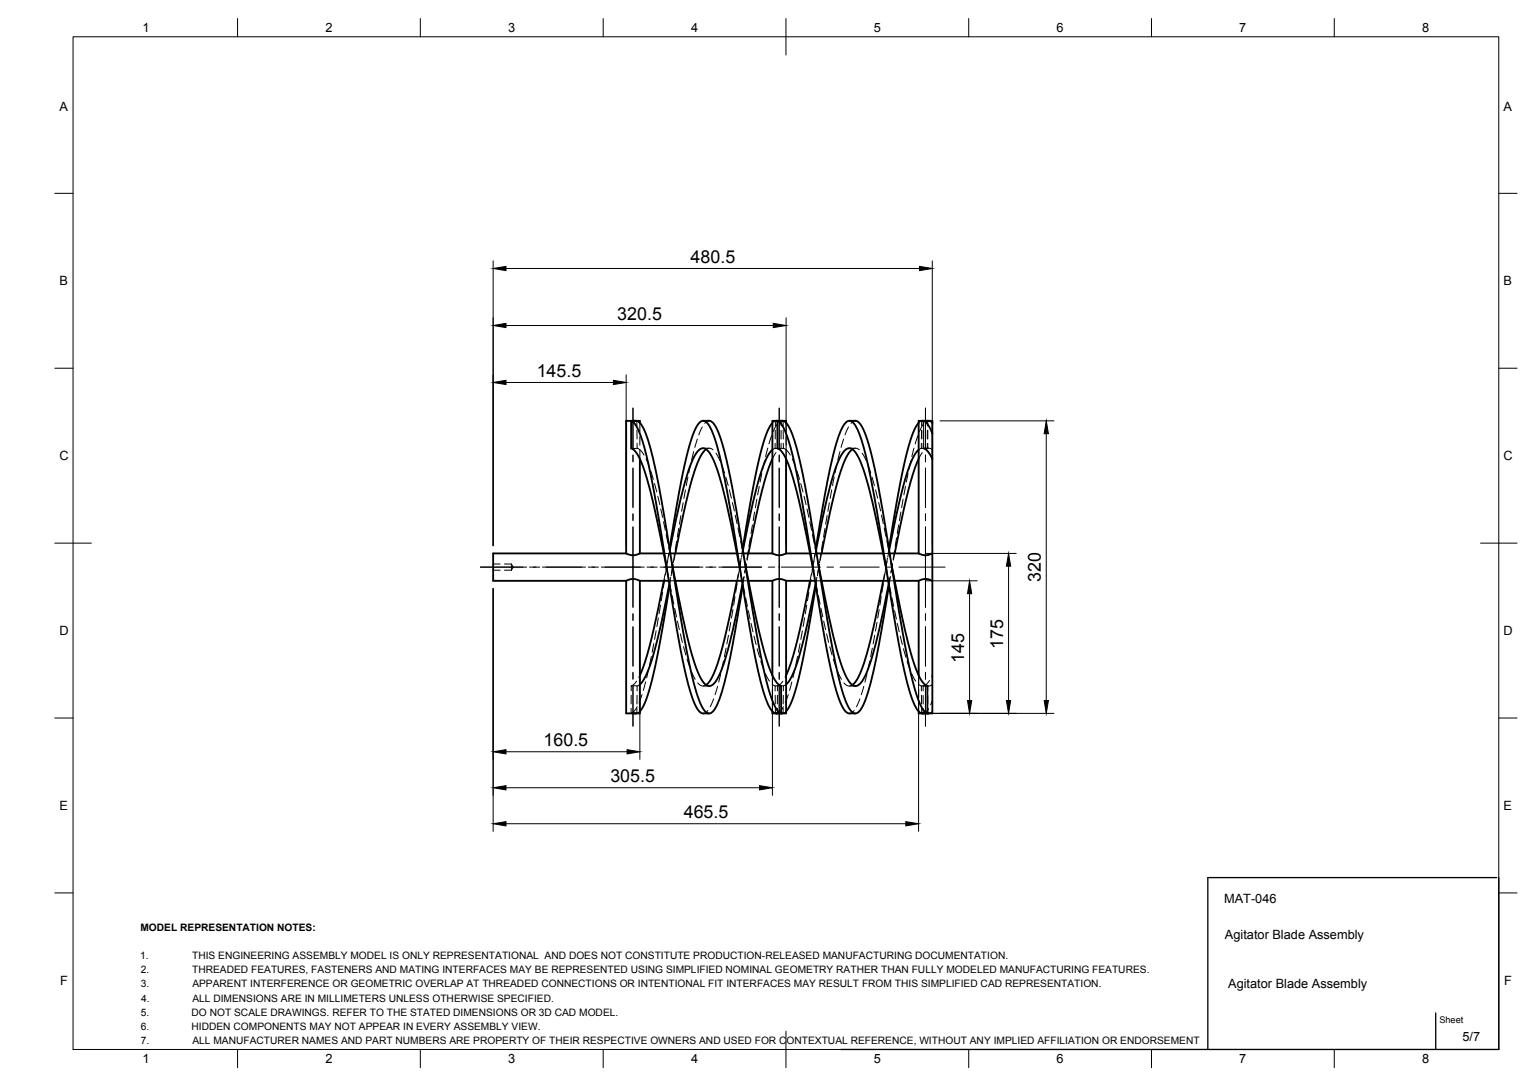
ISO-10303-21;
HEADER;
/* Generated by software containing ST-Developer
 * from STEP Tools, Inc. (www.steptools.com) 
 */

FILE_DESCRIPTION(
/* description */ ('STEP AP214'),
/* implementation_level */ '2;1');

FILE_NAME(
/* name */ 'Agitator Blade Assembly.step',
/* time_stamp */ '2026-11-14T22:16:48-08:00',
/* author */ (''),
/* organization */ (''),
/* preprocessor_version */ 'ST-DEVELOPER v20.2',
/* originating_system */ 'Autodesk Translation Framework v15.17.0.0',
/* authorisation */ '');

FILE_SCHEMA (('AUTOMOTIVE_DESIGN { 1 0 10303 214 3 1 1 }'));
ENDSEC;

DATA;
#10=MECHANICAL_DESIGN_GEOMETRIC_PRESENTATION_REPRESENTATION('',(#5496,#5497,#5498),#276462);
#335=CONICAL_SURFACE('',#110842,3.4,1.02974425867665);
#4017=(
BOUNDED_SURFACE()
B_SPLINE_SURFACE(1,2,((#265160,#265161,#265162,#265163,#265164,#265165,
#265166,#265167,#265168,#265169,#265170,#265171,#265172,#265173,#265174,
#265175,#265176,#265177,#265178,#265179,#265180,#265181,#265182,#265183,
#265184,#265185,#265186,#265187,#265188,#265189,#265190,#265191,#265192,
#265193,#265194,#265195,#265196,#265197,#265198,#265199,#265200,#265201,
#265202,#265203,#265204,#265205,#265206,#265207,#265208,#265209,#265210,
#265211,#265212,#265213,#265214,#265215,#265216,#265217,#265218,#265219,
#265220,#265221,#265222,#265223,#265224,#265225,#265226,#265227,#265228,
#265229,#265230,#265231,#265232,#265233,#265234,#265235,#265236,#265237,
#265238,#265239,#265240),(#265241,#265242,#265243,#265244,#265245,#265246,
#265247,#265248,#265249,#265250,#265251,#265252,#265253,#265254,#265255,
#265256,#265257,#265258,#265259,#265260,#265261,#265262,#265263,#265264,
#265265,#265266,#265267,#265268,#265269,#265270,#265271,#265272,#265273,
#265274,#265275,#265276,#265277,#265278,#265279,#265280,#265281,#265282,
#265283,#265284,#265285,#265286,#265287,#265288,#265289,#265290,#265291,
#265292,#265293,#265294,#265295,#265296,#265297,#265298,#265299,#265300,
#265301,#265302,#265303,#265304,#265305,#265306,#265307,#265308,#265309,
#265310,#265311,#265312,#265313,#265314,#265315,#265316,#265317,#265318,
#265319,#265320,#265321)),.UNSPECIFIED.,.F.,.F.,.F.)
B_SPLINE_SURFACE_WITH_KNOTS((2,2),(3,2,2,2,2,2,2,2,2,2,2,2,2,2,2,2,2,2,
2,2,2,2,2,2,2,2,2,2,2,2,2,2,2,2,2,2,2,2,2,2,3),(0.,1.),(0.,0.025,0.05,0.075,
0.1,0.125,0.15,0.175,0.2,0.225,0.25,0.275,0.3,0.325,0.35,0.375,0.4,0.425,
0.45,0.475,0.5,0.525,0.55,0.575,0.6,0.625,0.65,0.675,0.7,0.725,0.75,0.775,
0.8,0.825,0.85,0.875,0.9,0.925,0.95,0.975,1.),.UNSPECIFIED.)
GEOMETRIC_REPRESENTATION_ITEM()
RATIONAL_B_SPLINE_SURFACE(((1.,0.996917333733128,1.,0.996917333733128,1.,
0.996917333733128,1.,0.996917333733128,1.,0.996917333733128,1.,0.996917333733128,
1.,0.996917333733128,1.,0.996917333733128,1.,0.996917333733128,1.,0.996917333733128,
1.,0.996917333733128,1.,0.996917333733128,1.,0.996917333733128,1.,0.996917333733128,
1.,0.996917333733128,1.,0.996917333733128,1.,0.996917333733128,1.,0.996917333733128,
1.,0.996917333733128,1.,0.996917333733128,1.,0.996917333733128,1.,0.996917333733128,
1.,0.996917333733128,1.,0.996917333733128,1.,0.996917333733128,1.,0.996917333733128,
1.,0.996917333733128,1.,0.996917333733128,1.,0.996917333733128,1.,0.996917333733128,
1.,0.996917333733128,1.,0.996917333733128,1.,0.996917333733128,1.,0.996917333733128,
1.,0.996917333733128,1.,0.996917333733128,1.,0.996917333733128,1.,0.996917333733128,
1.,0.996917333733128,1.,0.996917333733128,1.),(1.,0.996917333733128,1.,
0.996917333733128,1.,0.996917333733128,1.,0.996917333733128,1.,0.996917333733128,
1.,0.996917333733128,1.,0.996917333733128,1.,0.996917333733128,1.,0.996917333733128,
1.,0.996917333733128,1.,0.996917333733128,1.,0.996917333733128,1.,0.996917333733128,
1.,0.996917333733128,1.,0.996917333733128,1.,0.996917333733128,1.,0.996917333733128,
1.,0.996917333733128,1.,0.996917333733128,1.,0.996917333733128,1.,0.996917333733128,
1.,0.996917333733128,1.,0.996917333733128,1.,0.996917333733128,1.,0.996917333733128,
1.,0.996917333733128,1.,0.996917333733128,1.,0.996917333733128,1.,0.996917333733128,
1.,0.996917333733128,1.,0.996917333733128,1.,0.996917333733128,1.,0.996917333733128,
1.,0.996917333733128,1.,0.996917333733128,1.,0.996917333733128,1.,0.996917333733128,
1.,0.996917333733128,1.,0.996917333733128,1.,0.996917333733128,1.)))
REPRESENTATION_ITEM('')
SURFACE()
);
#4018=(
BOUNDED_SURFACE()
B_SPLINE_SURFACE(1,2,((#265347,#265348,#265349,#265350,#265351,#265352,
#265353,#265354,#265355,#265356,#265357,#265358,#265359,#265360,#265361,
#265362,#265363,#265364,#265365,#265366,#265367,#265368,#265369,#265370,
#265371,#265372,#265373,#265374,#265375,#265376,#265377,#265378,#265379,
#265380,#265381,#265382,#265383,#265384,#265385,#265386,#265387,#265388,
#265389,#265390,#265391,#265392,#265393,#265394,#265395,#265396,#265397,
#265398,#265399,#265400,#265401,#265402,#265403,#265404,#265405,#265406,
#265407,#265408,#265409,#265410,#265411,#265412,#265413,#265414,#265415,
#265416,#265417,#265418,#265419,#265420,#265421,#265422,#265423,#265424,
#265425,#265426,#265427),(#265428,#265429,#265430,#265431,#265432,#265433,
#265434,#265435,#265436,#265437,#265438,#265439,#265440,#265441,#265442,
#265443,#265444,#265445,#265446,#265447,#265448,#265449,#265450,#265451,
#265452,#265453,#265454,#265455,#265456,#265457,#265458,#265459,#265460,
#265461,#265462,#265463,#265464,#265465,#265466,#265467,#265468,#265469,
#265470,#265471,#265472,#265473,#265474,#265475,#265476,#265477,#265478,
#265479,#265480,#265481,#265482,#265483,#265484,#265485,#265486,#265487,
#265488,#265489,#265490,#265491,#265492,#265493,#265494,#265495,#265496,
#265497,#265498,#265499,#265500,#265501,#265502,#265503,#265504,#265505,
#265506,#265507,#265508)),.UNSPECIFIED.,.F.,.F.,.F.)
B_SPLINE_SURFACE_WITH_KNOTS((2,2),(3,2,2,2,2,2,2,2,2,2,2,2,2,2,2,2,2,2,
2,2,2,2,2,2,2,2,2,2,2,2,2,2,2,2,2,2,2,2,2,2,3),(0.,1.),(0.,0.025,0.05,0.075,
0.1,0.125,0.15,0.175,0.2,0.225,0.25,0.275,0.3,0.325,0.35,0.375,0.4,0.425,
0.45,0.475,0.5,0.525,0.55,0.575,0.6,0.625,0.65,0.675,0.7,0.725,0.75,0.775,
0.8,0.825,0.85,0.875,0.9,0.925,0.95,0.975,1.),.UNSPECIFIED.)
GEOMETRIC_REPRESENTATION_ITEM()
RATIONAL_B_SPLINE_SURFACE(((1.,0.996917333733128,1.,0.996917333733128,1.,
0.996917333733128,1.,0.996917333733128,1.,0.996917333733128,1.,0.996917333733128,
1.,0.996917333733128,1.,0.996917333733128,1.,0.996917333733128,1.,0.996917333733128,
1.,0.996917333733128,1.,0.996917333733128,1.,0.996917333733128,1.,0.996917333733128,
1.,0.996917333733128,1.,0.996917333733128,1.,0.996917333733128,1.,0.996917333733128,
1.,0.996917333733128,1.,0.996917333733128,1.,0.996917333733128,1.,0.996917333733128,
1.,0.996917333733128,1.,0.996917333733128,1.,0.996917333733128,1.,0.996917333733128,
1.,0.996917333733128,1.,0.996917333733128,1.,0.996917333733128,1.,0.996917333733128,
1.,0.996917333733128,1.,0.996917333733128,1.,0.996917333733128,1.,0.996917333733128,
1.,0.996917333733128,1.,0.996917333733128,1.,0.996917333733128,1.,0.996917333733128,
1.,0.996917333733128,1.,0.996917333733128,1.),(1.,0.996917333733128,1.,
0.996917333733128,1.,0.996917333733128,1.,0.996917333733128,1.,0.996917333733128,
1.,0.996917333733128,1.,0.996917333733128,1.,0.996917333733128,1.,0.996917333733128,
1.,0.996917333733128,1.,0.996917333733128,1.,0.996917333733128,1.,0.996917333733128,
1.,0.996917333733128,1.,0.996917333733128,1.,0.996917333733128,1.,0.996917333733128,
1.,0.996917333733128,1.,0.996917333733128,1.,0.996917333733128,1.,0.996917333733128,
1.,0.996917333733128,1.,0.996917333733128,1.,0.996917333733128,1.,0.996917333733128,
1.,0.996917333733128,1.,0.996917333733128,1.,0.996917333733128,1.,0.996917333733128,
1.,0.996917333733128,1.,0.996917333733128,1.,0.996917333733128,1.,0.996917333733128,
1.,0.996917333733128,1.,0.996917333733128,1.,0.996917333733128,1.,0.996917333733128,
1.,0.996917333733128,1.,0.996917333733128,1.,0.996917333733128,1.)))
REPRESENTATION_ITEM('')
SURFACE()
);
#4019=(
BOUNDED_SURFACE()
B_SPLINE_SURFACE(1,2,((#265518,#265519,#265520,#265521,#265522,#265523,
#265524,#265525,#265526,#265527,#265528,#265529,#265530,#265531,#265532,
#265533,#265534,#265535,#265536,#265537,#265538,#265539,#265540,#265541,
#265542,#265543,#265544,#265545,#265546,#265547,#265548,#265549,#265550,
#265551,#265552,#265553,#265554,#265555,#265556,#265557,#265558,#265559,
#265560,#265561,#265562,#265563,#265564,#265565,#265566,#265567,#265568,
#265569,#265570,#265571,#265572,#265573,#265574,#265575,#265576,#265577,
#265578,#265579,#265580,#265581,#265582,#265583,#265584,#265585,#265586,
#265587,#265588,#265589,#265590,#265591,#265592,#265593,#265594,#265595,
#265596,#265597,#265598),(#265599,#265600,#265601,#265602,#265603,#265604,
#265605,#265606,#265607,#265608,#265609,#265610,#265611,#265612,#265613,
#265614,#265615,#265616,#265617,#265618,#265619,#265620,#265621,#265622,
#265623,#265624,#265625,#265626,#265627,#265628,#265629,#265630,#265631,
#265632,#265633,#265634,#265635,#265636,#265637,#265638,#265639,#265640,
#265641,#265642,#265643,#265644,#265645,#265646,#265647,#265648,#265649,
#265650,#265651,#265652,#265653,#265654,#265655,#265656,#265657,#265658,
#265659,#265660,#265661,#265662,#265663,#265664,#265665,#265666,#265667,
#265668,#265669,#265670,#265671,#265672,#265673,#265674,#265675,#265676,
#265677,#265678,#265679)),.UNSPECIFIED.,.F.,.F.,.F.)
B_SPLINE_SURFACE_WITH_KNOTS((2,2),(3,2,2,2,2,2,2,2,2,2,2,2,2,2,2,2,2,2,
2,2,2,2,2,2,2,2,2,2,2,2,2,2,2,2,2,2,2,2,2,2,3),(0.,1.),(0.,0.025,0.05,0.075,
0.1,0.125,0.15,0.175,0.2,0.225,0.25,0.275,0.3,0.325,0.35,0.375,0.4,0.425,
0.45,0.475,0.5,0.525,0.55,0.575,0.6,0.625,0.65,0.675,0.7,0.725,0.75,0.775,
0.8,0.825,0.85,0.875,0.9,0.925,0.95,0.975,1.),.UNSPECIFIED.)
GEOMETRIC_REPRESENTATION_ITEM()
RATIONAL_B_SPLINE_SURFACE(((1.,0.996917333733128,1.,0.996917333733128,1.,
0.996917333733128,1.,0.996917333733128,1.,0.996917333733128,1.,0.996917333733128,
1.,0.996917333733128,1.,0.996917333733128,1.,0.996917333733128,1.,0.996917333733128,
1.,0.996917333733128,1.,0.996917333733128,1.,0.996917333733128,1.,0.996917333733128,
1.,0.996917333733128,1.,0.996917333733128,1.,0.996917333733128,1.,0.996917333733128,
1.,0.996917333733128,1.,0.996917333733128,1.,0.996917333733128,1.,0.996917333733128,
1.,0.996917333733128,1.,0.996917333733128,1.,0.996917333733128,1.,0.996917333733128,
1.,0.996917333733128,1.,0.996917333733128,1.,0.996917333733128,1.,0.996917333733128,
1.,0.996917333733128,1.,0.996917333733128,1.,0.996917333733128,1.,0.996917333733128,
1.,0.996917333733128,1.,0.996917333733128,1.,0.996917333733128,1.,0.996917333733128,
1.,0.996917333733128,1.,0.996917333733128,1.),(1.,0.996917333733128,1.,
0.996917333733128,1.,0.996917333733128,1.,0.996917333733128,1.,0.996917333733128,
1.,0.996917333733128,1.,0.996917333733128,1.,0.996917333733128,1.,0.996917333733128,
1.,0.996917333733128,1.,0.996917333733128,1.,0.996917333733128,1.,0.996917333733128,
1.,0.996917333733128,1.,0.996917333733128,1.,0.996917333733128,1.,0.996917333733128,
1.,0.996917333733128,1.,0.996917333733128,1.,0.996917333733128,1.,0.996917333733128,
1.,0.996917333733128,1.,0.996917333733128,1.,0.996917333733128,1.,0.996917333733128,
1.,0.996917333733128,1.,0.996917333733128,1.,0.996917333733128,1.,0.996917333733128,
1.,0.996917333733128,1.,0.996917333733128,1.,0.996917333733128,1.,0.996917333733128,
1.,0.996917333733128,1.,0.996917333733128,1.,0.996917333733128,1.,0.996917333733128,
1.,0.996917333733128,1.,0.996917333733128,1.,0.996917333733128,1.)))
REPRESENTATION_ITEM('')
SURFACE()
);
#4020=(
BOUNDED_SURFACE()
B_SPLINE_SURFACE(1,2,((#265698,#265699,#265700,#265701,#265702,#265703,
#265704,#265705,#265706,#265707,#265708,#265709,#265710,#265711,#265712,
#265713,#265714,#265715,#265716,#265717,#265718,#265719,#265720,#265721,
#265722,#265723,#265724,#265725,#265726,#265727,#265728,#265729,#265730,
#265731,#265732,#265733,#265734,#265735,#265736,#265737,#265738,#265739,
#265740,#265741,#265742,#265743,#265744,#265745,#265746,#265747,#265748,
#265749,#265750,#265751,#265752,#265753,#265754,#265755,#265756,#265757,
#265758,#265759,#265760,#265761,#265762,#265763,#265764,#265765,#265766,
#265767,#265768,#265769,#265770,#265771,#265772,#265773,#265774,#265775,
#265776,#265777,#265778),(#265779,#265780,#265781,#265782,#265783,#265784,
#265785,#265786,#265787,#265788,#265789,#265790,#265791,#265792,#265793,
#265794,#265795,#265796,#265797,#265798,#265799,#265800,#265801,#265802,
#265803,#265804,#265805,#265806,#265807,#265808,#265809,#265810,#265811,
#265812,#265813,#265814,#265815,#265816,#265817,#265818,#265819,#265820,
#265821,#265822,#265823,#265824,#265825,#265826,#265827,#265828,#265829,
#265830,#265831,#265832,#265833,#265834,#265835,#265836,#265837,#265838,
#265839,#265840,#265841,#265842,#265843,#265844,#265845,#265846,#265847,
#265848,#265849,#265850,#265851,#265852,#265853,#265854,#265855,#265856,
#265857,#265858,#265859)),.UNSPECIFIED.,.F.,.F.,.F.)
B_SPLINE_SURFACE_WITH_KNOTS((2,2),(3,2,2,2,2,2,2,2,2,2,2,2,2,2,2,2,2,2,
2,2,2,2,2,2,2,2,2,2,2,2,2,2,2,2,2,2,2,2,2,2,3),(0.,1.),(0.,0.025,0.05,0.075,
0.1,0.125,0.15,0.175,0.2,0.225,0.25,0.275,0.3,0.325,0.35,0.375,0.4,0.425,
0.45,0.475,0.5,0.525,0.55,0.575,0.6,0.625,0.65,0.675,0.7,0.725,0.75,0.775,
0.8,0.825,0.85,0.875,0.9,0.925,0.95,0.975,1.),.UNSPECIFIED.)
GEOMETRIC_REPRESENTATION_ITEM()
RATIONAL_B_SPLINE_SURFACE(((1.,0.996917333733128,1.,0.996917333733128,1.,
0.996917333733128,1.,0.996917333733128,1.,0.996917333733128,1.,0.996917333733128,
1.,0.996917333733128,1.,0.996917333733128,1.,0.996917333733128,1.,0.996917333733128,
1.,0.996917333733128,1.,0.996917333733128,1.,0.996917333733128,1.,0.996917333733128,
1.,0.996917333733128,1.,0.996917333733128,1.,0.996917333733128,1.,0.996917333733128,
1.,0.996917333733128,1.,0.996917333733128,1.,0.996917333733128,1.,0.996917333733128,
1.,0.996917333733128,1.,0.996917333733128,1.,0.996917333733128,1.,0.996917333733128,
1.,0.996917333733128,1.,0.996917333733128,1.,0.996917333733128,1.,0.996917333733128,
1.,0.996917333733128,1.,0.996917333733128,1.,0.996917333733128,1.,0.996917333733128,
1.,0.996917333733128,1.,0.996917333733128,1.,0.996917333733128,1.,0.996917333733128,
1.,0.996917333733128,1.,0.996917333733128,1.),(1.,0.996917333733128,1.,
0.996917333733128,1.,0.996917333733128,1.,0.996917333733128,1.,0.996917333733128,
1.,0.996917333733128,1.,0.996917333733128,1.,0.996917333733128,1.,0.996917333733128,
1.,0.996917333733128,1.,0.996917333733128,1.,0.996917333733128,1.,0.996917333733128,
1.,0.996917333733128,1.,0.996917333733128,1.,0.996917333733128,1.,0.996917333733128,
1.,0.996917333733128,1.,0.996917333733128,1.,0.996917333733128,1.,0.996917333733128,
1.,0.996917333733128,1.,0.996917333733128,1.,0.996917333733128,1.,0.996917333733128,
1.,0.996917333733128,1.,0.996917333733128,1.,0.996917333733128,1.,0.996917333733128,
1.,0.996917333733128,1.,0.996917333733128,1.,0.996917333733128,1.,0.996917333733128,
1.,0.996917333733128,1.,0.996917333733128,1.,0.996917333733128,1.,0.996917333733128,
1.,0.996917333733128,1.,0.996917333733128,1.,0.996917333733128,1.)))
REPRESENTATION_ITEM('')
SURFACE()
);
#4021=(
BOUNDED_SURFACE()
B_SPLINE_SURFACE(1,2,((#265864,#265865,#265866,#265867,#265868,#265869,
#265870,#265871,#265872,#265873,#265874,#265875,#265876,#265877,#265878,
#265879,#265880,#265881,#265882,#265883,#265884,#265885,#265886,#265887,
#265888,#265889,#265890,#265891,#265892,#265893,#265894,#265895,#265896,
#265897,#265898,#265899,#265900,#265901,#265902,#265903,#265904,#265905,
#265906,#265907,#265908,#265909,#265910,#265911,#265912,#265913,#265914,
#265915,#265916,#265917,#265918,#265919,#265920,#265921,#265922,#265923,
#265924,#265925,#265926,#265927,#265928,#265929,#265930,#265931,#265932,
#265933,#265934,#265935,#265936,#265937,#265938,#265939,#265940,#265941,
#265942,#265943,#265944),(#265945,#265946,#265947,#265948,#265949,#265950,
#265951,#265952,#265953,#265954,#265955,#265956,#265957,#265958,#265959,
#265960,#265961,#265962,#265963,#265964,#265965,#265966,#265967,#265968,
#265969,#265970,#265971,#265972,#265973,#265974,#265975,#265976,#265977,
#265978,#265979,#265980,#265981,#265982,#265983,#265984,#265985,#265986,
#265987,#265988,#265989,#265990,#265991,#265992,#265993,#265994,#265995,
#265996,#265997,#265998,#265999,#266000,#266001,#266002,#266003,#266004,
#266005,#266006,#266007,#266008,#266009,#266010,#266011,#266012,#266013,
#266014,#266015,#266016,#266017,#266018,#266019,#266020,#266021,#266022,
#266023,#266024,#266025)),.UNSPECIFIED.,.F.,.F.,.F.)
B_SPLINE_SURFACE_WITH_KNOTS((2,2),(3,2,2,2,2,2,2,2,2,2,2,2,2,2,2,2,2,2,
2,2,2,2,2,2,2,2,2,2,2,2,2,2,2,2,2,2,2,2,2,2,3),(0.,1.),(0.,0.025,0.05,0.075,
0.1,0.125,0.15,0.175,0.2,0.225,0.25,0.275,0.3,0.325,0.35,0.375,0.4,0.425,
0.45,0.475,0.5,0.525,0.55,0.575,0.6,0.625,0.65,0.675,0.7,0.725,0.75,0.775,
0.8,0.825,0.85,0.875,0.9,0.925,0.95,0.975,1.),.UNSPECIFIED.)
GEOMETRIC_REPRESENTATION_ITEM()
RATIONAL_B_SPLINE_SURFACE(((1.,0.996917333733128,1.,0.996917333733128,1.,
0.996917333733128,1.,0.996917333733128,1.,0.996917333733128,1.,0.996917333733128,
1.,0.996917333733128,1.,0.996917333733128,1.,0.996917333733128,1.,0.996917333733128,
1.,0.996917333733128,1.,0.996917333733128,1.,0.996917333733128,1.,0.996917333733128,
1.,0.996917333733128,1.,0.996917333733128,1.,0.996917333733128,1.,0.996917333733128,
1.,0.996917333733128,1.,0.996917333733128,1.,0.996917333733128,1.,0.996917333733128,
1.,0.996917333733128,1.,0.996917333733128,1.,0.996917333733128,1.,0.996917333733128,
1.,0.996917333733128,1.,0.996917333733128,1.,0.996917333733128,1.,0.996917333733128,
1.,0.996917333733128,1.,0.996917333733128,1.,0.996917333733128,1.,0.996917333733128,
1.,0.996917333733128,1.,0.996917333733128,1.,0.996917333733128,1.,0.996917333733128,
1.,0.996917333733128,1.,0.996917333733128,1.),(1.,0.996917333733128,1.,
0.996917333733128,1.,0.996917333733128,1.,0.996917333733128,1.,0.996917333733128,
1.,0.996917333733128,1.,0.996917333733128,1.,0.996917333733128,1.,0.996917333733128,
1.,0.996917333733128,1.,0.996917333733128,1.,0.996917333733128,1.,0.996917333733128,
1.,0.996917333733128,1.,0.996917333733128,1.,0.996917333733128,1.,0.996917333733128,
1.,0.996917333733128,1.,0.996917333733128,1.,0.996917333733128,1.,0.996917333733128,
1.,0.996917333733128,1.,0.996917333733128,1.,0.996917333733128,1.,0.996917333733128,
1.,0.996917333733128,1.,0.996917333733128,1.,0.996917333733128,1.,0.996917333733128,
1.,0.996917333733128,1.,0.996917333733128,1.,0.996917333733128,1.,0.996917333733128,
1.,0.996917333733128,1.,0.996917333733128,1.,0.996917333733128,1.,0.996917333733128,
1.,0.996917333733128,1.,0.996917333733128,1.,0.996917333733128,1.)))
REPRESENTATION_ITEM('')
SURFACE()
);
#4022=(
BOUNDED_SURFACE()
B_SPLINE_SURFACE(1,2,((#266051,#266052,#266053,#266054,#266055,#266056,
#266057,#266058,#266059,#266060,#266061,#266062,#266063,#266064,#266065,
#266066,#266067,#266068,#266069,#266070,#266071,#266072,#266073,#266074,
#266075,#266076,#266077,#266078,#266079,#266080,#266081,#266082,#266083,
#266084,#266085,#266086,#266087,#266088,#266089,#266090,#266091,#266092,
#266093,#266094,#266095,#266096,#266097,#266098,#266099,#266100,#266101,
#266102,#266103,#266104,#266105,#266106,#266107,#266108,#266109,#266110,
#266111,#266112,#266113,#266114,#266115,#266116,#266117,#266118,#266119,
#266120,#266121,#266122,#266123,#266124,#266125,#266126,#266127,#266128,
#266129,#266130,#266131),(#266132,#266133,#266134,#266135,#266136,#266137,
#266138,#266139,#266140,#266141,#266142,#266143,#266144,#266145,#266146,
#266147,#266148,#266149,#266150,#266151,#266152,#266153,#266154,#266155,
#266156,#266157,#266158,#266159,#266160,#266161,#266162,#266163,#266164,
#266165,#266166,#266167,#266168,#266169,#266170,#266171,#266172,#266173,
#266174,#266175,#266176,#266177,#266178,#266179,#266180,#266181,#266182,
#266183,#266184,#266185,#266186,#266187,#266188,#266189,#266190,#266191,
#266192,#266193,#266194,#266195,#266196,#266197,#266198,#266199,#266200,
#266201,#266202,#266203,#266204,#266205,#266206,#266207,#266208,#266209,
#266210,#266211,#266212)),.UNSPECIFIED.,.F.,.F.,.F.)
B_SPLINE_SURFACE_WITH_KNOTS((2,2),(3,2,2,2,2,2,2,2,2,2,2,2,2,2,2,2,2,2,
2,2,2,2,2,2,2,2,2,2,2,2,2,2,2,2,2,2,2,2,2,2,3),(0.,1.),(0.,0.025,0.05,0.075,
0.1,0.125,0.15,0.175,0.2,0.225,0.25,0.275,0.3,0.325,0.35,0.375,0.4,0.425,
0.45,0.475,0.5,0.525,0.55,0.575,0.6,0.625,0.65,0.675,0.7,0.725,0.75,0.775,
0.8,0.825,0.85,0.875,0.9,0.925,0.95,0.975,1.),.UNSPECIFIED.)
GEOMETRIC_REPRESENTATION_ITEM()
RATIONAL_B_SPLINE_SURFACE(((1.,0.996917333733128,1.,0.996917333733128,1.,
0.996917333733128,1.,0.996917333733128,1.,0.996917333733128,1.,0.996917333733128,
1.,0.996917333733128,1.,0.996917333733128,1.,0.996917333733128,1.,0.996917333733128,
1.,0.996917333733128,1.,0.996917333733128,1.,0.996917333733128,1.,0.996917333733128,
1.,0.996917333733128,1.,0.996917333733128,1.,0.996917333733128,1.,0.996917333733128,
1.,0.996917333733128,1.,0.996917333733128,1.,0.996917333733128,1.,0.996917333733128,
1.,0.996917333733128,1.,0.996917333733128,1.,0.996917333733128,1.,0.996917333733128,
1.,0.996917333733128,1.,0.996917333733128,1.,0.996917333733128,1.,0.996917333733128,
1.,0.996917333733128,1.,0.996917333733128,1.,0.996917333733128,1.,0.996917333733128,
1.,0.996917333733128,1.,0.996917333733128,1.,0.996917333733128,1.,0.996917333733128,
1.,0.996917333733128,1.,0.996917333733128,1.),(1.,0.996917333733128,1.,
0.996917333733128,1.,0.996917333733128,1.,0.996917333733128,1.,0.996917333733128,
1.,0.996917333733128,1.,0.996917333733128,1.,0.996917333733128,1.,0.996917333733128,
1.,0.996917333733128,1.,0.996917333733128,1.,0.996917333733128,1.,0.996917333733128,
1.,0.996917333733128,1.,0.996917333733128,1.,0.996917333733128,1.,0.996917333733128,
1.,0.996917333733128,1.,0.996917333733128,1.,0.996917333733128,1.,0.996917333733128,
1.,0.996917333733128,1.,0.996917333733128,1.,0.996917333733128,1.,0.996917333733128,
1.,0.996917333733128,1.,0.996917333733128,1.,0.996917333733128,1.,0.996917333733128,
1.,0.996917333733128,1.,0.996917333733128,1.,0.996917333733128,1.,0.996917333733128,
1.,0.996917333733128,1.,0.996917333733128,1.,0.996917333733128,1.,0.996917333733128,
1.,0.996917333733128,1.,0.996917333733128,1.,0.996917333733128,1.)))
REPRESENTATION_ITEM('')
SURFACE()
);
#4023=(
BOUNDED_SURFACE()
B_SPLINE_SURFACE(1,2,((#266224,#266225,#266226,#266227,#266228,#266229,
#266230,#266231,#266232,#266233,#266234,#266235,#266236,#266237,#266238,
#266239,#266240,#266241,#266242,#266243,#266244,#266245,#266246,#266247,
#266248,#266249,#266250,#266251,#266252,#266253,#266254,#266255,#266256,
#266257,#266258,#266259,#266260,#266261,#266262,#266263,#266264,#266265,
#266266,#266267,#266268,#266269,#266270,#266271,#266272,#266273,#266274,
#266275,#266276,#266277,#266278,#266279,#266280,#266281,#266282,#266283,
#266284,#266285,#266286,#266287,#266288,#266289,#266290,#266291,#266292,
#266293,#266294,#266295,#266296,#266297,#266298,#266299,#266300,#266301,
#266302,#266303,#266304),(#266305,#266306,#266307,#266308,#266309,#266310,
#266311,#266312,#266313,#266314,#266315,#266316,#266317,#266318,#266319,
#266320,#266321,#266322,#266323,#266324,#266325,#266326,#266327,#266328,
#266329,#266330,#266331,#266332,#266333,#266334,#266335,#266336,#266337,
#266338,#266339,#266340,#266341,#266342,#266343,#266344,#266345,#266346,
#266347,#266348,#266349,#266350,#266351,#266352,#266353,#266354,#266355,
#266356,#266357,#266358,#266359,#266360,#266361,#266362,#266363,#266364,
#266365,#266366,#266367,#266368,#266369,#266370,#266371,#266372,#266373,
#266374,#266375,#266376,#266377,#266378,#266379,#266380,#266381,#266382,
#266383,#266384,#266385)),.UNSPECIFIED.,.F.,.F.,.F.)
B_SPLINE_SURFACE_WITH_KNOTS((2,2),(3,2,2,2,2,2,2,2,2,2,2,2,2,2,2,2,2,2,
2,2,2,2,2,2,2,2,2,2,2,2,2,2,2,2,2,2,2,2,2,2,3),(0.,1.),(0.,0.025,0.05,0.075,
0.1,0.125,0.15,0.175,0.2,0.225,0.25,0.275,0.3,0.325,0.35,0.375,0.4,0.425,
0.45,0.475,0.5,0.525,0.55,0.575,0.6,0.625,0.65,0.675,0.7,0.725,0.75,0.775,
0.8,0.825,0.85,0.875,0.9,0.925,0.95,0.975,1.),.UNSPECIFIED.)
GEOMETRIC_REPRESENTATION_ITEM()
RATIONAL_B_SPLINE_SURFACE(((1.,0.996917333733128,1.,0.996917333733128,1.,
0.996917333733128,1.,0.996917333733128,1.,0.996917333733128,1.,0.996917333733128,
1.,0.996917333733128,1.,0.996917333733128,1.,0.996917333733128,1.,0.996917333733128,
1.,0.996917333733128,1.,0.996917333733128,1.,0.996917333733128,1.,0.996917333733128,
1.,0.996917333733128,1.,0.996917333733128,1.,0.996917333733128,1.,0.996917333733128,
1.,0.996917333733128,1.,0.996917333733128,1.,0.996917333733128,1.,0.996917333733128,
1.,0.996917333733128,1.,0.996917333733128,1.,0.996917333733128,1.,0.996917333733128,
1.,0.996917333733128,1.,0.996917333733128,1.,0.996917333733128,1.,0.996917333733128,
1.,0.996917333733128,1.,0.996917333733128,1.,0.996917333733128,1.,0.996917333733128,
1.,0.996917333733128,1.,0.996917333733128,1.,0.996917333733128,1.,0.996917333733128,
1.,0.996917333733128,1.,0.996917333733128,1.),(1.,0.996917333733128,1.,
0.996917333733128,1.,0.996917333733128,1.,0.996917333733128,1.,0.996917333733128,
1.,0.996917333733128,1.,0.996917333733128,1.,0.996917333733128,1.,0.996917333733128,
1.,0.996917333733128,1.,0.996917333733128,1.,0.996917333733128,1.,0.996917333733128,
1.,0.996917333733128,1.,0.996917333733128,1.,0.996917333733128,1.,0.996917333733128,
1.,0.996917333733128,1.,0.996917333733128,1.,0.996917333733128,1.,0.996917333733128,
1.,0.996917333733128,1.,0.996917333733128,1.,0.996917333733128,1.,0.996917333733128,
1.,0.996917333733128,1.,0.996917333733128,1.,0.996917333733128,1.,0.996917333733128,
1.,0.996917333733128,1.,0.996917333733128,1.,0.996917333733128,1.,0.996917333733128,
1.,0.996917333733128,1.,0.996917333733128,1.,0.996917333733128,1.,0.996917333733128,
1.,0.996917333733128,1.,0.996917333733128,1.,0.996917333733128,1.)))
REPRESENTATION_ITEM('')
SURFACE()
);
#4024=(
BOUNDED_SURFACE()
B_SPLINE_SURFACE(1,2,((#266402,#266403,#266404,#266405,#266406,#266407,
#266408,#266409,#266410,#266411,#266412,#266413,#266414,#266415,#266416,
#266417,#266418,#266419,#266420,#266421,#266422,#266423,#266424,#266425,
#266426,#266427,#266428,#266429,#266430,#266431,#266432,#266433,#266434,
#266435,#266436,#266437,#266438,#266439,#266440,#266441,#266442,#266443,
#266444,#266445,#266446,#266447,#266448,#266449,#266450,#266451,#266452,
#266453,#266454,#266455,#266456,#266457,#266458,#266459,#266460,#266461,
#266462,#266463,#266464,#266465,#266466,#266467,#266468,#266469,#266470,
#266471,#266472,#266473,#266474,#266475,#266476,#266477,#266478,#266479,
#266480,#266481,#266482),(#266483,#266484,#266485,#266486,#266487,#266488,
#266489,#266490,#266491,#266492,#266493,#266494,#266495,#266496,#266497,
#266498,#266499,#266500,#266501,#266502,#266503,#266504,#266505,#266506,
#266507,#266508,#266509,#266510,#266511,#266512,#266513,#266514,#266515,
#266516,#266517,#266518,#266519,#266520,#266521,#266522,#266523,#266524,
#266525,#266526,#266527,#266528,#266529,#266530,#266531,#266532,#266533,
#266534,#266535,#266536,#266537,#266538,#266539,#266540,#266541,#266542,
#266543,#266544,#266545,#266546,#266547,#266548,#266549,#266550,#266551,
#266552,#266553,#266554,#266555,#266556,#266557,#266558,#266559,#266560,
#266561,#266562,#266563)),.UNSPECIFIED.,.F.,.F.,.F.)
B_SPLINE_SURFACE_WITH_KNOTS((2,2),(3,2,2,2,2,2,2,2,2,2,2,2,2,2,2,2,2,2,
2,2,2,2,2,2,2,2,2,2,2,2,2,2,2,2,2,2,2,2,2,2,3),(0.,1.),(0.,0.025,0.05,0.075,
0.1,0.125,0.15,0.175,0.2,0.225,0.25,0.275,0.3,0.325,0.35,0.375,0.4,0.425,
0.45,0.475,0.5,0.525,0.55,0.575,0.6,0.625,0.65,0.675,0.7,0.725,0.75,0.775,
0.8,0.825,0.85,0.875,0.9,0.925,0.95,0.975,1.),.UNSPECIFIED.)
GEOMETRIC_REPRESENTATION_ITEM()
RATIONAL_B_SPLINE_SURFACE(((1.,0.996917333733128,1.,0.996917333733128,1.,
0.996917333733128,1.,0.996917333733128,1.,0.996917333733128,1.,0.996917333733128,
1.,0.996917333733128,1.,0.996917333733128,1.,0.996917333733128,1.,0.996917333733128,
1.,0.996917333733128,1.,0.996917333733128,1.,0.996917333733128,1.,0.996917333733128,
1.,0.996917333733128,1.,0.996917333733128,1.,0.996917333733128,1.,0.996917333733128,
1.,0.996917333733128,1.,0.996917333733128,1.,0.996917333733128,1.,0.996917333733128,
1.,0.996917333733128,1.,0.996917333733128,1.,0.996917333733128,1.,0.996917333733128,
1.,0.996917333733128,1.,0.996917333733128,1.,0.996917333733128,1.,0.996917333733128,
1.,0.996917333733128,1.,0.996917333733128,1.,0.996917333733128,1.,0.996917333733128,
1.,0.996917333733128,1.,0.996917333733128,1.,0.996917333733128,1.,0.996917333733128,
1.,0.996917333733128,1.,0.996917333733128,1.),(1.,0.996917333733128,1.,
0.996917333733128,1.,0.996917333733128,1.,0.996917333733128,1.,0.996917333733128,
1.,0.996917333733128,1.,0.996917333733128,1.,0.996917333733128,1.,0.996917333733128,
1.,0.996917333733128,1.,0.996917333733128,1.,0.996917333733128,1.,0.996917333733128,
1.,0.996917333733128,1.,0.996917333733128,1.,0.996917333733128,1.,0.996917333733128,
1.,0.996917333733128,1.,0.996917333733128,1.,0.996917333733128,1.,0.996917333733128,
1.,0.996917333733128,1.,0.996917333733128,1.,0.996917333733128,1.,0.996917333733128,
1.,0.996917333733128,1.,0.996917333733128,1.,0.996917333733128,1.,0.996917333733128,
1.,0.996917333733128,1.,0.996917333733128,1.,0.996917333733128,1.,0.996917333733128,
1.,0.996917333733128,1.,0.996917333733128,1.,0.996917333733128,1.,0.996917333733128,
1.,0.996917333733128,1.,0.996917333733128,1.,0.996917333733128,1.)))
REPRESENTATION_ITEM('')
SURFACE()
);
#4025=(
BOUNDED_SURFACE()
B_SPLINE_SURFACE(1,2,((#267127,#267128,#267129,#267130,#267131,#267132,
#267133,#267134,#267135,#267136,#267137,#267138,#267139,#267140,#267141,
#267142,#267143,#267144,#267145,#267146,#267147,#267148,#267149,#267150,
#267151,#267152,#267153,#267154,#267155,#267156,#267157,#267158,#267159,
#267160,#267161,#267162,#267163,#267164,#267165,#267166,#267167,#267168,
#267169,#267170,#267171,#267172,#267173,#267174,#267175,#267176,#267177,
#267178,#267179,#267180,#267181,#267182,#267183,#267184,#267185,#267186,
#267187,#267188,#267189,#267190,#267191,#267192,#267193,#267194,#267195,
#267196,#267197,#267198,#267199,#267200,#267201,#267202,#267203,#267204,
#267205,#267206,#267207),(#267208,#267209,#267210,#267211,#267212,#267213,
#267214,#267215,#267216,#267217,#267218,#267219,#267220,#267221,#267222,
#267223,#267224,#267225,#267226,#267227,#267228,#267229,#267230,#267231,
#267232,#267233,#267234,#267235,#267236,#267237,#267238,#267239,#267240,
#267241,#267242,#267243,#267244,#267245,#267246,#267247,#267248,#267249,
#267250,#267251,#267252,#267253,#267254,#267255,#267256,#267257,#267258,
#267259,#267260,#267261,#267262,#267263,#267264,#267265,#267266,#267267,
#267268,#267269,#267270,#267271,#267272,#267273,#267274,#267275,#267276,
#267277,#267278,#267279,#267280,#267281,#267282,#267283,#267284,#267285,
#267286,#267287,#267288)),.UNSPECIFIED.,.F.,.F.,.F.)
B_SPLINE_SURFACE_WITH_KNOTS((2,2),(3,2,2,2,2,2,2,2,2,2,2,2,2,2,2,2,2,2,
2,2,2,2,2,2,2,2,2,2,2,2,2,2,2,2,2,2,2,2,2,2,3),(0.,1.),(0.,0.025,0.05,0.075,
0.1,0.125,0.15,0.175,0.2,0.225,0.25,0.275,0.3,0.325,0.35,0.375,0.4,0.425,
0.45,0.475,0.5,0.525,0.55,0.575,0.6,0.625,0.65,0.675,0.7,0.725,0.75,0.775,
0.8,0.825,0.85,0.875,0.9,0.925,0.95,0.975,1.),.UNSPECIFIED.)
GEOMETRIC_REPRESENTATION_ITEM()
RATIONAL_B_SPLINE_SURFACE(((1.,0.996917333733128,1.,0.996917333733128,1.,
0.996917333733128,1.,0.996917333733128,1.,0.996917333733128,1.,0.996917333733128,
1.,0.996917333733128,1.,0.996917333733128,1.,0.996917333733128,1.,0.996917333733128,
1.,0.996917333733128,1.,0.996917333733128,1.,0.996917333733128,1.,0.996917333733128,
1.,0.996917333733128,1.,0.996917333733128,1.,0.996917333733128,1.,0.996917333733128,
1.,0.996917333733128,1.,0.996917333733128,1.,0.996917333733128,1.,0.996917333733128,
1.,0.996917333733128,1.,0.996917333733128,1.,0.996917333733128,1.,0.996917333733128,
1.,0.996917333733128,1.,0.996917333733128,1.,0.996917333733128,1.,0.996917333733128,
1.,0.996917333733128,1.,0.996917333733128,1.,0.996917333733128,1.,0.996917333733128,
1.,0.996917333733128,1.,0.996917333733128,1.,0.996917333733128,1.,0.996917333733128,
1.,0.996917333733128,1.,0.996917333733128,1.),(1.,0.996917333733128,1.,
0.996917333733128,1.,0.996917333733128,1.,0.996917333733128,1.,0.996917333733128,
1.,0.996917333733128,1.,0.996917333733128,1.,0.996917333733128,1.,0.996917333733128,
1.,0.996917333733128,1.,0.996917333733128,1.,0.996917333733128,1.,0.996917333733128,
1.,0.996917333733128,1.,0.996917333733128,1.,0.996917333733128,1.,0.996917333733128,
1.,0.996917333733128,1.,0.996917333733128,1.,0.996917333733128,1.,0.996917333733128,
1.,0.996917333733128,1.,0.996917333733128,1.,0.996917333733128,1.,0.996917333733128,
1.,0.996917333733128,1.,0.996917333733128,1.,0.996917333733128,1.,0.996917333733128,
1.,0.996917333733128,1.,0.996917333733128,1.,0.996917333733128,1.,0.996917333733128,
1.,0.996917333733128,1.,0.996917333733128,1.,0.996917333733128,1.,0.996917333733128,
1.,0.996917333733128,1.,0.996917333733128,1.,0.996917333733128,1.)))
REPRESENTATION_ITEM('')
SURFACE()
);
#4026=(
BOUNDED_SURFACE()
B_SPLINE_SURFACE(1,2,((#267451,#267452,#267453,#267454,#267455,#267456,
#267457,#267458,#267459,#267460,#267461,#267462,#267463,#267464,#267465,
#267466,#267467,#267468,#267469,#267470,#267471,#267472,#267473,#267474,
#267475,#267476,#267477,#267478,#267479,#267480,#267481,#267482,#267483,
#267484,#267485,#267486,#267487,#267488,#267489,#267490,#267491,#267492,
#267493,#267494,#267495,#267496,#267497,#267498,#267499,#267500,#267501,
#267502,#267503,#267504,#267505,#267506,#267507,#267508,#267509,#267510,
#267511,#267512,#267513,#267514,#267515,#267516,#267517,#267518,#267519,
#267520,#267521,#267522,#267523,#267524,#267525,#267526,#267527,#267528,
#267529,#267530,#267531),(#267532,#267533,#267534,#267535,#267536,#267537,
#267538,#267539,#267540,#267541,#267542,#267543,#267544,#267545,#267546,
#267547,#267548,#267549,#267550,#267551,#267552,#267553,#267554,#267555,
#267556,#267557,#267558,#267559,#267560,#267561,#267562,#267563,#267564,
#267565,#267566,#267567,#267568,#267569,#267570,#267571,#267572,#267573,
#267574,#267575,#267576,#267577,#267578,#267579,#267580,#267581,#267582,
#267583,#267584,#267585,#267586,#267587,#267588,#267589,#267590,#267591,
#267592,#267593,#267594,#267595,#267596,#267597,#267598,#267599,#267600,
#267601,#267602,#267603,#267604,#267605,#267606,#267607,#267608,#267609,
#267610,#267611,#267612)),.UNSPECIFIED.,.F.,.F.,.F.)
B_SPLINE_SURFACE_WITH_KNOTS((2,2),(3,2,2,2,2,2,2,2,2,2,2,2,2,2,2,2,2,2,
2,2,2,2,2,2,2,2,2,2,2,2,2,2,2,2,2,2,2,2,2,2,3),(0.,1.),(0.,0.025,0.05,0.075,
0.1,0.125,0.15,0.175,0.2,0.225,0.25,0.275,0.3,0.325,0.35,0.375,0.4,0.425,
0.45,0.475,0.5,0.525,0.55,0.575,0.6,0.625,0.65,0.675,0.7,0.725,0.75,0.775,
0.8,0.825,0.85,0.875,0.9,0.925,0.95,0.975,1.),.UNSPECIFIED.)
GEOMETRIC_REPRESENTATION_ITEM()
RATIONAL_B_SPLINE_SURFACE(((1.,0.996917333733128,1.,0.996917333733128,1.,
0.996917333733128,1.,0.996917333733128,1.,0.996917333733128,1.,0.996917333733128,
1.,0.996917333733128,1.,0.996917333733128,1.,0.996917333733128,1.,0.996917333733128,
1.,0.996917333733128,1.,0.996917333733128,1.,0.996917333733128,1.,0.996917333733128,
1.,0.996917333733128,1.,0.996917333733128,1.,0.996917333733128,1.,0.996917333733128,
1.,0.996917333733128,1.,0.996917333733128,1.,0.996917333733128,1.,0.996917333733128,
1.,0.996917333733128,1.,0.996917333733128,1.,0.996917333733128,1.,0.996917333733128,
1.,0.996917333733128,1.,0.996917333733128,1.,0.996917333733128,1.,0.996917333733128,
1.,0.996917333733128,1.,0.996917333733128,1.,0.996917333733128,1.,0.996917333733128,
1.,0.996917333733128,1.,0.996917333733128,1.,0.996917333733128,1.,0.996917333733128,
1.,0.996917333733128,1.,0.996917333733128,1.),(1.,0.996917333733128,1.,
0.996917333733128,1.,0.996917333733128,1.,0.996917333733128,1.,0.996917333733128,
1.,0.996917333733128,1.,0.996917333733128,1.,0.996917333733128,1.,0.996917333733128,
1.,0.996917333733128,1.,0.996917333733128,1.,0.996917333733128,1.,0.996917333733128,
1.,0.996917333733128,1.,0.996917333733128,1.,0.996917333733128,1.,0.996917333733128,
1.,0.996917333733128,1.,0.996917333733128,1.,0.996917333733128,1.,0.996917333733128,
1.,0.996917333733128,1.,0.996917333733128,1.,0.996917333733128,1.,0.996917333733128,
1.,0.996917333733128,1.,0.996917333733128,1.,0.996917333733128,1.,0.996917333733128,
1.,0.996917333733128,1.,0.996917333733128,1.,0.996917333733128,1.,0.996917333733128,
1.,0.996917333733128,1.,0.996917333733128,1.,0.996917333733128,1.,0.996917333733128,
1.,0.996917333733128,1.,0.996917333733128,1.,0.996917333733128,1.)))
REPRESENTATION_ITEM('')
SURFACE()
);
#4027=(
BOUNDED_SURFACE()
B_SPLINE_SURFACE(1,2,((#267694,#267695,#267696,#267697,#267698,#267699,
#267700,#267701,#267702,#267703,#267704,#267705,#267706,#267707,#267708,
#267709,#267710,#267711,#267712,#267713,#267714,#267715,#267716,#267717,
#267718,#267719,#267720,#267721,#267722,#267723,#267724,#267725,#267726,
#267727,#267728,#267729,#267730,#267731,#267732,#267733,#267734,#267735,
#267736,#267737,#267738,#267739,#267740,#267741,#267742,#267743,#267744,
#267745,#267746,#267747,#267748,#267749,#267750,#267751,#267752,#267753,
#267754,#267755,#267756,#267757,#267758,#267759,#267760,#267761,#267762,
#267763,#267764,#267765,#267766,#267767,#267768,#267769,#267770,#267771,
#267772,#267773,#267774),(#267775,#267776,#267777,#267778,#267779,#267780,
#267781,#267782,#267783,#267784,#267785,#267786,#267787,#267788,#267789,
#267790,#267791,#267792,#267793,#267794,#267795,#267796,#267797,#267798,
#267799,#267800,#267801,#267802,#267803,#267804,#267805,#267806,#267807,
#267808,#267809,#267810,#267811,#267812,#267813,#267814,#267815,#267816,
#267817,#267818,#267819,#267820,#267821,#267822,#267823,#267824,#267825,
#267826,#267827,#267828,#267829,#267830,#267831,#267832,#267833,#267834,
#267835,#267836,#267837,#267838,#267839,#267840,#267841,#267842,#267843,
#267844,#267845,#267846,#267847,#267848,#267849,#267850,#267851,#267852,
#267853,#267854,#267855)),.UNSPECIFIED.,.F.,.F.,.F.)
B_SPLINE_SURFACE_WITH_KNOTS((2,2),(3,2,2,2,2,2,2,2,2,2,2,2,2,2,2,2,2,2,
2,2,2,2,2,2,2,2,2,2,2,2,2,2,2,2,2,2,2,2,2,2,3),(0.,1.),(0.,0.025,0.05,0.075,
0.1,0.125,0.15,0.175,0.2,0.225,0.25,0.275,0.3,0.325,0.35,0.375,0.4,0.425,
0.45,0.475,0.5,0.525,0.55,0.575,0.6,0.625,0.65,0.675,0.7,0.725,0.75,0.775,
0.8,0.825,0.85,0.875,0.9,0.925,0.95,0.975,1.),.UNSPECIFIED.)
GEOMETRIC_REPRESENTATION_ITEM()
RATIONAL_B_SPLINE_SURFACE(((1.,0.996917333733128,1.,0.996917333733128,1.,
0.996917333733128,1.,0.996917333733128,1.,0.996917333733128,1.,0.996917333733128,
1.,0.996917333733128,1.,0.996917333733128,1.,0.996917333733128,1.,0.996917333733128,
1.,0.996917333733128,1.,0.996917333733128,1.,0.996917333733128,1.,0.996917333733128,
1.,0.996917333733128,1.,0.996917333733128,1.,0.996917333733128,1.,0.996917333733128,
1.,0.996917333733128,1.,0.996917333733128,1.,0.996917333733128,1.,0.996917333733128,
1.,0.996917333733128,1.,0.996917333733128,1.,0.996917333733128,1.,0.996917333733128,
1.,0.996917333733128,1.,0.996917333733128,1.,0.996917333733128,1.,0.996917333733128,
1.,0.996917333733128,1.,0.996917333733128,1.,0.996917333733128,1.,0.996917333733128,
1.,0.996917333733128,1.,0.996917333733128,1.,0.996917333733128,1.,0.996917333733128,
1.,0.996917333733128,1.,0.996917333733128,1.),(1.,0.996917333733128,1.,
0.996917333733128,1.,0.996917333733128,1.,0.996917333733128,1.,0.996917333733128,
1.,0.996917333733128,1.,0.996917333733128,1.,0.996917333733128,1.,0.996917333733128,
1.,0.996917333733128,1.,0.996917333733128,1.,0.996917333733128,1.,0.996917333733128,
1.,0.996917333733128,1.,0.996917333733128,1.,0.996917333733128,1.,0.996917333733128,
1.,0.996917333733128,1.,0.996917333733128,1.,0.996917333733128,1.,0.996917333733128,
1.,0.996917333733128,1.,0.996917333733128,1.,0.996917333733128,1.,0.996917333733128,
1.,0.996917333733128,1.,0.996917333733128,1.,0.996917333733128,1.,0.996917333733128,
1.,0.996917333733128,1.,0.996917333733128,1.,0.996917333733128,1.,0.996917333733128,
1.,0.996917333733128,1.,0.996917333733128,1.,0.996917333733128,1.,0.996917333733128,
1.,0.996917333733128,1.,0.996917333733128,1.,0.996917333733128,1.)))
REPRESENTATION_ITEM('')
SURFACE()
);
#4028=(
BOUNDED_SURFACE()
B_SPLINE_SURFACE(1,2,((#267937,#267938,#267939,#267940,#267941,#267942,
#267943,#267944,#267945,#267946,#267947,#267948,#267949,#267950,#267951,
#267952,#267953,#267954,#267955,#267956,#267957,#267958,#267959,#267960,
#267961,#267962,#267963,#267964,#267965,#267966,#267967,#267968,#267969,
#267970,#267971,#267972,#267973,#267974,#267975,#267976,#267977,#267978,
#267979,#267980,#267981,#267982,#267983,#267984,#267985,#267986,#267987,
#267988,#267989,#267990,#267991,#267992,#267993,#267994,#267995,#267996,
#267997,#267998,#267999,#268000,#268001,#268002,#268003,#268004,#268005,
#268006,#268007,#268008,#268009,#268010,#268011,#268012,#268013,#268014,
#268015,#268016,#268017),(#268018,#268019,#268020,#268021,#268022,#268023,
#268024,#268025,#268026,#268027,#268028,#268029,#268030,#268031,#268032,
#268033,#268034,#268035,#268036,#268037,#268038,#268039,#268040,#268041,
#268042,#268043,#268044,#268045,#268046,#268047,#268048,#268049,#268050,
#268051,#268052,#268053,#268054,#268055,#268056,#268057,#268058,#268059,
#268060,#268061,#268062,#268063,#268064,#268065,#268066,#268067,#268068,
#268069,#268070,#268071,#268072,#268073,#268074,#268075,#268076,#268077,
#268078,#268079,#268080,#268081,#268082,#268083,#268084,#268085,#268086,
#268087,#268088,#268089,#268090,#268091,#268092,#268093,#268094,#268095,
#268096,#268097,#268098)),.UNSPECIFIED.,.F.,.F.,.F.)
B_SPLINE_SURFACE_WITH_KNOTS((2,2),(3,2,2,2,2,2,2,2,2,2,2,2,2,2,2,2,2,2,
2,2,2,2,2,2,2,2,2,2,2,2,2,2,2,2,2,2,2,2,2,2,3),(0.,1.),(0.,0.025,0.05,0.075,
0.1,0.125,0.15,0.175,0.2,0.225,0.25,0.275,0.3,0.325,0.35,0.375,0.4,0.425,
0.45,0.475,0.5,0.525,0.55,0.575,0.6,0.625,0.65,0.675,0.7,0.725,0.75,0.775,
0.8,0.825,0.85,0.875,0.9,0.925,0.95,0.975,1.),.UNSPECIFIED.)
GEOMETRIC_REPRESENTATION_ITEM()
RATIONAL_B_SPLINE_SURFACE(((1.,0.996917333733128,1.,0.996917333733128,1.,
0.996917333733128,1.,0.996917333733128,1.,0.996917333733128,1.,0.996917333733128,
1.,0.996917333733128,1.,0.996917333733128,1.,0.996917333733128,1.,0.996917333733128,
1.,0.996917333733128,1.,0.996917333733128,1.,0.996917333733128,1.,0.996917333733128,
1.,0.996917333733128,1.,0.996917333733128,1.,0.996917333733128,1.,0.996917333733128,
1.,0.996917333733128,1.,0.996917333733128,1.,0.996917333733128,1.,0.996917333733128,
1.,0.996917333733128,1.,0.996917333733128,1.,0.996917333733128,1.,0.996917333733128,
1.,0.996917333733128,1.,0.996917333733128,1.,0.996917333733128,1.,0.996917333733128,
1.,0.996917333733128,1.,0.996917333733128,1.,0.996917333733128,1.,0.996917333733128,
1.,0.996917333733128,1.,0.996917333733128,1.,0.996917333733128,1.,0.996917333733128,
1.,0.996917333733128,1.,0.996917333733128,1.),(1.,0.996917333733128,1.,
0.996917333733128,1.,0.996917333733128,1.,0.996917333733128,1.,0.996917333733128,
1.,0.996917333733128,1.,0.996917333733128,1.,0.996917333733128,1.,0.996917333733128,
1.,0.996917333733128,1.,0.996917333733128,1.,0.996917333733128,1.,0.996917333733128,
1.,0.996917333733128,1.,0.996917333733128,1.,0.996917333733128,1.,0.996917333733128,
1.,0.996917333733128,1.,0.996917333733128,1.,0.996917333733128,1.,0.996917333733128,
1.,0.996917333733128,1.,0.996917333733128,1.,0.996917333733128,1.,0.996917333733128,
1.,0.996917333733128,1.,0.996917333733128,1.,0.996917333733128,1.,0.996917333733128,
1.,0.996917333733128,1.,0.996917333733128,1.,0.996917333733128,1.,0.996917333733128,
1.,0.996917333733128,1.,0.996917333733128,1.,0.996917333733128,1.,0.996917333733128,
1.,0.996917333733128,1.,0.996917333733128,1.,0.996917333733128,1.)))
REPRESENTATION_ITEM('')
SURFACE()
);
#4029=(
BOUNDED_SURFACE()
B_SPLINE_SURFACE(1,2,((#268129,#268130,#268131,#268132,#268133,#268134,
#268135,#268136,#268137,#268138,#268139,#268140,#268141,#268142,#268143,
#268144,#268145,#268146,#268147,#268148,#268149,#268150,#268151,#268152,
#268153,#268154,#268155,#268156,#268157,#268158,#268159,#268160,#268161,
#268162,#268163,#268164,#268165,#268166,#268167,#268168,#268169,#268170,
#268171,#268172,#268173,#268174,#268175,#268176,#268177,#268178,#268179,
#268180,#268181,#268182,#268183,#268184,#268185,#268186,#268187,#268188,
#268189,#268190,#268191,#268192,#268193,#268194,#268195,#268196,#268197,
#268198,#268199,#268200,#268201,#268202,#268203,#268204,#268205,#268206,
#268207,#268208,#268209),(#268210,#268211,#268212,#268213,#268214,#268215,
#268216,#268217,#268218,#268219,#268220,#268221,#268222,#268223,#268224,
#268225,#268226,#268227,#268228,#268229,#268230,#268231,#268232,#268233,
#268234,#268235,#268236,#268237,#268238,#268239,#268240,#268241,#268242,
#268243,#268244,#268245,#268246,#268247,#268248,#268249,#268250,#268251,
#268252,#268253,#268254,#268255,#268256,#268257,#268258,#268259,#268260,
#268261,#268262,#268263,#268264,#268265,#268266,#268267,#268268,#268269,
#268270,#268271,#268272,#268273,#268274,#268275,#268276,#268277,#268278,
#268279,#268280,#268281,#268282,#268283,#268284,#268285,#268286,#268287,
#268288,#268289,#268290)),.UNSPECIFIED.,.F.,.F.,.F.)
B_SPLINE_SURFACE_WITH_KNOTS((2,2),(3,2,2,2,2,2,2,2,2,2,2,2,2,2,2,2,2,2,
2,2,2,2,2,2,2,2,2,2,2,2,2,2,2,2,2,2,2,2,2,2,3),(0.,1.),(0.,0.025,0.05,0.075,
0.1,0.125,0.15,0.175,0.2,0.225,0.25,0.275,0.3,0.325,0.35,0.375,0.4,0.425,
0.45,0.475,0.5,0.525,0.55,0.575,0.6,0.625,0.65,0.675,0.7,0.725,0.75,0.775,
0.8,0.825,0.85,0.875,0.9,0.925,0.95,0.975,1.),.UNSPECIFIED.)
GEOMETRIC_REPRESENTATION_ITEM()
RATIONAL_B_SPLINE_SURFACE(((1.,0.996917333733128,1.,0.996917333733128,1.,
0.996917333733128,1.,0.996917333733128,1.,0.996917333733128,1.,0.996917333733128,
1.,0.996917333733128,1.,0.996917333733128,1.,0.996917333733128,1.,0.996917333733128,
1.,0.996917333733128,1.,0.996917333733128,1.,0.996917333733128,1.,0.996917333733128,
1.,0.996917333733128,1.,0.996917333733128,1.,0.996917333733128,1.,0.996917333733128,
1.,0.996917333733128,1.,0.996917333733128,1.,0.996917333733128,1.,0.996917333733128,
1.,0.996917333733128,1.,0.996917333733128,1.,0.996917333733128,1.,0.996917333733128,
1.,0.996917333733128,1.,0.996917333733128,1.,0.996917333733128,1.,0.996917333733128,
1.,0.996917333733128,1.,0.996917333733128,1.,0.996917333733128,1.,0.996917333733128,
1.,0.996917333733128,1.,0.996917333733128,1.,0.996917333733128,1.,0.996917333733128,
1.,0.996917333733128,1.,0.996917333733128,1.),(1.,0.996917333733128,1.,
0.996917333733128,1.,0.996917333733128,1.,0.996917333733128,1.,0.996917333733128,
1.,0.996917333733128,1.,0.996917333733128,1.,0.996917333733128,1.,0.996917333733128,
1.,0.996917333733128,1.,0.996917333733128,1.,0.996917333733128,1.,0.996917333733128,
1.,0.996917333733128,1.,0.996917333733128,1.,0.996917333733128,1.,0.996917333733128,
1.,0.996917333733128,1.,0.996917333733128,1.,0.996917333733128,1.,0.996917333733128,
1.,0.996917333733128,1.,0.996917333733128,1.,0.996917333733128,1.,0.996917333733128,
1.,0.996917333733128,1.,0.996917333733128,1.,0.996917333733128,1.,0.996917333733128,
1.,0.996917333733128,1.,0.996917333733128,1.,0.996917333733128,1.,0.996917333733128,
1.,0.996917333733128,1.,0.996917333733128,1.,0.996917333733128,1.,0.996917333733128,
1.,0.996917333733128,1.,0.996917333733128,1.,0.996917333733128,1.)))
REPRESENTATION_ITEM('')
SURFACE()
);
#4030=(
BOUNDED_SURFACE()
B_SPLINE_SURFACE(1,2,((#268292,#268293,#268294,#268295,#268296,#268297,
#268298,#268299,#268300,#268301,#268302,#268303,#268304,#268305,#268306,
#268307,#268308,#268309,#268310,#268311,#268312,#268313,#268314,#268315,
#268316,#268317,#268318,#268319,#268320,#268321,#268322,#268323,#268324,
#268325,#268326,#268327,#268328,#268329,#268330,#268331,#268332,#268333,
#268334,#268335,#268336,#268337,#268338,#268339,#268340,#268341,#268342,
#268343,#268344,#268345,#268346,#268347,#268348,#268349,#268350,#268351,
#268352,#268353,#268354,#268355,#268356,#268357,#268358,#268359,#268360,
#268361,#268362,#268363,#268364,#268365,#268366,#268367,#268368,#268369,
#268370,#268371,#268372),(#268373,#268374,#268375,#268376,#268377,#268378,
#268379,#268380,#268381,#268382,#268383,#268384,#268385,#268386,#268387,
#268388,#268389,#268390,#268391,#268392,#268393,#268394,#268395,#268396,
#268397,#268398,#268399,#268400,#268401,#268402,#268403,#268404,#268405,
#268406,#268407,#268408,#268409,#268410,#268411,#268412,#268413,#268414,
#268415,#268416,#268417,#268418,#268419,#268420,#268421,#268422,#268423,
#268424,#268425,#268426,#268427,#268428,#268429,#268430,#268431,#268432,
#268433,#268434,#268435,#268436,#268437,#268438,#268439,#268440,#268441,
#268442,#268443,#268444,#268445,#268446,#268447,#268448,#268449,#268450,
#268451,#268452,#268453)),.UNSPECIFIED.,.F.,.F.,.F.)
B_SPLINE_SURFACE_WITH_KNOTS((2,2),(3,2,2,2,2,2,2,2,2,2,2,2,2,2,2,2,2,2,
2,2,2,2,2,2,2,2,2,2,2,2,2,2,2,2,2,2,2,2,2,2,3),(0.,1.),(0.,0.025,0.05,0.075,
0.1,0.125,0.15,0.175,0.2,0.225,0.25,0.275,0.3,0.325,0.35,0.375,0.4,0.425,
0.45,0.475,0.5,0.525,0.55,0.575,0.6,0.625,0.65,0.675,0.7,0.725,0.75,0.775,
0.8,0.825,0.85,0.875,0.9,0.925,0.95,0.975,1.),.UNSPECIFIED.)
GEOMETRIC_REPRESENTATION_ITEM()
RATIONAL_B_SPLINE_SURFACE(((1.,0.996917333733128,1.,0.996917333733128,1.,
0.996917333733128,1.,0.996917333733128,1.,0.996917333733128,1.,0.996917333733128,
1.,0.996917333733128,1.,0.996917333733128,1.,0.996917333733128,1.,0.996917333733128,
1.,0.996917333733128,1.,0.996917333733128,1.,0.996917333733128,1.,0.996917333733128,
1.,0.996917333733128,1.,0.996917333733128,1.,0.996917333733128,1.,0.996917333733128,
1.,0.996917333733128,1.,0.996917333733128,1.,0.996917333733128,1.,0.996917333733128,
1.,0.996917333733128,1.,0.996917333733128,1.,0.996917333733128,1.,0.996917333733128,
1.,0.996917333733128,1.,0.996917333733128,1.,0.996917333733128,1.,0.996917333733128,
1.,0.996917333733128,1.,0.996917333733128,1.,0.996917333733128,1.,0.996917333733128,
1.,0.996917333733128,1.,0.996917333733128,1.,0.996917333733128,1.,0.996917333733128,
1.,0.996917333733128,1.,0.996917333733128,1.),(1.,0.996917333733128,1.,
0.996917333733128,1.,0.996917333733128,1.,0.996917333733128,1.,0.996917333733128,
1.,0.996917333733128,1.,0.996917333733128,1.,0.996917333733128,1.,0.996917333733128,
1.,0.996917333733128,1.,0.996917333733128,1.,0.996917333733128,1.,0.996917333733128,
1.,0.996917333733128,1.,0.996917333733128,1.,0.996917333733128,1.,0.996917333733128,
1.,0.996917333733128,1.,0.996917333733128,1.,0.996917333733128,1.,0.996917333733128,
1.,0.996917333733128,1.,0.996917333733128,1.,0.996917333733128,1.,0.996917333733128,
1.,0.996917333733128,1.,0.996917333733128,1.,0.996917333733128,1.,0.996917333733128,
1.,0.996917333733128,1.,0.996917333733128,1.,0.996917333733128,1.,0.996917333733128,
1.,0.996917333733128,1.,0.996917333733128,1.,0.996917333733128,1.,0.996917333733128,
1.,0.996917333733128,1.,0.996917333733128,1.,0.996917333733128,1.)))
REPRESENTATION_ITEM('')
SURFACE()
);
#4031=(
BOUNDED_SURFACE()
B_SPLINE_SURFACE(1,2,((#268454,#268455,#268456,#268457,#268458,#268459,
#268460,#268461,#268462,#268463,#268464,#268465,#268466,#268467,#268468,
#268469,#268470,#268471,#268472,#268473,#268474,#268475,#268476,#268477,
#268478,#268479,#268480,#268481,#268482,#268483,#268484,#268485,#268486,
#268487,#268488,#268489,#268490,#268491,#268492,#268493,#268494,#268495,
#268496,#268497,#268498,#268499,#268500,#268501,#268502,#268503,#268504,
#268505,#268506,#268507,#268508,#268509,#268510,#268511,#268512,#268513,
#268514,#268515,#268516,#268517,#268518,#268519,#268520,#268521,#268522,
#268523,#268524,#268525,#268526,#268527,#268528,#268529,#268530,#268531,
#268532,#268533,#268534),(#268535,#268536,#268537,#268538,#268539,#268540,
#268541,#268542,#268543,#268544,#268545,#268546,#268547,#268548,#268549,
#268550,#268551,#268552,#268553,#268554,#268555,#268556,#268557,#268558,
#268559,#268560,#268561,#268562,#268563,#268564,#268565,#268566,#268567,
#268568,#268569,#268570,#268571,#268572,#268573,#268574,#268575,#268576,
#268577,#268578,#268579,#268580,#268581,#268582,#268583,#268584,#268585,
#268586,#268587,#268588,#268589,#268590,#268591,#268592,#268593,#268594,
#268595,#268596,#268597,#268598,#268599,#268600,#268601,#268602,#268603,
#268604,#268605,#268606,#268607,#268608,#268609,#268610,#268611,#268612,
#268613,#268614,#268615)),.UNSPECIFIED.,.F.,.F.,.F.)
B_SPLINE_SURFACE_WITH_KNOTS((2,2),(3,2,2,2,2,2,2,2,2,2,2,2,2,2,2,2,2,2,
2,2,2,2,2,2,2,2,2,2,2,2,2,2,2,2,2,2,2,2,2,2,3),(0.,1.),(0.,0.025,0.05,0.075,
0.1,0.125,0.15,0.175,0.2,0.225,0.25,0.275,0.3,0.325,0.35,0.375,0.4,0.425,
0.45,0.475,0.5,0.525,0.55,0.575,0.6,0.625,0.65,0.675,0.7,0.725,0.75,0.775,
0.8,0.825,0.85,0.875,0.9,0.925,0.95,0.975,1.),.UNSPECIFIED.)
GEOMETRIC_REPRESENTATION_ITEM()
RATIONAL_B_SPLINE_SURFACE(((1.,0.996917333733128,1.,0.996917333733128,1.,
0.996917333733128,1.,0.996917333733128,1.,0.996917333733128,1.,0.996917333733128,
1.,0.996917333733128,1.,0.996917333733128,1.,0.996917333733128,1.,0.996917333733128,
1.,0.996917333733128,1.,0.996917333733128,1.,0.996917333733128,1.,0.996917333733128,
1.,0.996917333733128,1.,0.996917333733128,1.,0.996917333733128,1.,0.996917333733128,
1.,0.996917333733128,1.,0.996917333733128,1.,0.996917333733128,1.,0.996917333733128,
1.,0.996917333733128,1.,0.996917333733128,1.,0.996917333733128,1.,0.996917333733128,
1.,0.996917333733128,1.,0.996917333733128,1.,0.996917333733128,1.,0.996917333733128,
1.,0.996917333733128,1.,0.996917333733128,1.,0.996917333733128,1.,0.996917333733128,
1.,0.996917333733128,1.,0.996917333733128,1.,0.996917333733128,1.,0.996917333733128,
1.,0.996917333733128,1.,0.996917333733128,1.),(1.,0.996917333733128,1.,
0.996917333733128,1.,0.996917333733128,1.,0.996917333733128,1.,0.996917333733128,
1.,0.996917333733128,1.,0.996917333733128,1.,0.996917333733128,1.,0.996917333733128,
1.,0.996917333733128,1.,0.996917333733128,1.,0.996917333733128,1.,0.996917333733128,
1.,0.996917333733128,1.,0.996917333733128,1.,0.996917333733128,1.,0.996917333733128,
1.,0.996917333733128,1.,0.996917333733128,1.,0.996917333733128,1.,0.996917333733128,
1.,0.996917333733128,1.,0.996917333733128,1.,0.996917333733128,1.,0.996917333733128,
1.,0.996917333733128,1.,0.996917333733128,1.,0.996917333733128,1.,0.996917333733128,
1.,0.996917333733128,1.,0.996917333733128,1.,0.996917333733128,1.,0.996917333733128,
1.,0.996917333733128,1.,0.996917333733128,1.,0.996917333733128,1.,0.996917333733128,
1.,0.996917333733128,1.,0.996917333733128,1.,0.996917333733128,1.)))
REPRESENTATION_ITEM('')
SURFACE()
);
#4032=(
BOUNDED_SURFACE()
B_SPLINE_SURFACE(1,2,((#268617,#268618,#268619,#268620,#268621,#268622,
#268623,#268624,#268625,#268626,#268627,#268628,#268629,#268630,#268631,
#268632,#268633,#268634,#268635,#268636,#268637,#268638,#268639,#268640,
#268641,#268642,#268643,#268644,#268645,#268646,#268647,#268648,#268649,
#268650,#268651,#268652,#268653,#268654,#268655,#268656,#268657,#268658,
#268659,#268660,#268661,#268662,#268663,#268664,#268665,#268666,#268667,
#268668,#268669,#268670,#268671,#268672,#268673,#268674,#268675,#268676,
#268677,#268678,#268679,#268680,#268681,#268682,#268683,#268684,#268685,
#268686,#268687,#268688,#268689,#268690,#268691,#268692,#268693,#268694,
#268695,#268696,#268697),(#268698,#268699,#268700,#268701,#268702,#268703,
#268704,#268705,#268706,#268707,#268708,#268709,#268710,#268711,#268712,
#268713,#268714,#268715,#268716,#268717,#268718,#268719,#268720,#268721,
#268722,#268723,#268724,#268725,#268726,#268727,#268728,#268729,#268730,
#268731,#268732,#268733,#268734,#268735,#268736,#268737,#268738,#268739,
#268740,#268741,#268742,#268743,#268744,#268745,#268746,#268747,#268748,
#268749,#268750,#268751,#268752,#268753,#268754,#268755,#268756,#268757,
#268758,#268759,#268760,#268761,#268762,#268763,#268764,#268765,#268766,
#268767,#268768,#268769,#268770,#268771,#268772,#268773,#268774,#268775,
#268776,#268777,#268778)),.UNSPECIFIED.,.F.,.F.,.F.)
B_SPLINE_SURFACE_WITH_KNOTS((2,2),(3,2,2,2,2,2,2,2,2,2,2,2,2,2,2,2,2,2,
2,2,2,2,2,2,2,2,2,2,2,2,2,2,2,2,2,2,2,2,2,2,3),(0.,1.),(0.,0.025,0.05,0.075,
0.1,0.125,0.15,0.175,0.2,0.225,0.25,0.275,0.3,0.325,0.35,0.375,0.4,0.425,
0.45,0.475,0.5,0.525,0.55,0.575,0.6,0.625,0.65,0.675,0.7,0.725,0.75,0.775,
0.8,0.825,0.85,0.875,0.9,0.925,0.95,0.975,1.),.UNSPECIFIED.)
GEOMETRIC_REPRESENTATION_ITEM()
RATIONAL_B_SPLINE_SURFACE(((1.,0.996917333733128,1.,0.996917333733128,1.,
0.996917333733128,1.,0.996917333733128,1.,0.996917333733128,1.,0.996917333733128,
1.,0.996917333733128,1.,0.996917333733128,1.,0.996917333733128,1.,0.996917333733128,
1.,0.996917333733128,1.,0.996917333733128,1.,0.996917333733128,1.,0.996917333733128,
1.,0.996917333733128,1.,0.996917333733128,1.,0.996917333733128,1.,0.996917333733128,
1.,0.996917333733128,1.,0.996917333733128,1.,0.996917333733128,1.,0.996917333733128,
1.,0.996917333733128,1.,0.996917333733128,1.,0.996917333733128,1.,0.996917333733128,
1.,0.996917333733128,1.,0.996917333733128,1.,0.996917333733128,1.,0.996917333733128,
1.,0.996917333733128,1.,0.996917333733128,1.,0.996917333733128,1.,0.996917333733128,
1.,0.996917333733128,1.,0.996917333733128,1.,0.996917333733128,1.,0.996917333733128,
1.,0.996917333733128,1.,0.996917333733128,1.),(1.,0.996917333733128,1.,
0.996917333733128,1.,0.996917333733128,1.,0.996917333733128,1.,0.996917333733128,
1.,0.996917333733128,1.,0.996917333733128,1.,0.996917333733128,1.,0.996917333733128,
1.,0.996917333733128,1.,0.996917333733128,1.,0.996917333733128,1.,0.996917333733128,
1.,0.996917333733128,1.,0.996917333733128,1.,0.996917333733128,1.,0.996917333733128,
1.,0.996917333733128,1.,0.996917333733128,1.,0.996917333733128,1.,0.996917333733128,
1.,0.996917333733128,1.,0.996917333733128,1.,0.996917333733128,1.,0.996917333733128,
1.,0.996917333733128,1.,0.996917333733128,1.,0.996917333733128,1.,0.996917333733128,
1.,0.996917333733128,1.,0.996917333733128,1.,0.996917333733128,1.,0.996917333733128,
1.,0.996917333733128,1.,0.996917333733128,1.,0.996917333733128,1.,0.996917333733128,
1.,0.996917333733128,1.,0.996917333733128,1.,0.996917333733128,1.)))
REPRESENTATION_ITEM('')
SURFACE()
);
#4033=(
BOUNDED_SURFACE()
B_SPLINE_SURFACE(1,2,((#268779,#268780,#268781,#268782,#268783,#268784,
#268785,#268786,#268787,#268788,#268789,#268790,#268791,#268792,#268793,
#268794,#268795,#268796,#268797,#268798,#268799,#268800,#268801,#268802,
#268803,#268804,#268805,#268806,#268807,#268808,#268809,#268810,#268811,
#268812,#268813,#268814,#268815,#268816,#268817,#268818,#268819,#268820,
#268821,#268822,#268823,#268824,#268825,#268826,#268827,#268828,#268829,
#268830,#268831,#268832,#268833,#268834,#268835,#268836,#268837,#268838,
#268839,#268840,#268841,#268842,#268843,#268844,#268845,#268846,#268847,
#268848,#268849,#268850,#268851,#268852,#268853,#268854,#268855,#268856,
#268857,#268858,#268859),(#268860,#268861,#268862,#268863,#268864,#268865,
#268866,#268867,#268868,#268869,#268870,#268871,#268872,#268873,#268874,
#268875,#268876,#268877,#268878,#268879,#268880,#268881,#268882,#268883,
#268884,#268885,#268886,#268887,#268888,#268889,#268890,#268891,#268892,
#268893,#268894,#268895,#268896,#268897,#268898,#268899,#268900,#268901,
#268902,#268903,#268904,#268905,#268906,#268907,#268908,#268909,#268910,
#268911,#268912,#268913,#268914,#268915,#268916,#268917,#268918,#268919,
#268920,#268921,#268922,#268923,#268924,#268925,#268926,#268927,#268928,
#268929,#268930,#268931,#268932,#268933,#268934,#268935,#268936,#268937,
#268938,#268939,#268940)),.UNSPECIFIED.,.F.,.F.,.F.)
B_SPLINE_SURFACE_WITH_KNOTS((2,2),(3,2,2,2,2,2,2,2,2,2,2,2,2,2,2,2,2,2,
2,2,2,2,2,2,2,2,2,2,2,2,2,2,2,2,2,2,2,2,2,2,3),(0.,1.),(0.,0.025,0.05,0.075,
0.1,0.125,0.15,0.175,0.2,0.225,0.25,0.275,0.3,0.325,0.35,0.375,0.4,0.425,
0.45,0.475,0.5,0.525,0.55,0.575,0.6,0.625,0.65,0.675,0.7,0.725,0.75,0.775,
0.8,0.825,0.85,0.875,0.9,0.925,0.95,0.975,1.),.UNSPECIFIED.)
GEOMETRIC_REPRESENTATION_ITEM()
RATIONAL_B_SPLINE_SURFACE(((1.,0.996917333733128,1.,0.996917333733128,1.,
0.996917333733128,1.,0.996917333733128,1.,0.996917333733128,1.,0.996917333733128,
1.,0.996917333733128,1.,0.996917333733128,1.,0.996917333733128,1.,0.996917333733128,
1.,0.996917333733128,1.,0.996917333733128,1.,0.996917333733128,1.,0.996917333733128,
1.,0.996917333733128,1.,0.996917333733128,1.,0.996917333733128,1.,0.996917333733128,
1.,0.996917333733128,1.,0.996917333733128,1.,0.996917333733128,1.,0.996917333733128,
1.,0.996917333733128,1.,0.996917333733128,1.,0.996917333733128,1.,0.996917333733128,
1.,0.996917333733128,1.,0.996917333733128,1.,0.996917333733128,1.,0.996917333733128,
1.,0.996917333733128,1.,0.996917333733128,1.,0.996917333733128,1.,0.996917333733128,
1.,0.996917333733128,1.,0.996917333733128,1.,0.996917333733128,1.,0.996917333733128,
1.,0.996917333733128,1.,0.996917333733128,1.),(1.,0.996917333733128,1.,
0.996917333733128,1.,0.996917333733128,1.,0.996917333733128,1.,0.996917333733128,
1.,0.996917333733128,1.,0.996917333733128,1.,0.996917333733128,1.,0.996917333733128,
1.,0.996917333733128,1.,0.996917333733128,1.,0.996917333733128,1.,0.996917333733128,
1.,0.996917333733128,1.,0.996917333733128,1.,0.996917333733128,1.,0.996917333733128,
1.,0.996917333733128,1.,0.996917333733128,1.,0.996917333733128,1.,0.996917333733128,
1.,0.996917333733128,1.,0.996917333733128,1.,0.996917333733128,1.,0.996917333733128,
1.,0.996917333733128,1.,0.996917333733128,1.,0.996917333733128,1.,0.996917333733128,
1.,0.996917333733128,1.,0.996917333733128,1.,0.996917333733128,1.,0.996917333733128,
1.,0.996917333733128,1.,0.996917333733128,1.,0.996917333733128,1.,0.996917333733128,
1.,0.996917333733128,1.,0.996917333733128,1.,0.996917333733128,1.)))
REPRESENTATION_ITEM('')
SURFACE()
);
#4034=(
BOUNDED_SURFACE()
B_SPLINE_SURFACE(1,2,((#269103,#269104,#269105,#269106,#269107,#269108,
#269109,#269110,#269111,#269112,#269113,#269114,#269115,#269116,#269117,
#269118,#269119,#269120,#269121,#269122,#269123,#269124,#269125,#269126,
#269127,#269128,#269129,#269130,#269131,#269132,#269133,#269134,#269135,
#269136,#269137,#269138,#269139,#269140,#269141,#269142,#269143,#269144,
#269145,#269146,#269147,#269148,#269149,#269150,#269151,#269152,#269153,
#269154,#269155,#269156,#269157,#269158,#269159,#269160,#269161,#269162,
#269163,#269164,#269165,#269166,#269167,#269168,#269169,#269170,#269171,
#269172,#269173,#269174,#269175,#269176,#269177,#269178,#269179,#269180,
#269181,#269182,#269183),(#269184,#269185,#269186,#269187,#269188,#269189,
#269190,#269191,#269192,#269193,#269194,#269195,#269196,#269197,#269198,
#269199,#269200,#269201,#269202,#269203,#269204,#269205,#269206,#269207,
#269208,#269209,#269210,#269211,#269212,#269213,#269214,#269215,#269216,
#269217,#269218,#269219,#269220,#269221,#269222,#269223,#269224,#269225,
#269226,#269227,#269228,#269229,#269230,#269231,#269232,#269233,#269234,
#269235,#269236,#269237,#269238,#269239,#269240,#269241,#269242,#269243,
#269244,#269245,#269246,#269247,#269248,#269249,#269250,#269251,#269252,
#269253,#269254,#269255,#269256,#269257,#269258,#269259,#269260,#269261,
#269262,#269263,#269264)),.UNSPECIFIED.,.F.,.F.,.F.)
B_SPLINE_SURFACE_WITH_KNOTS((2,2),(3,2,2,2,2,2,2,2,2,2,2,2,2,2,2,2,2,2,
2,2,2,2,2,2,2,2,2,2,2,2,2,2,2,2,2,2,2,2,2,2,3),(0.,1.),(0.,0.025,0.05,0.075,
0.1,0.125,0.15,0.175,0.2,0.225,0.25,0.275,0.3,0.325,0.35,0.375,0.4,0.425,
0.45,0.475,0.5,0.525,0.55,0.575,0.6,0.625,0.65,0.675,0.7,0.725,0.75,0.775,
0.8,0.825,0.85,0.875,0.9,0.925,0.95,0.975,1.),.UNSPECIFIED.)
GEOMETRIC_REPRESENTATION_ITEM()
RATIONAL_B_SPLINE_SURFACE(((1.,0.996917333733128,1.,0.996917333733128,1.,
0.996917333733128,1.,0.996917333733128,1.,0.996917333733128,1.,0.996917333733128,
1.,0.996917333733128,1.,0.996917333733128,1.,0.996917333733128,1.,0.996917333733128,
1.,0.996917333733128,1.,0.996917333733128,1.,0.996917333733128,1.,0.996917333733128,
1.,0.996917333733128,1.,0.996917333733128,1.,0.996917333733128,1.,0.996917333733128,
1.,0.996917333733128,1.,0.996917333733128,1.,0.996917333733128,1.,0.996917333733128,
1.,0.996917333733128,1.,0.996917333733128,1.,0.996917333733128,1.,0.996917333733128,
1.,0.996917333733128,1.,0.996917333733128,1.,0.996917333733128,1.,0.996917333733128,
1.,0.996917333733128,1.,0.996917333733128,1.,0.996917333733128,1.,0.996917333733128,
1.,0.996917333733128,1.,0.996917333733128,1.,0.996917333733128,1.,0.996917333733128,
1.,0.996917333733128,1.,0.996917333733128,1.),(1.,0.996917333733128,1.,
0.996917333733128,1.,0.996917333733128,1.,0.996917333733128,1.,0.996917333733128,
1.,0.996917333733128,1.,0.996917333733128,1.,0.996917333733128,1.,0.996917333733128,
1.,0.996917333733128,1.,0.996917333733128,1.,0.996917333733128,1.,0.996917333733128,
1.,0.996917333733128,1.,0.996917333733128,1.,0.996917333733128,1.,0.996917333733128,
1.,0.996917333733128,1.,0.996917333733128,1.,0.996917333733128,1.,0.996917333733128,
1.,0.996917333733128,1.,0.996917333733128,1.,0.996917333733128,1.,0.996917333733128,
1.,0.996917333733128,1.,0.996917333733128,1.,0.996917333733128,1.,0.996917333733128,
1.,0.996917333733128,1.,0.996917333733128,1.,0.996917333733128,1.,0.996917333733128,
1.,0.996917333733128,1.,0.996917333733128,1.,0.996917333733128,1.,0.996917333733128,
1.,0.996917333733128,1.,0.996917333733128,1.,0.996917333733128,1.)))
REPRESENTATION_ITEM('')
SURFACE()
);
#4035=(
BOUNDED_SURFACE()
B_SPLINE_SURFACE(1,2,((#269346,#269347,#269348,#269349,#269350,#269351,
#269352,#269353,#269354,#269355,#269356,#269357,#269358,#269359,#269360,
#269361,#269362,#269363,#269364,#269365,#269366,#269367,#269368,#269369,
#269370,#269371,#269372,#269373,#269374,#269375,#269376,#269377,#269378,
#269379,#269380,#269381,#269382,#269383,#269384,#269385,#269386,#269387,
#269388,#269389,#269390,#269391,#269392,#269393,#269394,#269395,#269396,
#269397,#269398,#269399,#269400,#269401,#269402,#269403,#269404,#269405,
#269406,#269407,#269408,#269409,#269410,#269411,#269412,#269413,#269414,
#269415,#269416,#269417,#269418,#269419,#269420,#269421,#269422,#269423,
#269424,#269425,#269426),(#269427,#269428,#269429,#269430,#269431,#269432,
#269433,#269434,#269435,#269436,#269437,#269438,#269439,#269440,#269441,
#269442,#269443,#269444,#269445,#269446,#269447,#269448,#269449,#269450,
#269451,#269452,#269453,#269454,#269455,#269456,#269457,#269458,#269459,
#269460,#269461,#269462,#269463,#269464,#269465,#269466,#269467,#269468,
#269469,#269470,#269471,#269472,#269473,#269474,#269475,#269476,#269477,
#269478,#269479,#269480,#269481,#269482,#269483,#269484,#269485,#269486,
#269487,#269488,#269489,#269490,#269491,#269492,#269493,#269494,#269495,
#269496,#269497,#269498,#269499,#269500,#269501,#269502,#269503,#269504,
#269505,#269506,#269507)),.UNSPECIFIED.,.F.,.F.,.F.)
B_SPLINE_SURFACE_WITH_KNOTS((2,2),(3,2,2,2,2,2,2,2,2,2,2,2,2,2,2,2,2,2,
2,2,2,2,2,2,2,2,2,2,2,2,2,2,2,2,2,2,2,2,2,2,3),(0.,1.),(0.,0.025,0.05,0.075,
0.1,0.125,0.15,0.175,0.2,0.225,0.25,0.275,0.3,0.325,0.35,0.375,0.4,0.425,
0.45,0.475,0.5,0.525,0.55,0.575,0.6,0.625,0.65,0.675,0.7,0.725,0.75,0.775,
0.8,0.825,0.85,0.875,0.9,0.925,0.95,0.975,1.),.UNSPECIFIED.)
GEOMETRIC_REPRESENTATION_ITEM()
RATIONAL_B_SPLINE_SURFACE(((1.,0.996917333733128,1.,0.996917333733128,1.,
0.996917333733128,1.,0.996917333733128,1.,0.996917333733128,1.,0.996917333733128,
1.,0.996917333733128,1.,0.996917333733128,1.,0.996917333733128,1.,0.996917333733128,
1.,0.996917333733128,1.,0.996917333733128,1.,0.996917333733128,1.,0.996917333733128,
1.,0.996917333733128,1.,0.996917333733128,1.,0.996917333733128,1.,0.996917333733128,
1.,0.996917333733128,1.,0.996917333733128,1.,0.996917333733128,1.,0.996917333733128,
1.,0.996917333733128,1.,0.996917333733128,1.,0.996917333733128,1.,0.996917333733128,
1.,0.996917333733128,1.,0.996917333733128,1.,0.996917333733128,1.,0.996917333733128,
1.,0.996917333733128,1.,0.996917333733128,1.,0.996917333733128,1.,0.996917333733128,
1.,0.996917333733128,1.,0.996917333733128,1.,0.996917333733128,1.,0.996917333733128,
1.,0.996917333733128,1.,0.996917333733128,1.),(1.,0.996917333733128,1.,
0.996917333733128,1.,0.996917333733128,1.,0.996917333733128,1.,0.996917333733128,
1.,0.996917333733128,1.,0.996917333733128,1.,0.996917333733128,1.,0.996917333733128,
1.,0.996917333733128,1.,0.996917333733128,1.,0.996917333733128,1.,0.996917333733128,
1.,0.996917333733128,1.,0.996917333733128,1.,0.996917333733128,1.,0.996917333733128,
1.,0.996917333733128,1.,0.996917333733128,1.,0.996917333733128,1.,0.996917333733128,
1.,0.996917333733128,1.,0.996917333733128,1.,0.996917333733128,1.,0.996917333733128,
1.,0.996917333733128,1.,0.996917333733128,1.,0.996917333733128,1.,0.996917333733128,
1.,0.996917333733128,1.,0.996917333733128,1.,0.996917333733128,1.,0.996917333733128,
1.,0.996917333733128,1.,0.996917333733128,1.,0.996917333733128,1.,0.996917333733128,
1.,0.996917333733128,1.,0.996917333733128,1.,0.996917333733128,1.)))
REPRESENTATION_ITEM('')
SURFACE()
);
#4036=(
BOUNDED_SURFACE()
B_SPLINE_SURFACE(1,2,((#269589,#269590,#269591,#269592,#269593,#269594,
#269595,#269596,#269597,#269598,#269599,#269600,#269601,#269602,#269603,
#269604,#269605,#269606,#269607,#269608,#269609,#269610,#269611,#269612,
#269613,#269614,#269615,#269616,#269617,#269618,#269619,#269620,#269621,
#269622,#269623,#269624,#269625,#269626,#269627,#269628,#269629,#269630,
#269631,#269632,#269633,#269634,#269635,#269636,#269637,#269638,#269639,
#269640,#269641,#269642,#269643,#269644,#269645,#269646,#269647,#269648,
#269649,#269650,#269651,#269652,#269653,#269654,#269655,#269656,#269657,
#269658,#269659,#269660,#269661,#269662,#269663,#269664,#269665,#269666,
#269667,#269668,#269669),(#269670,#269671,#269672,#269673,#269674,#269675,
#269676,#269677,#269678,#269679,#269680,#269681,#269682,#269683,#269684,
#269685,#269686,#269687,#269688,#269689,#269690,#269691,#269692,#269693,
#269694,#269695,#269696,#269697,#269698,#269699,#269700,#269701,#269702,
#269703,#269704,#269705,#269706,#269707,#269708,#269709,#269710,#269711,
#269712,#269713,#269714,#269715,#269716,#269717,#269718,#269719,#269720,
#269721,#269722,#269723,#269724,#269725,#269726,#269727,#269728,#269729,
#269730,#269731,#269732,#269733,#269734,#269735,#269736,#269737,#269738,
#269739,#269740,#269741,#269742,#269743,#269744,#269745,#269746,#269747,
#269748,#269749,#269750)),.UNSPECIFIED.,.F.,.F.,.F.)
B_SPLINE_SURFACE_WITH_KNOTS((2,2),(3,2,2,2,2,2,2,2,2,2,2,2,2,2,2,2,2,2,
2,2,2,2,2,2,2,2,2,2,2,2,2,2,2,2,2,2,2,2,2,2,3),(0.,1.),(0.,0.025,0.05,0.075,
0.1,0.125,0.15,0.175,0.2,0.225,0.25,0.275,0.3,0.325,0.35,0.375,0.4,0.425,
0.45,0.475,0.5,0.525,0.55,0.575,0.6,0.625,0.65,0.675,0.7,0.725,0.75,0.775,
0.8,0.825,0.85,0.875,0.9,0.925,0.95,0.975,1.),.UNSPECIFIED.)
GEOMETRIC_REPRESENTATION_ITEM()
RATIONAL_B_SPLINE_SURFACE(((1.,0.996917333733128,1.,0.996917333733128,1.,
0.996917333733128,1.,0.996917333733128,1.,0.996917333733128,1.,0.996917333733128,
1.,0.996917333733128,1.,0.996917333733128,1.,0.996917333733128,1.,0.996917333733128,
1.,0.996917333733128,1.,0.996917333733128,1.,0.996917333733128,1.,0.996917333733128,
1.,0.996917333733128,1.,0.996917333733128,1.,0.996917333733128,1.,0.996917333733128,
1.,0.996917333733128,1.,0.996917333733128,1.,0.996917333733128,1.,0.996917333733128,
1.,0.996917333733128,1.,0.996917333733128,1.,0.996917333733128,1.,0.996917333733128,
1.,0.996917333733128,1.,0.996917333733128,1.,0.996917333733128,1.,0.996917333733128,
1.,0.996917333733128,1.,0.996917333733128,1.,0.996917333733128,1.,0.996917333733128,
1.,0.996917333733128,1.,0.996917333733128,1.,0.996917333733128,1.,0.996917333733128,
1.,0.996917333733128,1.,0.996917333733128,1.),(1.,0.996917333733128,1.,
0.996917333733128,1.,0.996917333733128,1.,0.996917333733128,1.,0.996917333733128,
1.,0.996917333733128,1.,0.996917333733128,1.,0.996917333733128,1.,0.996917333733128,
1.,0.996917333733128,1.,0.996917333733128,1.,0.996917333733128,1.,0.996917333733128,
1.,0.996917333733128,1.,0.996917333733128,1.,0.996917333733128,1.,0.996917333733128,
1.,0.996917333733128,1.,0.996917333733128,1.,0.996917333733128,1.,0.996917333733128,
1.,0.996917333733128,1.,0.996917333733128,1.,0.996917333733128,1.,0.996917333733128,
1.,0.996917333733128,1.,0.996917333733128,1.,0.996917333733128,1.,0.996917333733128,
1.,0.996917333733128,1.,0.996917333733128,1.,0.996917333733128,1.,0.996917333733128,
1.,0.996917333733128,1.,0.996917333733128,1.,0.996917333733128,1.,0.996917333733128,
1.,0.996917333733128,1.,0.996917333733128,1.,0.996917333733128,1.)))
REPRESENTATION_ITEM('')
SURFACE()
);
#4037=(
BOUNDED_SURFACE()
B_SPLINE_SURFACE(1,2,((#269751,#269752,#269753,#269754,#269755,#269756,
#269757,#269758,#269759,#269760,#269761,#269762,#269763,#269764,#269765,
#269766,#269767,#269768,#269769,#269770,#269771,#269772,#269773,#269774,
#269775,#269776,#269777,#269778,#269779,#269780,#269781,#269782,#269783,
#269784,#269785,#269786,#269787,#269788,#269789,#269790,#269791,#269792,
#269793,#269794,#269795,#269796,#269797,#269798,#269799,#269800,#269801,
#269802,#269803,#269804,#269805,#269806,#269807,#269808,#269809,#269810,
#269811,#269812,#269813,#269814,#269815,#269816,#269817,#269818,#269819,
#269820,#269821,#269822,#269823,#269824,#269825,#269826,#269827,#269828,
#269829,#269830,#269831),(#269832,#269833,#269834,#269835,#269836,#269837,
#269838,#269839,#269840,#269841,#269842,#269843,#269844,#269845,#269846,
#269847,#269848,#269849,#269850,#269851,#269852,#269853,#269854,#269855,
#269856,#269857,#269858,#269859,#269860,#269861,#269862,#269863,#269864,
#269865,#269866,#269867,#269868,#269869,#269870,#269871,#269872,#269873,
#269874,#269875,#269876,#269877,#269878,#269879,#269880,#269881,#269882,
#269883,#269884,#269885,#269886,#269887,#269888,#269889,#269890,#269891,
#269892,#269893,#269894,#269895,#269896,#269897,#269898,#269899,#269900,
#269901,#269902,#269903,#269904,#269905,#269906,#269907,#269908,#269909,
#269910,#269911,#269912)),.UNSPECIFIED.,.F.,.F.,.F.)
B_SPLINE_SURFACE_WITH_KNOTS((2,2),(3,2,2,2,2,2,2,2,2,2,2,2,2,2,2,2,2,2,
2,2,2,2,2,2,2,2,2,2,2,2,2,2,2,2,2,2,2,2,2,2,3),(0.,1.),(0.,0.025,0.05,0.075,
0.1,0.125,0.15,0.175,0.2,0.225,0.25,0.275,0.3,0.325,0.35,0.375,0.4,0.425,
0.45,0.475,0.5,0.525,0.55,0.575,0.6,0.625,0.65,0.675,0.7,0.725,0.75,0.775,
0.8,0.825,0.85,0.875,0.9,0.925,0.95,0.975,1.),.UNSPECIFIED.)
GEOMETRIC_REPRESENTATION_ITEM()
RATIONAL_B_SPLINE_SURFACE(((1.,0.996917333733128,1.,0.996917333733128,1.,
0.996917333733128,1.,0.996917333733128,1.,0.996917333733128,1.,0.996917333733128,
1.,0.996917333733128,1.,0.996917333733128,1.,0.996917333733128,1.,0.996917333733128,
1.,0.996917333733128,1.,0.996917333733128,1.,0.996917333733128,1.,0.996917333733128,
1.,0.996917333733128,1.,0.996917333733128,1.,0.996917333733128,1.,0.996917333733128,
1.,0.996917333733128,1.,0.996917333733128,1.,0.996917333733128,1.,0.996917333733128,
1.,0.996917333733128,1.,0.996917333733128,1.,0.996917333733128,1.,0.996917333733128,
1.,0.996917333733128,1.,0.996917333733128,1.,0.996917333733128,1.,0.996917333733128,
1.,0.996917333733128,1.,0.996917333733128,1.,0.996917333733128,1.,0.996917333733128,
1.,0.996917333733128,1.,0.996917333733128,1.,0.996917333733128,1.,0.996917333733128,
1.,0.996917333733128,1.,0.996917333733128,1.),(1.,0.996917333733128,1.,
0.996917333733128,1.,0.996917333733128,1.,0.996917333733128,1.,0.996917333733128,
1.,0.996917333733128,1.,0.996917333733128,1.,0.996917333733128,1.,0.996917333733128,
1.,0.996917333733128,1.,0.996917333733128,1.,0.996917333733128,1.,0.996917333733128,
1.,0.996917333733128,1.,0.996917333733128,1.,0.996917333733128,1.,0.996917333733128,
1.,0.996917333733128,1.,0.996917333733128,1.,0.996917333733128,1.,0.996917333733128,
1.,0.996917333733128,1.,0.996917333733128,1.,0.996917333733128,1.,0.996917333733128,
1.,0.996917333733128,1.,0.996917333733128,1.,0.996917333733128,1.,0.996917333733128,
1.,0.996917333733128,1.,0.996917333733128,1.,0.996917333733128,1.,0.996917333733128,
1.,0.996917333733128,1.,0.996917333733128,1.,0.996917333733128,1.,0.996917333733128,
1.,0.996917333733128,1.,0.996917333733128,1.,0.996917333733128,1.)))
REPRESENTATION_ITEM('')
SURFACE()
);
#4038=(
BOUNDED_SURFACE()
B_SPLINE_SURFACE(1,2,((#270075,#270076,#270077,#270078,#270079,#270080,
#270081,#270082,#270083,#270084,#270085,#270086,#270087,#270088,#270089,
#270090,#270091,#270092,#270093,#270094,#270095,#270096,#270097,#270098,
#270099,#270100,#270101,#270102,#270103,#270104,#270105,#270106,#270107,
#270108,#270109,#270110,#270111,#270112,#270113,#270114,#270115,#270116,
#270117,#270118,#270119,#270120,#270121,#270122,#270123,#270124,#270125,
#270126,#270127,#270128,#270129,#270130,#270131,#270132,#270133,#270134,
#270135,#270136,#270137,#270138,#270139,#270140,#270141,#270142,#270143,
#270144,#270145,#270146,#270147,#270148,#270149,#270150,#270151,#270152,
#270153,#270154,#270155),(#270156,#270157,#270158,#270159,#270160,#270161,
#270162,#270163,#270164,#270165,#270166,#270167,#270168,#270169,#270170,
#270171,#270172,#270173,#270174,#270175,#270176,#270177,#270178,#270179,
#270180,#270181,#270182,#270183,#270184,#270185,#270186,#270187,#270188,
#270189,#270190,#270191,#270192,#270193,#270194,#270195,#270196,#270197,
#270198,#270199,#270200,#270201,#270202,#270203,#270204,#270205,#270206,
#270207,#270208,#270209,#270210,#270211,#270212,#270213,#270214,#270215,
#270216,#270217,#270218,#270219,#270220,#270221,#270222,#270223,#270224,
#270225,#270226,#270227,#270228,#270229,#270230,#270231,#270232,#270233,
#270234,#270235,#270236)),.UNSPECIFIED.,.F.,.F.,.F.)
B_SPLINE_SURFACE_WITH_KNOTS((2,2),(3,2,2,2,2,2,2,2,2,2,2,2,2,2,2,2,2,2,
2,2,2,2,2,2,2,2,2,2,2,2,2,2,2,2,2,2,2,2,2,2,3),(0.,1.),(0.,0.025,0.05,0.075,
0.1,0.125,0.15,0.175,0.2,0.225,0.25,0.275,0.3,0.325,0.35,0.375,0.4,0.425,
0.45,0.475,0.5,0.525,0.55,0.575,0.6,0.625,0.65,0.675,0.7,0.725,0.75,0.775,
0.8,0.825,0.85,0.875,0.9,0.925,0.95,0.975,1.),.UNSPECIFIED.)
GEOMETRIC_REPRESENTATION_ITEM()
RATIONAL_B_SPLINE_SURFACE(((1.,0.996917333733128,1.,0.996917333733128,1.,
0.996917333733128,1.,0.996917333733128,1.,0.996917333733128,1.,0.996917333733128,
1.,0.996917333733128,1.,0.996917333733128,1.,0.996917333733128,1.,0.996917333733128,
1.,0.996917333733128,1.,0.996917333733128,1.,0.996917333733128,1.,0.996917333733128,
1.,0.996917333733128,1.,0.996917333733128,1.,0.996917333733128,1.,0.996917333733128,
1.,0.996917333733128,1.,0.996917333733128,1.,0.996917333733128,1.,0.996917333733128,
1.,0.996917333733128,1.,0.996917333733128,1.,0.996917333733128,1.,0.996917333733128,
1.,0.996917333733128,1.,0.996917333733128,1.,0.996917333733128,1.,0.996917333733128,
1.,0.996917333733128,1.,0.996917333733128,1.,0.996917333733128,1.,0.996917333733128,
1.,0.996917333733128,1.,0.996917333733128,1.,0.996917333733128,1.,0.996917333733128,
1.,0.996917333733128,1.,0.996917333733128,1.),(1.,0.996917333733128,1.,
0.996917333733128,1.,0.996917333733128,1.,0.996917333733128,1.,0.996917333733128,
1.,0.996917333733128,1.,0.996917333733128,1.,0.996917333733128,1.,0.996917333733128,
1.,0.996917333733128,1.,0.996917333733128,1.,0.996917333733128,1.,0.996917333733128,
1.,0.996917333733128,1.,0.996917333733128,1.,0.996917333733128,1.,0.996917333733128,
1.,0.996917333733128,1.,0.996917333733128,1.,0.996917333733128,1.,0.996917333733128,
1.,0.996917333733128,1.,0.996917333733128,1.,0.996917333733128,1.,0.996917333733128,
1.,0.996917333733128,1.,0.996917333733128,1.,0.996917333733128,1.,0.996917333733128,
1.,0.996917333733128,1.,0.996917333733128,1.,0.996917333733128,1.,0.996917333733128,
1.,0.996917333733128,1.,0.996917333733128,1.,0.996917333733128,1.,0.996917333733128,
1.,0.996917333733128,1.,0.996917333733128,1.,0.996917333733128,1.)))
REPRESENTATION_ITEM('')
SURFACE()
);
#4039=(
BOUNDED_SURFACE()
B_SPLINE_SURFACE(1,2,((#270318,#270319,#270320,#270321,#270322,#270323,
#270324,#270325,#270326,#270327,#270328,#270329,#270330,#270331,#270332,
#270333,#270334,#270335,#270336,#270337,#270338,#270339,#270340,#270341,
#270342,#270343,#270344,#270345,#270346,#270347,#270348,#270349,#270350,
#270351,#270352,#270353,#270354,#270355,#270356,#270357,#270358,#270359,
#270360,#270361,#270362,#270363,#270364,#270365,#270366,#270367,#270368,
#270369,#270370,#270371,#270372,#270373,#270374,#270375,#270376,#270377,
#270378,#270379,#270380,#270381,#270382,#270383,#270384,#270385,#270386,
#270387,#270388,#270389,#270390,#270391,#270392,#270393,#270394,#270395,
#270396,#270397,#270398),(#270399,#270400,#270401,#270402,#270403,#270404,
#270405,#270406,#270407,#270408,#270409,#270410,#270411,#270412,#270413,
#270414,#270415,#270416,#270417,#270418,#270419,#270420,#270421,#270422,
#270423,#270424,#270425,#270426,#270427,#270428,#270429,#270430,#270431,
#270432,#270433,#270434,#270435,#270436,#270437,#270438,#270439,#270440,
#270441,#270442,#270443,#270444,#270445,#270446,#270447,#270448,#270449,
#270450,#270451,#270452,#270453,#270454,#270455,#270456,#270457,#270458,
#270459,#270460,#270461,#270462,#270463,#270464,#270465,#270466,#270467,
#270468,#270469,#270470,#270471,#270472,#270473,#270474,#270475,#270476,
#270477,#270478,#270479)),.UNSPECIFIED.,.F.,.F.,.F.)
B_SPLINE_SURFACE_WITH_KNOTS((2,2),(3,2,2,2,2,2,2,2,2,2,2,2,2,2,2,2,2,2,
2,2,2,2,2,2,2,2,2,2,2,2,2,2,2,2,2,2,2,2,2,2,3),(0.,1.),(0.,0.025,0.05,0.075,
0.1,0.125,0.15,0.175,0.2,0.225,0.25,0.275,0.3,0.325,0.35,0.375,0.4,0.425,
0.45,0.475,0.5,0.525,0.55,0.575,0.6,0.625,0.65,0.675,0.7,0.725,0.75,0.775,
0.8,0.825,0.85,0.875,0.9,0.925,0.95,0.975,1.),.UNSPECIFIED.)
GEOMETRIC_REPRESENTATION_ITEM()
RATIONAL_B_SPLINE_SURFACE(((1.,0.996917333733128,1.,0.996917333733128,1.,
0.996917333733128,1.,0.996917333733128,1.,0.996917333733128,1.,0.996917333733128,
1.,0.996917333733128,1.,0.996917333733128,1.,0.996917333733128,1.,0.996917333733128,
1.,0.996917333733128,1.,0.996917333733128,1.,0.996917333733128,1.,0.996917333733128,
1.,0.996917333733128,1.,0.996917333733128,1.,0.996917333733128,1.,0.996917333733128,
1.,0.996917333733128,1.,0.996917333733128,1.,0.996917333733128,1.,0.996917333733128,
1.,0.996917333733128,1.,0.996917333733128,1.,0.996917333733128,1.,0.996917333733128,
1.,0.996917333733128,1.,0.996917333733128,1.,0.996917333733128,1.,0.996917333733128,
1.,0.996917333733128,1.,0.996917333733128,1.,0.996917333733128,1.,0.996917333733128,
1.,0.996917333733128,1.,0.996917333733128,1.,0.996917333733128,1.,0.996917333733128,
1.,0.996917333733128,1.,0.996917333733128,1.),(1.,0.996917333733128,1.,
0.996917333733128,1.,0.996917333733128,1.,0.996917333733128,1.,0.996917333733128,
1.,0.996917333733128,1.,0.996917333733128,1.,0.996917333733128,1.,0.996917333733128,
1.,0.996917333733128,1.,0.996917333733128,1.,0.996917333733128,1.,0.996917333733128,
1.,0.996917333733128,1.,0.996917333733128,1.,0.996917333733128,1.,0.996917333733128,
1.,0.996917333733128,1.,0.996917333733128,1.,0.996917333733128,1.,0.996917333733128,
1.,0.996917333733128,1.,0.996917333733128,1.,0.996917333733128,1.,0.996917333733128,
1.,0.996917333733128,1.,0.996917333733128,1.,0.996917333733128,1.,0.996917333733128,
1.,0.996917333733128,1.,0.996917333733128,1.,0.996917333733128,1.,0.996917333733128,
1.,0.996917333733128,1.,0.996917333733128,1.,0.996917333733128,1.,0.996917333733128,
1.,0.996917333733128,1.,0.996917333733128,1.,0.996917333733128,1.)))
REPRESENTATION_ITEM('')
SURFACE()
);
#4040=(
BOUNDED_SURFACE()
B_SPLINE_SURFACE(1,2,((#270561,#270562,#270563,#270564,#270565,#270566,
#270567,#270568,#270569,#270570,#270571,#270572,#270573,#270574,#270575,
#270576,#270577,#270578,#270579,#270580,#270581,#270582,#270583,#270584,
#270585,#270586,#270587,#270588,#270589,#270590,#270591,#270592,#270593,
#270594,#270595,#270596,#270597,#270598,#270599,#270600,#270601,#270602,
#270603,#270604,#270605,#270606,#270607,#270608,#270609,#270610,#270611,
#270612,#270613,#270614,#270615,#270616,#270617,#270618,#270619,#270620,
#270621,#270622,#270623,#270624,#270625,#270626,#270627,#270628,#270629,
#270630,#270631,#270632,#270633,#270634,#270635,#270636,#270637,#270638,
#270639,#270640,#270641),(#270642,#270643,#270644,#270645,#270646,#270647,
#270648,#270649,#270650,#270651,#270652,#270653,#270654,#270655,#270656,
#270657,#270658,#270659,#270660,#270661,#270662,#270663,#270664,#270665,
#270666,#270667,#270668,#270669,#270670,#270671,#270672,#270673,#270674,
#270675,#270676,#270677,#270678,#270679,#270680,#270681,#270682,#270683,
#270684,#270685,#270686,#270687,#270688,#270689,#270690,#270691,#270692,
#270693,#270694,#270695,#270696,#270697,#270698,#270699,#270700,#270701,
#270702,#270703,#270704,#270705,#270706,#270707,#270708,#270709,#270710,
#270711,#270712,#270713,#270714,#270715,#270716,#270717,#270718,#270719,
#270720,#270721,#270722)),.UNSPECIFIED.,.F.,.F.,.F.)
B_SPLINE_SURFACE_WITH_KNOTS((2,2),(3,2,2,2,2,2,2,2,2,2,2,2,2,2,2,2,2,2,
2,2,2,2,2,2,2,2,2,2,2,2,2,2,2,2,2,2,2,2,2,2,3),(0.,1.),(0.,0.025,0.05,0.075,
0.1,0.125,0.15,0.175,0.2,0.225,0.25,0.275,0.3,0.325,0.35,0.375,0.4,0.425,
0.45,0.475,0.5,0.525,0.55,0.575,0.6,0.625,0.65,0.675,0.7,0.725,0.75,0.775,
0.8,0.825,0.85,0.875,0.9,0.925,0.95,0.975,1.),.UNSPECIFIED.)
GEOMETRIC_REPRESENTATION_ITEM()
RATIONAL_B_SPLINE_SURFACE(((1.,0.996917333733128,1.,0.996917333733128,1.,
0.996917333733128,1.,0.996917333733128,1.,0.996917333733128,1.,0.996917333733128,
1.,0.996917333733128,1.,0.996917333733128,1.,0.996917333733128,1.,0.996917333733128,
1.,0.996917333733128,1.,0.996917333733128,1.,0.996917333733128,1.,0.996917333733128,
1.,0.996917333733128,1.,0.996917333733128,1.,0.996917333733128,1.,0.996917333733128,
1.,0.996917333733128,1.,0.996917333733128,1.,0.996917333733128,1.,0.996917333733128,
1.,0.996917333733128,1.,0.996917333733128,1.,0.996917333733128,1.,0.996917333733128,
1.,0.996917333733128,1.,0.996917333733128,1.,0.996917333733128,1.,0.996917333733128,
1.,0.996917333733128,1.,0.996917333733128,1.,0.996917333733128,1.,0.996917333733128,
1.,0.996917333733128,1.,0.996917333733128,1.,0.996917333733128,1.,0.996917333733128,
1.,0.996917333733128,1.,0.996917333733128,1.),(1.,0.996917333733128,1.,
0.996917333733128,1.,0.996917333733128,1.,0.996917333733128,1.,0.996917333733128,
1.,0.996917333733128,1.,0.996917333733128,1.,0.996917333733128,1.,0.996917333733128,
1.,0.996917333733128,1.,0.996917333733128,1.,0.996917333733128,1.,0.996917333733128,
1.,0.996917333733128,1.,0.996917333733128,1.,0.996917333733128,1.,0.996917333733128,
1.,0.996917333733128,1.,0.996917333733128,1.,0.996917333733128,1.,0.996917333733128,
1.,0.996917333733128,1.,0.996917333733128,1.,0.996917333733128,1.,0.996917333733128,
1.,0.996917333733128,1.,0.996917333733128,1.,0.996917333733128,1.,0.996917333733128,
1.,0.996917333733128,1.,0.996917333733128,1.,0.996917333733128,1.,0.996917333733128,
1.,0.996917333733128,1.,0.996917333733128,1.,0.996917333733128,1.,0.996917333733128,
1.,0.996917333733128,1.,0.996917333733128,1.,0.996917333733128,1.)))
REPRESENTATION_ITEM('')
SURFACE()
);
#4041=(
BOUNDED_SURFACE()
B_SPLINE_SURFACE(1,2,((#270723,#270724,#270725,#270726,#270727,#270728,
#270729,#270730,#270731,#270732,#270733,#270734,#270735,#270736,#270737,
#270738,#270739,#270740,#270741,#270742,#270743,#270744,#270745,#270746,
#270747,#270748,#270749,#270750,#270751,#270752,#270753,#270754,#270755,
#270756,#270757,#270758,#270759,#270760,#270761,#270762,#270763,#270764,
#270765,#270766,#270767,#270768,#270769,#270770,#270771,#270772,#270773,
#270774,#270775,#270776,#270777,#270778,#270779,#270780,#270781,#270782,
#270783,#270784,#270785,#270786,#270787,#270788,#270789,#270790,#270791,
#270792,#270793,#270794,#270795,#270796,#270797,#270798,#270799,#270800,
#270801,#270802,#270803),(#270804,#270805,#270806,#270807,#270808,#270809,
#270810,#270811,#270812,#270813,#270814,#270815,#270816,#270817,#270818,
#270819,#270820,#270821,#270822,#270823,#270824,#270825,#270826,#270827,
#270828,#270829,#270830,#270831,#270832,#270833,#270834,#270835,#270836,
#270837,#270838,#270839,#270840,#270841,#270842,#270843,#270844,#270845,
#270846,#270847,#270848,#270849,#270850,#270851,#270852,#270853,#270854,
#270855,#270856,#270857,#270858,#270859,#270860,#270861,#270862,#270863,
#270864,#270865,#270866,#270867,#270868,#270869,#270870,#270871,#270872,
#270873,#270874,#270875,#270876,#270877,#270878,#270879,#270880,#270881,
#270882,#270883,#270884)),.UNSPECIFIED.,.F.,.F.,.F.)
B_SPLINE_SURFACE_WITH_KNOTS((2,2),(3,2,2,2,2,2,2,2,2,2,2,2,2,2,2,2,2,2,
2,2,2,2,2,2,2,2,2,2,2,2,2,2,2,2,2,2,2,2,2,2,3),(0.,1.),(0.,0.025,0.05,0.075,
0.1,0.125,0.15,0.175,0.2,0.225,0.25,0.275,0.3,0.325,0.35,0.375,0.4,0.425,
0.45,0.475,0.5,0.525,0.55,0.575,0.6,0.625,0.65,0.675,0.7,0.725,0.75,0.775,
0.8,0.825,0.85,0.875,0.9,0.925,0.95,0.975,1.),.UNSPECIFIED.)
GEOMETRIC_REPRESENTATION_ITEM()
RATIONAL_B_SPLINE_SURFACE(((1.,0.996917333733128,1.,0.996917333733128,1.,
0.996917333733128,1.,0.996917333733128,1.,0.996917333733128,1.,0.996917333733128,
1.,0.996917333733128,1.,0.996917333733128,1.,0.996917333733128,1.,0.996917333733128,
1.,0.996917333733128,1.,0.996917333733128,1.,0.996917333733128,1.,0.996917333733128,
1.,0.996917333733128,1.,0.996917333733128,1.,0.996917333733128,1.,0.996917333733128,
1.,0.996917333733128,1.,0.996917333733128,1.,0.996917333733128,1.,0.996917333733128,
1.,0.996917333733128,1.,0.996917333733128,1.,0.996917333733128,1.,0.996917333733128,
1.,0.996917333733128,1.,0.996917333733128,1.,0.996917333733128,1.,0.996917333733128,
1.,0.996917333733128,1.,0.996917333733128,1.,0.996917333733128,1.,0.996917333733128,
1.,0.996917333733128,1.,0.996917333733128,1.,0.996917333733128,1.,0.996917333733128,
1.,0.996917333733128,1.,0.996917333733128,1.),(1.,0.996917333733128,1.,
0.996917333733128,1.,0.996917333733128,1.,0.996917333733128,1.,0.996917333733128,
1.,0.996917333733128,1.,0.996917333733128,1.,0.996917333733128,1.,0.996917333733128,
1.,0.996917333733128,1.,0.996917333733128,1.,0.996917333733128,1.,0.996917333733128,
1.,0.996917333733128,1.,0.996917333733128,1.,0.996917333733128,1.,0.996917333733128,
1.,0.996917333733128,1.,0.996917333733128,1.,0.996917333733128,1.,0.996917333733128,
1.,0.996917333733128,1.,0.996917333733128,1.,0.996917333733128,1.,0.996917333733128,
1.,0.996917333733128,1.,0.996917333733128,1.,0.996917333733128,1.,0.996917333733128,
1.,0.996917333733128,1.,0.996917333733128,1.,0.996917333733128,1.,0.996917333733128,
1.,0.996917333733128,1.,0.996917333733128,1.,0.996917333733128,1.,0.996917333733128,
1.,0.996917333733128,1.,0.996917333733128,1.,0.996917333733128,1.)))
REPRESENTATION_ITEM('')
SURFACE()
);
#4042=(
BOUNDED_SURFACE()
B_SPLINE_SURFACE(1,2,((#271047,#271048,#271049,#271050,#271051,#271052,
#271053,#271054,#271055,#271056,#271057,#271058,#271059,#271060,#271061,
#271062,#271063,#271064,#271065,#271066,#271067,#271068,#271069,#271070,
#271071,#271072,#271073,#271074,#271075,#271076,#271077,#271078,#271079,
#271080,#271081,#271082,#271083,#271084,#271085,#271086,#271087,#271088,
#271089,#271090,#271091,#271092,#271093,#271094,#271095,#271096,#271097,
#271098,#271099,#271100,#271101,#271102,#271103,#271104,#271105,#271106,
#271107,#271108,#271109,#271110,#271111,#271112,#271113,#271114,#271115,
#271116,#271117,#271118,#271119,#271120,#271121,#271122,#271123,#271124,
#271125,#271126,#271127),(#271128,#271129,#271130,#271131,#271132,#271133,
#271134,#271135,#271136,#271137,#271138,#271139,#271140,#271141,#271142,
#271143,#271144,#271145,#271146,#271147,#271148,#271149,#271150,#271151,
#271152,#271153,#271154,#271155,#271156,#271157,#271158,#271159,#271160,
#271161,#271162,#271163,#271164,#271165,#271166,#271167,#271168,#271169,
#271170,#271171,#271172,#271173,#271174,#271175,#271176,#271177,#271178,
#271179,#271180,#271181,#271182,#271183,#271184,#271185,#271186,#271187,
#271188,#271189,#271190,#271191,#271192,#271193,#271194,#271195,#271196,
#271197,#271198,#271199,#271200,#271201,#271202,#271203,#271204,#271205,
#271206,#271207,#271208)),.UNSPECIFIED.,.F.,.F.,.F.)
B_SPLINE_SURFACE_WITH_KNOTS((2,2),(3,2,2,2,2,2,2,2,2,2,2,2,2,2,2,2,2,2,
2,2,2,2,2,2,2,2,2,2,2,2,2,2,2,2,2,2,2,2,2,2,3),(0.,1.),(0.,0.025,0.05,0.075,
0.1,0.125,0.15,0.175,0.2,0.225,0.25,0.275,0.3,0.325,0.35,0.375,0.4,0.425,
0.45,0.475,0.5,0.525,0.55,0.575,0.6,0.625,0.65,0.675,0.7,0.725,0.75,0.775,
0.8,0.825,0.85,0.875,0.9,0.925,0.95,0.975,1.),.UNSPECIFIED.)
GEOMETRIC_REPRESENTATION_ITEM()
RATIONAL_B_SPLINE_SURFACE(((1.,0.996917333733128,1.,0.996917333733128,1.,
0.996917333733128,1.,0.996917333733128,1.,0.996917333733128,1.,0.996917333733128,
1.,0.996917333733128,1.,0.996917333733128,1.,0.996917333733128,1.,0.996917333733128,
1.,0.996917333733128,1.,0.996917333733128,1.,0.996917333733128,1.,0.996917333733128,
1.,0.996917333733128,1.,0.996917333733128,1.,0.996917333733128,1.,0.996917333733128,
1.,0.996917333733128,1.,0.996917333733128,1.,0.996917333733128,1.,0.996917333733128,
1.,0.996917333733128,1.,0.996917333733128,1.,0.996917333733128,1.,0.996917333733128,
1.,0.996917333733128,1.,0.996917333733128,1.,0.996917333733128,1.,0.996917333733128,
1.,0.996917333733128,1.,0.996917333733128,1.,0.996917333733128,1.,0.996917333733128,
1.,0.996917333733128,1.,0.996917333733128,1.,0.996917333733128,1.,0.996917333733128,
1.,0.996917333733128,1.,0.996917333733128,1.),(1.,0.996917333733128,1.,
0.996917333733128,1.,0.996917333733128,1.,0.996917333733128,1.,0.996917333733128,
1.,0.996917333733128,1.,0.996917333733128,1.,0.996917333733128,1.,0.996917333733128,
1.,0.996917333733128,1.,0.996917333733128,1.,0.996917333733128,1.,0.996917333733128,
1.,0.996917333733128,1.,0.996917333733128,1.,0.996917333733128,1.,0.996917333733128,
1.,0.996917333733128,1.,0.996917333733128,1.,0.996917333733128,1.,0.996917333733128,
1.,0.996917333733128,1.,0.996917333733128,1.,0.996917333733128,1.,0.996917333733128,
1.,0.996917333733128,1.,0.996917333733128,1.,0.996917333733128,1.,0.996917333733128,
1.,0.996917333733128,1.,0.996917333733128,1.,0.996917333733128,1.,0.996917333733128,
1.,0.996917333733128,1.,0.996917333733128,1.,0.996917333733128,1.,0.996917333733128,
1.,0.996917333733128,1.,0.996917333733128,1.,0.996917333733128,1.)))
REPRESENTATION_ITEM('')
SURFACE()
);
#4043=(
BOUNDED_SURFACE()
B_SPLINE_SURFACE(1,2,((#271290,#271291,#271292,#271293,#271294,#271295,
#271296,#271297,#271298,#271299,#271300,#271301,#271302,#271303,#271304,
#271305,#271306,#271307,#271308,#271309,#271310,#271311,#271312,#271313,
#271314,#271315,#271316,#271317,#271318,#271319,#271320,#271321,#271322,
#271323,#271324,#271325,#271326,#271327,#271328,#271329,#271330,#271331,
#271332,#271333,#271334,#271335,#271336,#271337,#271338,#271339,#271340,
#271341,#271342,#271343,#271344,#271345,#271346,#271347,#271348,#271349,
#271350,#271351,#271352,#271353,#271354,#271355,#271356,#271357,#271358,
#271359,#271360,#271361,#271362,#271363,#271364,#271365,#271366,#271367,
#271368,#271369,#271370),(#271371,#271372,#271373,#271374,#271375,#271376,
#271377,#271378,#271379,#271380,#271381,#271382,#271383,#271384,#271385,
#271386,#271387,#271388,#271389,#271390,#271391,#271392,#271393,#271394,
#271395,#271396,#271397,#271398,#271399,#271400,#271401,#271402,#271403,
#271404,#271405,#271406,#271407,#271408,#271409,#271410,#271411,#271412,
#271413,#271414,#271415,#271416,#271417,#271418,#271419,#271420,#271421,
#271422,#271423,#271424,#271425,#271426,#271427,#271428,#271429,#271430,
#271431,#271432,#271433,#271434,#271435,#271436,#271437,#271438,#271439,
#271440,#271441,#271442,#271443,#271444,#271445,#271446,#271447,#271448,
#271449,#271450,#271451)),.UNSPECIFIED.,.F.,.F.,.F.)
B_SPLINE_SURFACE_WITH_KNOTS((2,2),(3,2,2,2,2,2,2,2,2,2,2,2,2,2,2,2,2,2,
2,2,2,2,2,2,2,2,2,2,2,2,2,2,2,2,2,2,2,2,2,2,3),(0.,1.),(0.,0.025,0.05,0.075,
0.1,0.125,0.15,0.175,0.2,0.225,0.25,0.275,0.3,0.325,0.35,0.375,0.4,0.425,
0.45,0.475,0.5,0.525,0.55,0.575,0.6,0.625,0.65,0.675,0.7,0.725,0.75,0.775,
0.8,0.825,0.85,0.875,0.9,0.925,0.95,0.975,1.),.UNSPECIFIED.)
GEOMETRIC_REPRESENTATION_ITEM()
RATIONAL_B_SPLINE_SURFACE(((1.,0.996917333733128,1.,0.996917333733128,1.,
0.996917333733128,1.,0.996917333733128,1.,0.996917333733128,1.,0.996917333733128,
1.,0.996917333733128,1.,0.996917333733128,1.,0.996917333733128,1.,0.996917333733128,
1.,0.996917333733128,1.,0.996917333733128,1.,0.996917333733128,1.,0.996917333733128,
1.,0.996917333733128,1.,0.996917333733128,1.,0.996917333733128,1.,0.996917333733128,
1.,0.996917333733128,1.,0.996917333733128,1.,0.996917333733128,1.,0.996917333733128,
1.,0.996917333733128,1.,0.996917333733128,1.,0.996917333733128,1.,0.996917333733128,
1.,0.996917333733128,1.,0.996917333733128,1.,0.996917333733128,1.,0.996917333733128,
1.,0.996917333733128,1.,0.996917333733128,1.,0.996917333733128,1.,0.996917333733128,
1.,0.996917333733128,1.,0.996917333733128,1.,0.996917333733128,1.,0.996917333733128,
1.,0.996917333733128,1.,0.996917333733128,1.),(1.,0.996917333733128,1.,
0.996917333733128,1.,0.996917333733128,1.,0.996917333733128,1.,0.996917333733128,
1.,0.996917333733128,1.,0.996917333733128,1.,0.996917333733128,1.,0.996917333733128,
1.,0.996917333733128,1.,0.996917333733128,1.,0.996917333733128,1.,0.996917333733128,
1.,0.996917333733128,1.,0.996917333733128,1.,0.996917333733128,1.,0.996917333733128,
1.,0.996917333733128,1.,0.996917333733128,1.,0.996917333733128,1.,0.996917333733128,
1.,0.996917333733128,1.,0.996917333733128,1.,0.996917333733128,1.,0.996917333733128,
1.,0.996917333733128,1.,0.996917333733128,1.,0.996917333733128,1.,0.996917333733128,
1.,0.996917333733128,1.,0.996917333733128,1.,0.996917333733128,1.,0.996917333733128,
1.,0.996917333733128,1.,0.996917333733128,1.,0.996917333733128,1.,0.996917333733128,
1.,0.996917333733128,1.,0.996917333733128,1.,0.996917333733128,1.)))
REPRESENTATION_ITEM('')
SURFACE()
);
#4044=(
BOUNDED_SURFACE()
B_SPLINE_SURFACE(1,2,((#271533,#271534,#271535,#271536,#271537,#271538,
#271539,#271540,#271541,#271542,#271543,#271544,#271545,#271546,#271547,
#271548,#271549,#271550,#271551,#271552,#271553,#271554,#271555,#271556,
#271557,#271558,#271559,#271560,#271561,#271562,#271563,#271564,#271565,
#271566,#271567,#271568,#271569,#271570,#271571,#271572,#271573,#271574,
#271575,#271576,#271577,#271578,#271579,#271580,#271581,#271582,#271583,
#271584,#271585,#271586,#271587,#271588,#271589,#271590,#271591,#271592,
#271593,#271594,#271595,#271596,#271597,#271598,#271599,#271600,#271601,
#271602,#271603,#271604,#271605,#271606,#271607,#271608,#271609,#271610,
#271611,#271612,#271613),(#271614,#271615,#271616,#271617,#271618,#271619,
#271620,#271621,#271622,#271623,#271624,#271625,#271626,#271627,#271628,
#271629,#271630,#271631,#271632,#271633,#271634,#271635,#271636,#271637,
#271638,#271639,#271640,#271641,#271642,#271643,#271644,#271645,#271646,
#271647,#271648,#271649,#271650,#271651,#271652,#271653,#271654,#271655,
#271656,#271657,#271658,#271659,#271660,#271661,#271662,#271663,#271664,
#271665,#271666,#271667,#271668,#271669,#271670,#271671,#271672,#271673,
#271674,#271675,#271676,#271677,#271678,#271679,#271680,#271681,#271682,
#271683,#271684,#271685,#271686,#271687,#271688,#271689,#271690,#271691,
#271692,#271693,#271694)),.UNSPECIFIED.,.F.,.F.,.F.)
B_SPLINE_SURFACE_WITH_KNOTS((2,2),(3,2,2,2,2,2,2,2,2,2,2,2,2,2,2,2,2,2,
2,2,2,2,2,2,2,2,2,2,2,2,2,2,2,2,2,2,2,2,2,2,3),(0.,1.),(0.,0.025,0.05,0.075,
0.1,0.125,0.15,0.175,0.2,0.225,0.25,0.275,0.3,0.325,0.35,0.375,0.4,0.425,
0.45,0.475,0.5,0.525,0.55,0.575,0.6,0.625,0.65,0.675,0.7,0.725,0.75,0.775,
0.8,0.825,0.85,0.875,0.9,0.925,0.95,0.975,1.),.UNSPECIFIED.)
GEOMETRIC_REPRESENTATION_ITEM()
RATIONAL_B_SPLINE_SURFACE(((1.,0.996917333733128,1.,0.996917333733128,1.,
0.996917333733128,1.,0.996917333733128,1.,0.996917333733128,1.,0.996917333733128,
1.,0.996917333733128,1.,0.996917333733128,1.,0.996917333733128,1.,0.996917333733128,
1.,0.996917333733128,1.,0.996917333733128,1.,0.996917333733128,1.,0.996917333733128,
1.,0.996917333733128,1.,0.996917333733128,1.,0.996917333733128,1.,0.996917333733128,
1.,0.996917333733128,1.,0.996917333733128,1.,0.996917333733128,1.,0.996917333733128,
1.,0.996917333733128,1.,0.996917333733128,1.,0.996917333733128,1.,0.996917333733128,
1.,0.996917333733128,1.,0.996917333733128,1.,0.996917333733128,1.,0.996917333733128,
1.,0.996917333733128,1.,0.996917333733128,1.,0.996917333733128,1.,0.996917333733128,
1.,0.996917333733128,1.,0.996917333733128,1.,0.996917333733128,1.,0.996917333733128,
1.,0.996917333733128,1.,0.996917333733128,1.),(1.,0.996917333733128,1.,
0.996917333733128,1.,0.996917333733128,1.,0.996917333733128,1.,0.996917333733128,
1.,0.996917333733128,1.,0.996917333733128,1.,0.996917333733128,1.,0.996917333733128,
1.,0.996917333733128,1.,0.996917333733128,1.,0.996917333733128,1.,0.996917333733128,
1.,0.996917333733128,1.,0.996917333733128,1.,0.996917333733128,1.,0.996917333733128,
1.,0.996917333733128,1.,0.996917333733128,1.,0.996917333733128,1.,0.996917333733128,
1.,0.996917333733128,1.,0.996917333733128,1.,0.996917333733128,1.,0.996917333733128,
1.,0.996917333733128,1.,0.996917333733128,1.,0.996917333733128,1.,0.996917333733128,
1.,0.996917333733128,1.,0.996917333733128,1.,0.996917333733128,1.,0.996917333733128,
1.,0.996917333733128,1.,0.996917333733128,1.,0.996917333733128,1.,0.996917333733128,
1.,0.996917333733128,1.,0.996917333733128,1.,0.996917333733128,1.)))
REPRESENTATION_ITEM('')
SURFACE()
);
#4045=(
BOUNDED_SURFACE()
B_SPLINE_SURFACE(1,2,((#271725,#271726,#271727,#271728,#271729,#271730,
#271731,#271732,#271733,#271734,#271735,#271736,#271737,#271738,#271739,
#271740,#271741,#271742,#271743,#271744,#271745,#271746,#271747,#271748,
#271749,#271750,#271751,#271752,#271753,#271754,#271755,#271756,#271757,
#271758,#271759,#271760,#271761,#271762,#271763,#271764,#271765,#271766,
#271767,#271768,#271769,#271770,#271771,#271772,#271773,#271774,#271775,
#271776,#271777,#271778,#271779,#271780,#271781,#271782,#271783,#271784,
#271785,#271786,#271787,#271788,#271789,#271790,#271791,#271792,#271793,
#271794,#271795,#271796,#271797,#271798,#271799,#271800,#271801,#271802,
#271803,#271804,#271805),(#271806,#271807,#271808,#271809,#271810,#271811,
#271812,#271813,#271814,#271815,#271816,#271817,#271818,#271819,#271820,
#271821,#271822,#271823,#271824,#271825,#271826,#271827,#271828,#271829,
#271830,#271831,#271832,#271833,#271834,#271835,#271836,#271837,#271838,
#271839,#271840,#271841,#271842,#271843,#271844,#271845,#271846,#271847,
#271848,#271849,#271850,#271851,#271852,#271853,#271854,#271855,#271856,
#271857,#271858,#271859,#271860,#271861,#271862,#271863,#271864,#271865,
#271866,#271867,#271868,#271869,#271870,#271871,#271872,#271873,#271874,
#271875,#271876,#271877,#271878,#271879,#271880,#271881,#271882,#271883,
#271884,#271885,#271886)),.UNSPECIFIED.,.F.,.F.,.F.)
B_SPLINE_SURFACE_WITH_KNOTS((2,2),(3,2,2,2,2,2,2,2,2,2,2,2,2,2,2,2,2,2,
2,2,2,2,2,2,2,2,2,2,2,2,2,2,2,2,2,2,2,2,2,2,3),(0.,1.),(0.,0.025,0.05,0.075,
0.1,0.125,0.15,0.175,0.2,0.225,0.25,0.275,0.3,0.325,0.35,0.375,0.4,0.425,
0.45,0.475,0.5,0.525,0.55,0.575,0.6,0.625,0.65,0.675,0.7,0.725,0.75,0.775,
0.8,0.825,0.85,0.875,0.9,0.925,0.95,0.975,1.),.UNSPECIFIED.)
GEOMETRIC_REPRESENTATION_ITEM()
RATIONAL_B_SPLINE_SURFACE(((1.,0.996917333733128,1.,0.996917333733128,1.,
0.996917333733128,1.,0.996917333733128,1.,0.996917333733128,1.,0.996917333733128,
1.,0.996917333733128,1.,0.996917333733128,1.,0.996917333733128,1.,0.996917333733128,
1.,0.996917333733128,1.,0.996917333733128,1.,0.996917333733128,1.,0.996917333733128,
1.,0.996917333733128,1.,0.996917333733128,1.,0.996917333733128,1.,0.996917333733128,
1.,0.996917333733128,1.,0.996917333733128,1.,0.996917333733128,1.,0.996917333733128,
1.,0.996917333733128,1.,0.996917333733128,1.,0.996917333733128,1.,0.996917333733128,
1.,0.996917333733128,1.,0.996917333733128,1.,0.996917333733128,1.,0.996917333733128,
1.,0.996917333733128,1.,0.996917333733128,1.,0.996917333733128,1.,0.996917333733128,
1.,0.996917333733128,1.,0.996917333733128,1.,0.996917333733128,1.,0.996917333733128,
1.,0.996917333733128,1.,0.996917333733128,1.),(1.,0.996917333733128,1.,
0.996917333733128,1.,0.996917333733128,1.,0.996917333733128,1.,0.996917333733128,
1.,0.996917333733128,1.,0.996917333733128,1.,0.996917333733128,1.,0.996917333733128,
1.,0.996917333733128,1.,0.996917333733128,1.,0.996917333733128,1.,0.996917333733128,
1.,0.996917333733128,1.,0.996917333733128,1.,0.996917333733128,1.,0.996917333733128,
1.,0.996917333733128,1.,0.996917333733128,1.,0.996917333733128,1.,0.996917333733128,
1.,0.996917333733128,1.,0.996917333733128,1.,0.996917333733128,1.,0.996917333733128,
1.,0.996917333733128,1.,0.996917333733128,1.,0.996917333733128,1.,0.996917333733128,
1.,0.996917333733128,1.,0.996917333733128,1.,0.996917333733128,1.,0.996917333733128,
1.,0.996917333733128,1.,0.996917333733128,1.,0.996917333733128,1.,0.996917333733128,
1.,0.996917333733128,1.,0.996917333733128,1.,0.996917333733128,1.)))
REPRESENTATION_ITEM('')
SURFACE()
);
#4046=(
BOUNDED_SURFACE()
B_SPLINE_SURFACE(1,2,((#271888,#271889,#271890,#271891,#271892,#271893,
#271894,#271895,#271896,#271897,#271898,#271899,#271900,#271901,#271902,
#271903,#271904,#271905,#271906,#271907,#271908,#271909,#271910,#271911,
#271912,#271913,#271914,#271915,#271916,#271917,#271918,#271919,#271920,
#271921,#271922,#271923,#271924,#271925,#271926,#271927,#271928,#271929,
#271930,#271931,#271932,#271933,#271934,#271935,#271936,#271937,#271938,
#271939,#271940,#271941,#271942,#271943,#271944,#271945,#271946,#271947,
#271948,#271949,#271950,#271951,#271952,#271953,#271954,#271955,#271956,
#271957,#271958,#271959,#271960,#271961,#271962,#271963,#271964,#271965,
#271966,#271967,#271968),(#271969,#271970,#271971,#271972,#271973,#271974,
#271975,#271976,#271977,#271978,#271979,#271980,#271981,#271982,#271983,
#271984,#271985,#271986,#271987,#271988,#271989,#271990,#271991,#271992,
#271993,#271994,#271995,#271996,#271997,#271998,#271999,#272000,#272001,
#272002,#272003,#272004,#272005,#272006,#272007,#272008,#272009,#272010,
#272011,#272012,#272013,#272014,#272015,#272016,#272017,#272018,#272019,
#272020,#272021,#272022,#272023,#272024,#272025,#272026,#272027,#272028,
#272029,#272030,#272031,#272032,#272033,#272034,#272035,#272036,#272037,
#272038,#272039,#272040,#272041,#272042,#272043,#272044,#272045,#272046,
#272047,#272048,#272049)),.UNSPECIFIED.,.F.,.F.,.F.)
B_SPLINE_SURFACE_WITH_KNOTS((2,2),(3,2,2,2,2,2,2,2,2,2,2,2,2,2,2,2,2,2,
2,2,2,2,2,2,2,2,2,2,2,2,2,2,2,2,2,2,2,2,2,2,3),(0.,1.),(0.,0.025,0.05,0.075,
0.1,0.125,0.15,0.175,0.2,0.225,0.25,0.275,0.3,0.325,0.35,0.375,0.4,0.425,
0.45,0.475,0.5,0.525,0.55,0.575,0.6,0.625,0.65,0.675,0.7,0.725,0.75,0.775,
0.8,0.825,0.85,0.875,0.9,0.925,0.95,0.975,1.),.UNSPECIFIED.)
GEOMETRIC_REPRESENTATION_ITEM()
RATIONAL_B_SPLINE_SURFACE(((1.,0.996917333733128,1.,0.996917333733128,1.,
0.996917333733128,1.,0.996917333733128,1.,0.996917333733128,1.,0.996917333733128,
1.,0.996917333733128,1.,0.996917333733128,1.,0.996917333733128,1.,0.996917333733128,
1.,0.996917333733128,1.,0.996917333733128,1.,0.996917333733128,1.,0.996917333733128,
1.,0.996917333733128,1.,0.996917333733128,1.,0.996917333733128,1.,0.996917333733128,
1.,0.996917333733128,1.,0.996917333733128,1.,0.996917333733128,1.,0.996917333733128,
1.,0.996917333733128,1.,0.996917333733128,1.,0.996917333733128,1.,0.996917333733128,
1.,0.996917333733128,1.,0.996917333733128,1.,0.996917333733128,1.,0.996917333733128,
1.,0.996917333733128,1.,0.996917333733128,1.,0.996917333733128,1.,0.996917333733128,
1.,0.996917333733128,1.,0.996917333733128,1.,0.996917333733128,1.,0.996917333733128,
1.,0.996917333733128,1.,0.996917333733128,1.),(1.,0.996917333733128,1.,
0.996917333733128,1.,0.996917333733128,1.,0.996917333733128,1.,0.996917333733128,
1.,0.996917333733128,1.,0.996917333733128,1.,0.996917333733128,1.,0.996917333733128,
1.,0.996917333733128,1.,0.996917333733128,1.,0.996917333733128,1.,0.996917333733128,
1.,0.996917333733128,1.,0.996917333733128,1.,0.996917333733128,1.,0.996917333733128,
1.,0.996917333733128,1.,0.996917333733128,1.,0.996917333733128,1.,0.996917333733128,
1.,0.996917333733128,1.,0.996917333733128,1.,0.996917333733128,1.,0.996917333733128,
1.,0.996917333733128,1.,0.996917333733128,1.,0.996917333733128,1.,0.996917333733128,
1.,0.996917333733128,1.,0.996917333733128,1.,0.996917333733128,1.,0.996917333733128,
1.,0.996917333733128,1.,0.996917333733128,1.,0.996917333733128,1.,0.996917333733128,
1.,0.996917333733128,1.,0.996917333733128,1.,0.996917333733128,1.)))
REPRESENTATION_ITEM('')
SURFACE()
);
#4047=(
BOUNDED_SURFACE()
B_SPLINE_SURFACE(1,2,((#272050,#272051,#272052,#272053,#272054,#272055,
#272056,#272057,#272058,#272059,#272060,#272061,#272062,#272063,#272064,
#272065,#272066,#272067,#272068,#272069,#272070,#272071,#272072,#272073,
#272074,#272075,#272076,#272077,#272078,#272079,#272080,#272081,#272082,
#272083,#272084,#272085,#272086,#272087,#272088,#272089,#272090,#272091,
#272092,#272093,#272094,#272095,#272096,#272097,#272098,#272099,#272100,
#272101,#272102,#272103,#272104,#272105,#272106,#272107,#272108,#272109,
#272110,#272111,#272112,#272113,#272114,#272115,#272116,#272117,#272118,
#272119,#272120,#272121,#272122,#272123,#272124,#272125,#272126,#272127,
#272128,#272129,#272130),(#272131,#272132,#272133,#272134,#272135,#272136,
#272137,#272138,#272139,#272140,#272141,#272142,#272143,#272144,#272145,
#272146,#272147,#272148,#272149,#272150,#272151,#272152,#272153,#272154,
#272155,#272156,#272157,#272158,#272159,#272160,#272161,#272162,#272163,
#272164,#272165,#272166,#272167,#272168,#272169,#272170,#272171,#272172,
#272173,#272174,#272175,#272176,#272177,#272178,#272179,#272180,#272181,
#272182,#272183,#272184,#272185,#272186,#272187,#272188,#272189,#272190,
#272191,#272192,#272193,#272194,#272195,#272196,#272197,#272198,#272199,
#272200,#272201,#272202,#272203,#272204,#272205,#272206,#272207,#272208,
#272209,#272210,#272211)),.UNSPECIFIED.,.F.,.F.,.F.)
B_SPLINE_SURFACE_WITH_KNOTS((2,2),(3,2,2,2,2,2,2,2,2,2,2,2,2,2,2,2,2,2,
2,2,2,2,2,2,2,2,2,2,2,2,2,2,2,2,2,2,2,2,2,2,3),(0.,1.),(0.,0.025,0.05,0.075,
0.1,0.125,0.15,0.175,0.2,0.225,0.25,0.275,0.3,0.325,0.35,0.375,0.4,0.425,
0.45,0.475,0.5,0.525,0.55,0.575,0.6,0.625,0.65,0.675,0.7,0.725,0.75,0.775,
0.8,0.825,0.85,0.875,0.9,0.925,0.95,0.975,1.),.UNSPECIFIED.)
GEOMETRIC_REPRESENTATION_ITEM()
RATIONAL_B_SPLINE_SURFACE(((1.,0.996917333733128,1.,0.996917333733128,1.,
0.996917333733128,1.,0.996917333733128,1.,0.996917333733128,1.,0.996917333733128,
1.,0.996917333733128,1.,0.996917333733128,1.,0.996917333733128,1.,0.996917333733128,
1.,0.996917333733128,1.,0.996917333733128,1.,0.996917333733128,1.,0.996917333733128,
1.,0.996917333733128,1.,0.996917333733128,1.,0.996917333733128,1.,0.996917333733128,
1.,0.996917333733128,1.,0.996917333733128,1.,0.996917333733128,1.,0.996917333733128,
1.,0.996917333733128,1.,0.996917333733128,1.,0.996917333733128,1.,0.996917333733128,
1.,0.996917333733128,1.,0.996917333733128,1.,0.996917333733128,1.,0.996917333733128,
1.,0.996917333733128,1.,0.996917333733128,1.,0.996917333733128,1.,0.996917333733128,
1.,0.996917333733128,1.,0.996917333733128,1.,0.996917333733128,1.,0.996917333733128,
1.,0.996917333733128,1.,0.996917333733128,1.),(1.,0.996917333733128,1.,
0.996917333733128,1.,0.996917333733128,1.,0.996917333733128,1.,0.996917333733128,
1.,0.996917333733128,1.,0.996917333733128,1.,0.996917333733128,1.,0.996917333733128,
1.,0.996917333733128,1.,0.996917333733128,1.,0.996917333733128,1.,0.996917333733128,
1.,0.996917333733128,1.,0.996917333733128,1.,0.996917333733128,1.,0.996917333733128,
1.,0.996917333733128,1.,0.996917333733128,1.,0.996917333733128,1.,0.996917333733128,
1.,0.996917333733128,1.,0.996917333733128,1.,0.996917333733128,1.,0.996917333733128,
1.,0.996917333733128,1.,0.996917333733128,1.,0.996917333733128,1.,0.996917333733128,
1.,0.996917333733128,1.,0.996917333733128,1.,0.996917333733128,1.,0.996917333733128,
1.,0.996917333733128,1.,0.996917333733128,1.,0.996917333733128,1.,0.996917333733128,
1.,0.996917333733128,1.,0.996917333733128,1.,0.996917333733128,1.)))
REPRESENTATION_ITEM('')
SURFACE()
);
#4048=(
BOUNDED_SURFACE()
B_SPLINE_SURFACE(1,2,((#272213,#272214,#272215,#272216,#272217,#272218,
#272219,#272220,#272221,#272222,#272223,#272224,#272225,#272226,#272227,
#272228,#272229,#272230,#272231,#272232,#272233,#272234,#272235,#272236,
#272237,#272238,#272239,#272240,#272241,#272242,#272243,#272244,#272245,
#272246,#272247,#272248,#272249,#272250,#272251,#272252,#272253,#272254,
#272255,#272256,#272257,#272258,#272259,#272260,#272261,#272262,#272263,
#272264,#272265,#272266,#272267,#272268,#272269,#272270,#272271,#272272,
#272273,#272274,#272275,#272276,#272277,#272278,#272279,#272280,#272281,
#272282,#272283,#272284,#272285,#272286,#272287,#272288,#272289,#272290,
#272291,#272292,#272293),(#272294,#272295,#272296,#272297,#272298,#272299,
#272300,#272301,#272302,#272303,#272304,#272305,#272306,#272307,#272308,
#272309,#272310,#272311,#272312,#272313,#272314,#272315,#272316,#272317,
#272318,#272319,#272320,#272321,#272322,#272323,#272324,#272325,#272326,
#272327,#272328,#272329,#272330,#272331,#272332,#272333,#272334,#272335,
#272336,#272337,#272338,#272339,#272340,#272341,#272342,#272343,#272344,
#272345,#272346,#272347,#272348,#272349,#272350,#272351,#272352,#272353,
#272354,#272355,#272356,#272357,#272358,#272359,#272360,#272361,#272362,
#272363,#272364,#272365,#272366,#272367,#272368,#272369,#272370,#272371,
#272372,#272373,#272374)),.UNSPECIFIED.,.F.,.F.,.F.)
B_SPLINE_SURFACE_WITH_KNOTS((2,2),(3,2,2,2,2,2,2,2,2,2,2,2,2,2,2,2,2,2,
2,2,2,2,2,2,2,2,2,2,2,2,2,2,2,2,2,2,2,2,2,2,3),(0.,1.),(0.,0.025,0.05,0.075,
0.1,0.125,0.15,0.175,0.2,0.225,0.25,0.275,0.3,0.325,0.35,0.375,0.4,0.425,
0.45,0.475,0.5,0.525,0.55,0.575,0.6,0.625,0.65,0.675,0.7,0.725,0.75,0.775,
0.8,0.825,0.85,0.875,0.9,0.925,0.95,0.975,1.),.UNSPECIFIED.)
GEOMETRIC_REPRESENTATION_ITEM()
RATIONAL_B_SPLINE_SURFACE(((1.,0.996917333733128,1.,0.996917333733128,1.,
0.996917333733128,1.,0.996917333733128,1.,0.996917333733128,1.,0.996917333733128,
1.,0.996917333733128,1.,0.996917333733128,1.,0.996917333733128,1.,0.996917333733128,
1.,0.996917333733128,1.,0.996917333733128,1.,0.996917333733128,1.,0.996917333733128,
1.,0.996917333733128,1.,0.996917333733128,1.,0.996917333733128,1.,0.996917333733128,
1.,0.996917333733128,1.,0.996917333733128,1.,0.996917333733128,1.,0.996917333733128,
1.,0.996917333733128,1.,0.996917333733128,1.,0.996917333733128,1.,0.996917333733128,
1.,0.996917333733128,1.,0.996917333733128,1.,0.996917333733128,1.,0.996917333733128,
1.,0.996917333733128,1.,0.996917333733128,1.,0.996917333733128,1.,0.996917333733128,
1.,0.996917333733128,1.,0.996917333733128,1.,0.996917333733128,1.,0.996917333733128,
1.,0.996917333733128,1.,0.996917333733128,1.),(1.,0.996917333733128,1.,
0.996917333733128,1.,0.996917333733128,1.,0.996917333733128,1.,0.996917333733128,
1.,0.996917333733128,1.,0.996917333733128,1.,0.996917333733128,1.,0.996917333733128,
1.,0.996917333733128,1.,0.996917333733128,1.,0.996917333733128,1.,0.996917333733128,
1.,0.996917333733128,1.,0.996917333733128,1.,0.996917333733128,1.,0.996917333733128,
1.,0.996917333733128,1.,0.996917333733128,1.,0.996917333733128,1.,0.996917333733128,
1.,0.996917333733128,1.,0.996917333733128,1.,0.996917333733128,1.,0.996917333733128,
1.,0.996917333733128,1.,0.996917333733128,1.,0.996917333733128,1.,0.996917333733128,
1.,0.996917333733128,1.,0.996917333733128,1.,0.996917333733128,1.,0.996917333733128,
1.,0.996917333733128,1.,0.996917333733128,1.,0.996917333733128,1.,0.996917333733128,
1.,0.996917333733128,1.,0.996917333733128,1.,0.996917333733128,1.)))
REPRESENTATION_ITEM('')
SURFACE()
);
#4049=(
BOUNDED_SURFACE()
B_SPLINE_SURFACE(1,2,((#272391,#272392,#272393,#272394,#272395,#272396,
#272397,#272398,#272399,#272400,#272401,#272402,#272403,#272404,#272405,
#272406,#272407,#272408,#272409,#272410,#272411,#272412,#272413,#272414,
#272415,#272416,#272417,#272418,#272419,#272420,#272421,#272422,#272423,
#272424,#272425,#272426,#272427,#272428,#272429,#272430,#272431,#272432,
#272433,#272434,#272435,#272436,#272437,#272438,#272439,#272440,#272441,
#272442,#272443,#272444,#272445,#272446,#272447,#272448,#272449,#272450,
#272451,#272452,#272453,#272454,#272455,#272456,#272457,#272458,#272459,
#272460,#272461,#272462,#272463,#272464,#272465,#272466,#272467,#272468,
#272469,#272470,#272471),(#272472,#272473,#272474,#272475,#272476,#272477,
#272478,#272479,#272480,#272481,#272482,#272483,#272484,#272485,#272486,
#272487,#272488,#272489,#272490,#272491,#272492,#272493,#272494,#272495,
#272496,#272497,#272498,#272499,#272500,#272501,#272502,#272503,#272504,
#272505,#272506,#272507,#272508,#272509,#272510,#272511,#272512,#272513,
#272514,#272515,#272516,#272517,#272518,#272519,#272520,#272521,#272522,
#272523,#272524,#272525,#272526,#272527,#272528,#272529,#272530,#272531,
#272532,#272533,#272534,#272535,#272536,#272537,#272538,#272539,#272540,
#272541,#272542,#272543,#272544,#272545,#272546,#272547,#272548,#272549,
#272550,#272551,#272552)),.UNSPECIFIED.,.F.,.F.,.F.)
B_SPLINE_SURFACE_WITH_KNOTS((2,2),(3,2,2,2,2,2,2,2,2,2,2,2,2,2,2,2,2,2,
2,2,2,2,2,2,2,2,2,2,2,2,2,2,2,2,2,2,2,2,2,2,3),(0.,1.),(0.,0.025,0.05,0.075,
0.1,0.125,0.15,0.175,0.2,0.225,0.25,0.275,0.3,0.325,0.35,0.375,0.4,0.425,
0.45,0.475,0.5,0.525,0.55,0.575,0.6,0.625,0.65,0.675,0.7,0.725,0.75,0.775,
0.8,0.825,0.85,0.875,0.9,0.925,0.95,0.975,1.),.UNSPECIFIED.)
GEOMETRIC_REPRESENTATION_ITEM()
RATIONAL_B_SPLINE_SURFACE(((1.,0.996917333733128,1.,0.996917333733128,1.,
0.996917333733128,1.,0.996917333733128,1.,0.996917333733128,1.,0.996917333733128,
1.,0.996917333733128,1.,0.996917333733128,1.,0.996917333733128,1.,0.996917333733128,
1.,0.996917333733128,1.,0.996917333733128,1.,0.996917333733128,1.,0.996917333733128,
1.,0.996917333733128,1.,0.996917333733128,1.,0.996917333733128,1.,0.996917333733128,
1.,0.996917333733128,1.,0.996917333733128,1.,0.996917333733128,1.,0.996917333733128,
1.,0.996917333733128,1.,0.996917333733128,1.,0.996917333733128,1.,0.996917333733128,
1.,0.996917333733128,1.,0.996917333733128,1.,0.996917333733128,1.,0.996917333733128,
1.,0.996917333733128,1.,0.996917333733128,1.,0.996917333733128,1.,0.996917333733128,
1.,0.996917333733128,1.,0.996917333733128,1.,0.996917333733128,1.,0.996917333733128,
1.,0.996917333733128,1.,0.996917333733128,1.),(1.,0.996917333733128,1.,
0.996917333733128,1.,0.996917333733128,1.,0.996917333733128,1.,0.996917333733128,
1.,0.996917333733128,1.,0.996917333733128,1.,0.996917333733128,1.,0.996917333733128,
1.,0.996917333733128,1.,0.996917333733128,1.,0.996917333733128,1.,0.996917333733128,
1.,0.996917333733128,1.,0.996917333733128,1.,0.996917333733128,1.,0.996917333733128,
1.,0.996917333733128,1.,0.996917333733128,1.,0.996917333733128,1.,0.996917333733128,
1.,0.996917333733128,1.,0.996917333733128,1.,0.996917333733128,1.,0.996917333733128,
1.,0.996917333733128,1.,0.996917333733128,1.,0.996917333733128,1.,0.996917333733128,
1.,0.996917333733128,1.,0.996917333733128,1.,0.996917333733128,1.,0.996917333733128,
1.,0.996917333733128,1.,0.996917333733128,1.,0.996917333733128,1.,0.996917333733128,
1.,0.996917333733128,1.,0.996917333733128,1.,0.996917333733128,1.)))
REPRESENTATION_ITEM('')
SURFACE()
);
#4050=(
BOUNDED_SURFACE()
B_SPLINE_SURFACE(1,2,((#272554,#272555,#272556,#272557,#272558,#272559,
#272560,#272561,#272562,#272563,#272564,#272565,#272566,#272567,#272568,
#272569,#272570,#272571,#272572,#272573,#272574,#272575,#272576,#272577,
#272578,#272579,#272580,#272581,#272582,#272583,#272584,#272585,#272586,
#272587,#272588,#272589,#272590,#272591,#272592,#272593,#272594,#272595,
#272596,#272597,#272598,#272599,#272600,#272601,#272602,#272603,#272604,
#272605,#272606,#272607,#272608,#272609,#272610,#272611,#272612,#272613,
#272614,#272615,#272616,#272617,#272618,#272619,#272620,#272621,#272622,
#272623,#272624,#272625,#272626,#272627,#272628,#272629,#272630,#272631,
#272632,#272633,#272634),(#272635,#272636,#272637,#272638,#272639,#272640,
#272641,#272642,#272643,#272644,#272645,#272646,#272647,#272648,#272649,
#272650,#272651,#272652,#272653,#272654,#272655,#272656,#272657,#272658,
#272659,#272660,#272661,#272662,#272663,#272664,#272665,#272666,#272667,
#272668,#272669,#272670,#272671,#272672,#272673,#272674,#272675,#272676,
#272677,#272678,#272679,#272680,#272681,#272682,#272683,#272684,#272685,
#272686,#272687,#272688,#272689,#272690,#272691,#272692,#272693,#272694,
#272695,#272696,#272697,#272698,#272699,#272700,#272701,#272702,#272703,
#272704,#272705,#272706,#272707,#272708,#272709,#272710,#272711,#272712,
#272713,#272714,#272715)),.UNSPECIFIED.,.F.,.F.,.F.)
B_SPLINE_SURFACE_WITH_KNOTS((2,2),(3,2,2,2,2,2,2,2,2,2,2,2,2,2,2,2,2,2,
2,2,2,2,2,2,2,2,2,2,2,2,2,2,2,2,2,2,2,2,2,2,3),(0.,1.),(0.,0.025,0.05,0.075,
0.1,0.125,0.15,0.175,0.2,0.225,0.25,0.275,0.3,0.325,0.35,0.375,0.4,0.425,
0.45,0.475,0.5,0.525,0.55,0.575,0.6,0.625,0.65,0.675,0.7,0.725,0.75,0.775,
0.8,0.825,0.85,0.875,0.9,0.925,0.95,0.975,1.),.UNSPECIFIED.)
GEOMETRIC_REPRESENTATION_ITEM()
RATIONAL_B_SPLINE_SURFACE(((1.,0.996917333733128,1.,0.996917333733128,1.,
0.996917333733128,1.,0.996917333733128,1.,0.996917333733128,1.,0.996917333733128,
1.,0.996917333733128,1.,0.996917333733128,1.,0.996917333733128,1.,0.996917333733128,
1.,0.996917333733128,1.,0.996917333733128,1.,0.996917333733128,1.,0.996917333733128,
1.,0.996917333733128,1.,0.996917333733128,1.,0.996917333733128,1.,0.996917333733128,
1.,0.996917333733128,1.,0.996917333733128,1.,0.996917333733128,1.,0.996917333733128,
1.,0.996917333733128,1.,0.996917333733128,1.,0.996917333733128,1.,0.996917333733128,
1.,0.996917333733128,1.,0.996917333733128,1.,0.996917333733128,1.,0.996917333733128,
1.,0.996917333733128,1.,0.996917333733128,1.,0.996917333733128,1.,0.996917333733128,
1.,0.996917333733128,1.,0.996917333733128,1.,0.996917333733128,1.,0.996917333733128,
1.,0.996917333733128,1.,0.996917333733128,1.),(1.,0.996917333733128,1.,
0.996917333733128,1.,0.996917333733128,1.,0.996917333733128,1.,0.996917333733128,
1.,0.996917333733128,1.,0.996917333733128,1.,0.996917333733128,1.,0.996917333733128,
1.,0.996917333733128,1.,0.996917333733128,1.,0.996917333733128,1.,0.996917333733128,
1.,0.996917333733128,1.,0.996917333733128,1.,0.996917333733128,1.,0.996917333733128,
1.,0.996917333733128,1.,0.996917333733128,1.,0.996917333733128,1.,0.996917333733128,
1.,0.996917333733128,1.,0.996917333733128,1.,0.996917333733128,1.,0.996917333733128,
1.,0.996917333733128,1.,0.996917333733128,1.,0.996917333733128,1.,0.996917333733128,
1.,0.996917333733128,1.,0.996917333733128,1.,0.996917333733128,1.,0.996917333733128,
1.,0.996917333733128,1.,0.996917333733128,1.,0.996917333733128,1.,0.996917333733128,
1.,0.996917333733128,1.,0.996917333733128,1.,0.996917333733128,1.)))
REPRESENTATION_ITEM('')
SURFACE()
);
#4051=(
BOUNDED_SURFACE()
B_SPLINE_SURFACE(1,2,((#272732,#272733,#272734,#272735,#272736,#272737,
#272738,#272739,#272740,#272741,#272742,#272743,#272744,#272745,#272746,
#272747,#272748,#272749,#272750,#272751,#272752,#272753,#272754,#272755,
#272756,#272757,#272758,#272759,#272760,#272761,#272762,#272763,#272764,
#272765,#272766,#272767,#272768,#272769,#272770,#272771,#272772,#272773,
#272774,#272775,#272776,#272777,#272778,#272779,#272780,#272781,#272782,
#272783,#272784,#272785,#272786,#272787,#272788,#272789,#272790,#272791,
#272792,#272793,#272794,#272795,#272796,#272797,#272798,#272799,#272800,
#272801,#272802,#272803,#272804,#272805,#272806,#272807,#272808,#272809,
#272810,#272811,#272812),(#272813,#272814,#272815,#272816,#272817,#272818,
#272819,#272820,#272821,#272822,#272823,#272824,#272825,#272826,#272827,
#272828,#272829,#272830,#272831,#272832,#272833,#272834,#272835,#272836,
#272837,#272838,#272839,#272840,#272841,#272842,#272843,#272844,#272845,
#272846,#272847,#272848,#272849,#272850,#272851,#272852,#272853,#272854,
#272855,#272856,#272857,#272858,#272859,#272860,#272861,#272862,#272863,
#272864,#272865,#272866,#272867,#272868,#272869,#272870,#272871,#272872,
#272873,#272874,#272875,#272876,#272877,#272878,#272879,#272880,#272881,
#272882,#272883,#272884,#272885,#272886,#272887,#272888,#272889,#272890,
#272891,#272892,#272893)),.UNSPECIFIED.,.F.,.F.,.F.)
B_SPLINE_SURFACE_WITH_KNOTS((2,2),(3,2,2,2,2,2,2,2,2,2,2,2,2,2,2,2,2,2,
2,2,2,2,2,2,2,2,2,2,2,2,2,2,2,2,2,2,2,2,2,2,3),(0.,1.),(0.,0.025,0.05,0.075,
0.1,0.125,0.15,0.175,0.2,0.225,0.25,0.275,0.3,0.325,0.35,0.375,0.4,0.425,
0.45,0.475,0.5,0.525,0.55,0.575,0.6,0.625,0.65,0.675,0.7,0.725,0.75,0.775,
0.8,0.825,0.85,0.875,0.9,0.925,0.95,0.975,1.),.UNSPECIFIED.)
GEOMETRIC_REPRESENTATION_ITEM()
RATIONAL_B_SPLINE_SURFACE(((1.,0.996917333733128,1.,0.996917333733128,1.,
0.996917333733128,1.,0.996917333733128,1.,0.996917333733128,1.,0.996917333733128,
1.,0.996917333733128,1.,0.996917333733128,1.,0.996917333733128,1.,0.996917333733128,
1.,0.996917333733128,1.,0.996917333733128,1.,0.996917333733128,1.,0.996917333733128,
1.,0.996917333733128,1.,0.996917333733128,1.,0.996917333733128,1.,0.996917333733128,
1.,0.996917333733128,1.,0.996917333733128,1.,0.996917333733128,1.,0.996917333733128,
1.,0.996917333733128,1.,0.996917333733128,1.,0.996917333733128,1.,0.996917333733128,
1.,0.996917333733128,1.,0.996917333733128,1.,0.996917333733128,1.,0.996917333733128,
1.,0.996917333733128,1.,0.996917333733128,1.,0.996917333733128,1.,0.996917333733128,
1.,0.996917333733128,1.,0.996917333733128,1.,0.996917333733128,1.,0.996917333733128,
1.,0.996917333733128,1.,0.996917333733128,1.),(1.,0.996917333733128,1.,
0.996917333733128,1.,0.996917333733128,1.,0.996917333733128,1.,0.996917333733128,
1.,0.996917333733128,1.,0.996917333733128,1.,0.996917333733128,1.,0.996917333733128,
1.,0.996917333733128,1.,0.996917333733128,1.,0.996917333733128,1.,0.996917333733128,
1.,0.996917333733128,1.,0.996917333733128,1.,0.996917333733128,1.,0.996917333733128,
1.,0.996917333733128,1.,0.996917333733128,1.,0.996917333733128,1.,0.996917333733128,
1.,0.996917333733128,1.,0.996917333733128,1.,0.996917333733128,1.,0.996917333733128,
1.,0.996917333733128,1.,0.996917333733128,1.,0.996917333733128,1.,0.996917333733128,
1.,0.996917333733128,1.,0.996917333733128,1.,0.996917333733128,1.,0.996917333733128,
1.,0.996917333733128,1.,0.996917333733128,1.,0.996917333733128,1.,0.996917333733128,
1.,0.996917333733128,1.,0.996917333733128,1.,0.996917333733128,1.)))
REPRESENTATION_ITEM('')
SURFACE()
);
#4052=(
BOUNDED_SURFACE()
B_SPLINE_SURFACE(1,2,((#272895,#272896,#272897,#272898,#272899,#272900,
#272901,#272902,#272903,#272904,#272905,#272906,#272907,#272908,#272909,
#272910,#272911,#272912,#272913,#272914,#272915,#272916,#272917,#272918,
#272919,#272920,#272921,#272922,#272923,#272924,#272925,#272926,#272927,
#272928,#272929,#272930,#272931,#272932,#272933,#272934,#272935,#272936,
#272937,#272938,#272939,#272940,#272941,#272942,#272943,#272944,#272945,
#272946,#272947,#272948,#272949,#272950,#272951,#272952,#272953,#272954,
#272955,#272956,#272957,#272958,#272959,#272960,#272961,#272962,#272963,
#272964,#272965,#272966,#272967,#272968,#272969,#272970,#272971,#272972,
#272973,#272974,#272975),(#272976,#272977,#272978,#272979,#272980,#272981,
#272982,#272983,#272984,#272985,#272986,#272987,#272988,#272989,#272990,
#272991,#272992,#272993,#272994,#272995,#272996,#272997,#272998,#272999,
#273000,#273001,#273002,#273003,#273004,#273005,#273006,#273007,#273008,
#273009,#273010,#273011,#273012,#273013,#273014,#273015,#273016,#273017,
#273018,#273019,#273020,#273021,#273022,#273023,#273024,#273025,#273026,
#273027,#273028,#273029,#273030,#273031,#273032,#273033,#273034,#273035,
#273036,#273037,#273038,#273039,#273040,#273041,#273042,#273043,#273044,
#273045,#273046,#273047,#273048,#273049,#273050,#273051,#273052,#273053,
#273054,#273055,#273056)),.UNSPECIFIED.,.F.,.F.,.F.)
B_SPLINE_SURFACE_WITH_KNOTS((2,2),(3,2,2,2,2,2,2,2,2,2,2,2,2,2,2,2,2,2,
2,2,2,2,2,2,2,2,2,2,2,2,2,2,2,2,2,2,2,2,2,2,3),(0.,1.),(0.,0.025,0.05,0.075,
0.1,0.125,0.15,0.175,0.2,0.225,0.25,0.275,0.3,0.325,0.35,0.375,0.4,0.425,
0.45,0.475,0.5,0.525,0.55,0.575,0.6,0.625,0.65,0.675,0.7,0.725,0.75,0.775,
0.8,0.825,0.85,0.875,0.9,0.925,0.95,0.975,1.),.UNSPECIFIED.)
GEOMETRIC_REPRESENTATION_ITEM()
RATIONAL_B_SPLINE_SURFACE(((1.,0.996917333733128,1.,0.996917333733128,1.,
0.996917333733128,1.,0.996917333733128,1.,0.996917333733128,1.,0.996917333733128,
1.,0.996917333733128,1.,0.996917333733128,1.,0.996917333733128,1.,0.996917333733128,
1.,0.996917333733128,1.,0.996917333733128,1.,0.996917333733128,1.,0.996917333733128,
1.,0.996917333733128,1.,0.996917333733128,1.,0.996917333733128,1.,0.996917333733128,
1.,0.996917333733128,1.,0.996917333733128,1.,0.996917333733128,1.,0.996917333733128,
1.,0.996917333733128,1.,0.996917333733128,1.,0.996917333733128,1.,0.996917333733128,
1.,0.996917333733128,1.,0.996917333733128,1.,0.996917333733128,1.,0.996917333733128,
1.,0.996917333733128,1.,0.996917333733128,1.,0.996917333733128,1.,0.996917333733128,
1.,0.996917333733128,1.,0.996917333733128,1.,0.996917333733128,1.,0.996917333733128,
1.,0.996917333733128,1.,0.996917333733128,1.),(1.,0.996917333733128,1.,
0.996917333733128,1.,0.996917333733128,1.,0.996917333733128,1.,0.996917333733128,
1.,0.996917333733128,1.,0.996917333733128,1.,0.996917333733128,1.,0.996917333733128,
1.,0.996917333733128,1.,0.996917333733128,1.,0.996917333733128,1.,0.996917333733128,
1.,0.996917333733128,1.,0.996917333733128,1.,0.996917333733128,1.,0.996917333733128,
1.,0.996917333733128,1.,0.996917333733128,1.,0.996917333733128,1.,0.996917333733128,
1.,0.996917333733128,1.,0.996917333733128,1.,0.996917333733128,1.,0.996917333733128,
1.,0.996917333733128,1.,0.996917333733128,1.,0.996917333733128,1.,0.996917333733128,
1.,0.996917333733128,1.,0.996917333733128,1.,0.996917333733128,1.,0.996917333733128,
1.,0.996917333733128,1.,0.996917333733128,1.,0.996917333733128,1.,0.996917333733128,
1.,0.996917333733128,1.,0.996917333733128,1.,0.996917333733128,1.)))
REPRESENTATION_ITEM('')
SURFACE()
);
#4053=(
BOUNDED_SURFACE()
B_SPLINE_SURFACE(1,2,((#273073,#273074,#273075,#273076,#273077,#273078,
#273079,#273080,#273081,#273082,#273083,#273084,#273085,#273086,#273087,
#273088,#273089,#273090,#273091,#273092,#273093,#273094,#273095,#273096,
#273097,#273098,#273099,#273100,#273101,#273102,#273103,#273104,#273105,
#273106,#273107,#273108,#273109,#273110,#273111,#273112,#273113,#273114,
#273115,#273116,#273117,#273118,#273119,#273120,#273121,#273122,#273123,
#273124,#273125,#273126,#273127,#273128,#273129,#273130,#273131,#273132,
#273133,#273134,#273135,#273136,#273137,#273138,#273139,#273140,#273141,
#273142,#273143,#273144,#273145,#273146,#273147,#273148,#273149,#273150,
#273151,#273152,#273153),(#273154,#273155,#273156,#273157,#273158,#273159,
#273160,#273161,#273162,#273163,#273164,#273165,#273166,#273167,#273168,
#273169,#273170,#273171,#273172,#273173,#273174,#273175,#273176,#273177,
#273178,#273179,#273180,#273181,#273182,#273183,#273184,#273185,#273186,
#273187,#273188,#273189,#273190,#273191,#273192,#273193,#273194,#273195,
#273196,#273197,#273198,#273199,#273200,#273201,#273202,#273203,#273204,
#273205,#273206,#273207,#273208,#273209,#273210,#273211,#273212,#273213,
#273214,#273215,#273216,#273217,#273218,#273219,#273220,#273221,#273222,
#273223,#273224,#273225,#273226,#273227,#273228,#273229,#273230,#273231,
#273232,#273233,#273234)),.UNSPECIFIED.,.F.,.F.,.F.)
B_SPLINE_SURFACE_WITH_KNOTS((2,2),(3,2,2,2,2,2,2,2,2,2,2,2,2,2,2,2,2,2,
2,2,2,2,2,2,2,2,2,2,2,2,2,2,2,2,2,2,2,2,2,2,3),(0.,1.),(0.,0.025,0.05,0.075,
0.1,0.125,0.15,0.175,0.2,0.225,0.25,0.275,0.3,0.325,0.35,0.375,0.4,0.425,
0.45,0.475,0.5,0.525,0.55,0.575,0.6,0.625,0.65,0.675,0.7,0.725,0.75,0.775,
0.8,0.825,0.85,0.875,0.9,0.925,0.95,0.975,1.),.UNSPECIFIED.)
GEOMETRIC_REPRESENTATION_ITEM()
RATIONAL_B_SPLINE_SURFACE(((1.,0.996917333733128,1.,0.996917333733128,1.,
0.996917333733128,1.,0.996917333733128,1.,0.996917333733128,1.,0.996917333733128,
1.,0.996917333733128,1.,0.996917333733128,1.,0.996917333733128,1.,0.996917333733128,
1.,0.996917333733128,1.,0.996917333733128,1.,0.996917333733128,1.,0.996917333733128,
1.,0.996917333733128,1.,0.996917333733128,1.,0.996917333733128,1.,0.996917333733128,
1.,0.996917333733128,1.,0.996917333733128,1.,0.996917333733128,1.,0.996917333733128,
1.,0.996917333733128,1.,0.996917333733128,1.,0.996917333733128,1.,0.996917333733128,
1.,0.996917333733128,1.,0.996917333733128,1.,0.996917333733128,1.,0.996917333733128,
1.,0.996917333733128,1.,0.996917333733128,1.,0.996917333733128,1.,0.996917333733128,
1.,0.996917333733128,1.,0.996917333733128,1.,0.996917333733128,1.,0.996917333733128,
1.,0.996917333733128,1.,0.996917333733128,1.),(1.,0.996917333733128,1.,
0.996917333733128,1.,0.996917333733128,1.,0.996917333733128,1.,0.996917333733128,
1.,0.996917333733128,1.,0.996917333733128,1.,0.996917333733128,1.,0.996917333733128,
1.,0.996917333733128,1.,0.996917333733128,1.,0.996917333733128,1.,0.996917333733128,
1.,0.996917333733128,1.,0.996917333733128,1.,0.996917333733128,1.,0.996917333733128,
1.,0.996917333733128,1.,0.996917333733128,1.,0.996917333733128,1.,0.996917333733128,
1.,0.996917333733128,1.,0.996917333733128,1.,0.996917333733128,1.,0.996917333733128,
1.,0.996917333733128,1.,0.996917333733128,1.,0.996917333733128,1.,0.996917333733128,
1.,0.996917333733128,1.,0.996917333733128,1.,0.996917333733128,1.,0.996917333733128,
1.,0.996917333733128,1.,0.996917333733128,1.,0.996917333733128,1.,0.996917333733128,
1.,0.996917333733128,1.,0.996917333733128,1.,0.996917333733128,1.)))
REPRESENTATION_ITEM('')
SURFACE()
);
#4054=(
BOUNDED_SURFACE()
B_SPLINE_SURFACE(1,2,((#273236,#273237,#273238,#273239,#273240,#273241,
#273242,#273243,#273244,#273245,#273246,#273247,#273248,#273249,#273250,
#273251,#273252,#273253,#273254,#273255,#273256,#273257,#273258,#273259,
#273260,#273261,#273262,#273263,#273264,#273265,#273266,#273267,#273268,
#273269,#273270,#273271,#273272,#273273,#273274,#273275,#273276,#273277,
#273278,#273279,#273280,#273281,#273282,#273283,#273284,#273285,#273286,
#273287,#273288,#273289,#273290,#273291,#273292,#273293,#273294,#273295,
#273296,#273297,#273298,#273299,#273300,#273301,#273302,#273303,#273304,
#273305,#273306,#273307,#273308,#273309,#273310,#273311,#273312,#273313,
#273314,#273315,#273316),(#273317,#273318,#273319,#273320,#273321,#273322,
#273323,#273324,#273325,#273326,#273327,#273328,#273329,#273330,#273331,
#273332,#273333,#273334,#273335,#273336,#273337,#273338,#273339,#273340,
#273341,#273342,#273343,#273344,#273345,#273346,#273347,#273348,#273349,
#273350,#273351,#273352,#273353,#273354,#273355,#273356,#273357,#273358,
#273359,#273360,#273361,#273362,#273363,#273364,#273365,#273366,#273367,
#273368,#273369,#273370,#273371,#273372,#273373,#273374,#273375,#273376,
#273377,#273378,#273379,#273380,#273381,#273382,#273383,#273384,#273385,
#273386,#273387,#273388,#273389,#273390,#273391,#273392,#273393,#273394,
#273395,#273396,#273397)),.UNSPECIFIED.,.F.,.F.,.F.)
B_SPLINE_SURFACE_WITH_KNOTS((2,2),(3,2,2,2,2,2,2,2,2,2,2,2,2,2,2,2,2,2,
2,2,2,2,2,2,2,2,2,2,2,2,2,2,2,2,2,2,2,2,2,2,3),(0.,1.),(0.,0.025,0.05,0.075,
0.1,0.125,0.15,0.175,0.2,0.225,0.25,0.275,0.3,0.325,0.35,0.375,0.4,0.425,
0.45,0.475,0.5,0.525,0.55,0.575,0.6,0.625,0.65,0.675,0.7,0.725,0.75,0.775,
0.8,0.825,0.85,0.875,0.9,0.925,0.95,0.975,1.),.UNSPECIFIED.)
GEOMETRIC_REPRESENTATION_ITEM()
RATIONAL_B_SPLINE_SURFACE(((1.,0.996917333733128,1.,0.996917333733128,1.,
0.996917333733128,1.,0.996917333733128,1.,0.996917333733128,1.,0.996917333733128,
1.,0.996917333733128,1.,0.996917333733128,1.,0.996917333733128,1.,0.996917333733128,
1.,0.996917333733128,1.,0.996917333733128,1.,0.996917333733128,1.,0.996917333733128,
1.,0.996917333733128,1.,0.996917333733128,1.,0.996917333733128,1.,0.996917333733128,
1.,0.996917333733128,1.,0.996917333733128,1.,0.996917333733128,1.,0.996917333733128,
1.,0.996917333733128,1.,0.996917333733128,1.,0.996917333733128,1.,0.996917333733128,
1.,0.996917333733128,1.,0.996917333733128,1.,0.996917333733128,1.,0.996917333733128,
1.,0.996917333733128,1.,0.996917333733128,1.,0.996917333733128,1.,0.996917333733128,
1.,0.996917333733128,1.,0.996917333733128,1.,0.996917333733128,1.,0.996917333733128,
1.,0.996917333733128,1.,0.996917333733128,1.),(1.,0.996917333733128,1.,
0.996917333733128,1.,0.996917333733128,1.,0.996917333733128,1.,0.996917333733128,
1.,0.996917333733128,1.,0.996917333733128,1.,0.996917333733128,1.,0.996917333733128,
1.,0.996917333733128,1.,0.996917333733128,1.,0.996917333733128,1.,0.996917333733128,
1.,0.996917333733128,1.,0.996917333733128,1.,0.996917333733128,1.,0.996917333733128,
1.,0.996917333733128,1.,0.996917333733128,1.,0.996917333733128,1.,0.996917333733128,
1.,0.996917333733128,1.,0.996917333733128,1.,0.996917333733128,1.,0.996917333733128,
1.,0.996917333733128,1.,0.996917333733128,1.,0.996917333733128,1.,0.996917333733128,
1.,0.996917333733128,1.,0.996917333733128,1.,0.996917333733128,1.,0.996917333733128,
1.,0.996917333733128,1.,0.996917333733128,1.,0.996917333733128,1.,0.996917333733128,
1.,0.996917333733128,1.,0.996917333733128,1.,0.996917333733128,1.)))
REPRESENTATION_ITEM('')
SURFACE()
);
#4055=(
BOUNDED_SURFACE()
B_SPLINE_SURFACE(1,2,((#273414,#273415,#273416,#273417,#273418,#273419,
#273420,#273421,#273422,#273423,#273424,#273425,#273426,#273427,#273428,
#273429,#273430,#273431,#273432,#273433,#273434,#273435,#273436,#273437,
#273438,#273439,#273440,#273441,#273442,#273443,#273444,#273445,#273446,
#273447,#273448,#273449,#273450,#273451,#273452,#273453,#273454,#273455,
#273456,#273457,#273458,#273459,#273460,#273461,#273462,#273463,#273464,
#273465,#273466,#273467,#273468,#273469,#273470,#273471,#273472,#273473,
#273474,#273475,#273476,#273477,#273478,#273479,#273480,#273481,#273482,
#273483,#273484,#273485,#273486,#273487,#273488,#273489,#273490,#273491,
#273492,#273493,#273494),(#273495,#273496,#273497,#273498,#273499,#273500,
#273501,#273502,#273503,#273504,#273505,#273506,#273507,#273508,#273509,
#273510,#273511,#273512,#273513,#273514,#273515,#273516,#273517,#273518,
#273519,#273520,#273521,#273522,#273523,#273524,#273525,#273526,#273527,
#273528,#273529,#273530,#273531,#273532,#273533,#273534,#273535,#273536,
#273537,#273538,#273539,#273540,#273541,#273542,#273543,#273544,#273545,
#273546,#273547,#273548,#273549,#273550,#273551,#273552,#273553,#273554,
#273555,#273556,#273557,#273558,#273559,#273560,#273561,#273562,#273563,
#273564,#273565,#273566,#273567,#273568,#273569,#273570,#273571,#273572,
#273573,#273574,#273575)),.UNSPECIFIED.,.F.,.F.,.F.)
B_SPLINE_SURFACE_WITH_KNOTS((2,2),(3,2,2,2,2,2,2,2,2,2,2,2,2,2,2,2,2,2,
2,2,2,2,2,2,2,2,2,2,2,2,2,2,2,2,2,2,2,2,2,2,3),(0.,1.),(0.,0.025,0.05,0.075,
0.1,0.125,0.15,0.175,0.2,0.225,0.25,0.275,0.3,0.325,0.35,0.375,0.4,0.425,
0.45,0.475,0.5,0.525,0.55,0.575,0.6,0.625,0.65,0.675,0.7,0.725,0.75,0.775,
0.8,0.825,0.85,0.875,0.9,0.925,0.95,0.975,1.),.UNSPECIFIED.)
GEOMETRIC_REPRESENTATION_ITEM()
RATIONAL_B_SPLINE_SURFACE(((1.,0.996917333733128,1.,0.996917333733128,1.,
0.996917333733128,1.,0.996917333733128,1.,0.996917333733128,1.,0.996917333733128,
1.,0.996917333733128,1.,0.996917333733128,1.,0.996917333733128,1.,0.996917333733128,
1.,0.996917333733128,1.,0.996917333733128,1.,0.996917333733128,1.,0.996917333733128,
1.,0.996917333733128,1.,0.996917333733128,1.,0.996917333733128,1.,0.996917333733128,
1.,0.996917333733128,1.,0.996917333733128,1.,0.996917333733128,1.,0.996917333733128,
1.,0.996917333733128,1.,0.996917333733128,1.,0.996917333733128,1.,0.996917333733128,
1.,0.996917333733128,1.,0.996917333733128,1.,0.996917333733128,1.,0.996917333733128,
1.,0.996917333733128,1.,0.996917333733128,1.,0.996917333733128,1.,0.996917333733128,
1.,0.996917333733128,1.,0.996917333733128,1.,0.996917333733128,1.,0.996917333733128,
1.,0.996917333733128,1.,0.996917333733128,1.),(1.,0.996917333733128,1.,
0.996917333733128,1.,0.996917333733128,1.,0.996917333733128,1.,0.996917333733128,
1.,0.996917333733128,1.,0.996917333733128,1.,0.996917333733128,1.,0.996917333733128,
1.,0.996917333733128,1.,0.996917333733128,1.,0.996917333733128,1.,0.996917333733128,
1.,0.996917333733128,1.,0.996917333733128,1.,0.996917333733128,1.,0.996917333733128,
1.,0.996917333733128,1.,0.996917333733128,1.,0.996917333733128,1.,0.996917333733128,
1.,0.996917333733128,1.,0.996917333733128,1.,0.996917333733128,1.,0.996917333733128,
1.,0.996917333733128,1.,0.996917333733128,1.,0.996917333733128,1.,0.996917333733128,
1.,0.996917333733128,1.,0.996917333733128,1.,0.996917333733128,1.,0.996917333733128,
1.,0.996917333733128,1.,0.996917333733128,1.,0.996917333733128,1.,0.996917333733128,
1.,0.996917333733128,1.,0.996917333733128,1.,0.996917333733128,1.)))
REPRESENTATION_ITEM('')
SURFACE()
);
#4056=(
BOUNDED_SURFACE()
B_SPLINE_SURFACE(1,2,((#273577,#273578,#273579,#273580,#273581,#273582,
#273583,#273584,#273585,#273586,#273587,#273588,#273589,#273590,#273591,
#273592,#273593,#273594,#273595,#273596,#273597,#273598,#273599,#273600,
#273601,#273602,#273603,#273604,#273605,#273606,#273607,#273608,#273609,
#273610,#273611,#273612,#273613,#273614,#273615,#273616,#273617,#273618,
#273619,#273620,#273621,#273622,#273623,#273624,#273625,#273626,#273627,
#273628,#273629,#273630,#273631,#273632,#273633,#273634,#273635,#273636,
#273637,#273638,#273639,#273640,#273641,#273642,#273643,#273644,#273645,
#273646,#273647,#273648,#273649,#273650,#273651,#273652,#273653,#273654,
#273655,#273656,#273657),(#273658,#273659,#273660,#273661,#273662,#273663,
#273664,#273665,#273666,#273667,#273668,#273669,#273670,#273671,#273672,
#273673,#273674,#273675,#273676,#273677,#273678,#273679,#273680,#273681,
#273682,#273683,#273684,#273685,#273686,#273687,#273688,#273689,#273690,
#273691,#273692,#273693,#273694,#273695,#273696,#273697,#273698,#273699,
#273700,#273701,#273702,#273703,#273704,#273705,#273706,#273707,#273708,
#273709,#273710,#273711,#273712,#273713,#273714,#273715,#273716,#273717,
#273718,#273719,#273720,#273721,#273722,#273723,#273724,#273725,#273726,
#273727,#273728,#273729,#273730,#273731,#273732,#273733,#273734,#273735,
#273736,#273737,#273738)),.UNSPECIFIED.,.F.,.F.,.F.)
B_SPLINE_SURFACE_WITH_KNOTS((2,2),(3,2,2,2,2,2,2,2,2,2,2,2,2,2,2,2,2,2,
2,2,2,2,2,2,2,2,2,2,2,2,2,2,2,2,2,2,2,2,2,2,3),(0.,1.),(0.,0.025,0.05,0.075,
0.1,0.125,0.15,0.175,0.2,0.225,0.25,0.275,0.3,0.325,0.35,0.375,0.4,0.425,
0.45,0.475,0.5,0.525,0.55,0.575,0.6,0.625,0.65,0.675,0.7,0.725,0.75,0.775,
0.8,0.825,0.85,0.875,0.9,0.925,0.95,0.975,1.),.UNSPECIFIED.)
GEOMETRIC_REPRESENTATION_ITEM()
RATIONAL_B_SPLINE_SURFACE(((1.,0.996917333733128,1.,0.996917333733128,1.,
0.996917333733128,1.,0.996917333733128,1.,0.996917333733128,1.,0.996917333733128,
1.,0.996917333733128,1.,0.996917333733128,1.,0.996917333733128,1.,0.996917333733128,
1.,0.996917333733128,1.,0.996917333733128,1.,0.996917333733128,1.,0.996917333733128,
1.,0.996917333733128,1.,0.996917333733128,1.,0.996917333733128,1.,0.996917333733128,
1.,0.996917333733128,1.,0.996917333733128,1.,0.996917333733128,1.,0.996917333733128,
1.,0.996917333733128,1.,0.996917333733128,1.,0.996917333733128,1.,0.996917333733128,
1.,0.996917333733128,1.,0.996917333733128,1.,0.996917333733128,1.,0.996917333733128,
1.,0.996917333733128,1.,0.996917333733128,1.,0.996917333733128,1.,0.996917333733128,
1.,0.996917333733128,1.,0.996917333733128,1.,0.996917333733128,1.,0.996917333733128,
1.,0.996917333733128,1.,0.996917333733128,1.),(1.,0.996917333733128,1.,
0.996917333733128,1.,0.996917333733128,1.,0.996917333733128,1.,0.996917333733128,
1.,0.996917333733128,1.,0.996917333733128,1.,0.996917333733128,1.,0.996917333733128,
1.,0.996917333733128,1.,0.996917333733128,1.,0.996917333733128,1.,0.996917333733128,
1.,0.996917333733128,1.,0.996917333733128,1.,0.996917333733128,1.,0.996917333733128,
1.,0.996917333733128,1.,0.996917333733128,1.,0.996917333733128,1.,0.996917333733128,
1.,0.996917333733128,1.,0.996917333733128,1.,0.996917333733128,1.,0.996917333733128,
1.,0.996917333733128,1.,0.996917333733128,1.,0.996917333733128,1.,0.996917333733128,
1.,0.996917333733128,1.,0.996917333733128,1.,0.996917333733128,1.,0.996917333733128,
1.,0.996917333733128,1.,0.996917333733128,1.,0.996917333733128,1.,0.996917333733128,
1.,0.996917333733128,1.,0.996917333733128,1.,0.996917333733128,1.)))
REPRESENTATION_ITEM('')
SURFACE()
);
#4149=(
BOUNDED_CURVE()
B_SPLINE_CURVE(2,(#265333,#265334,#265335,#265336,#265337),
 .UNSPECIFIED.,.F.,.F.)
B_SPLINE_CURVE_WITH_KNOTS((3,2,3),(0.,0.025,0.0310216655371715),
 .UNSPECIFIED.)
CURVE()
GEOMETRIC_REPRESENTATION_ITEM()
RATIONAL_B_SPLINE_CURVE((1.,0.996917333733128,1.,0.999257488591127,0.998872669611195))
REPRESENTATION_ITEM('')
);
#4150=(
BOUNDED_CURVE()
B_SPLINE_CURVE(2,(#265340,#265341,#265342,#265343,#265344,#265345,#265346),
 .UNSPECIFIED.,.F.,.F.)
B_SPLINE_CURVE_WITH_KNOTS((3,2,2,3),(0.,0.025,0.05,0.0627352828483757),
 .UNSPECIFIED.)
CURVE()
GEOMETRIC_REPRESENTATION_ITEM()
RATIONAL_B_SPLINE_CURVE((1.,0.996917333733128,1.,0.996917333733128,1.,0.99842965492657,
0.998459212947514))
REPRESENTATION_ITEM('')
);
#4151=(
BOUNDED_CURVE()
B_SPLINE_CURVE(2,(#265512,#265513,#265514,#265515,#265516),
 .UNSPECIFIED.,.F.,.F.)
B_SPLINE_CURVE_WITH_KNOTS((3,2,3),(0.,0.025,0.0310216655371717),
 .UNSPECIFIED.)
CURVE()
GEOMETRIC_REPRESENTATION_ITEM()
RATIONAL_B_SPLINE_CURVE((1.,0.996917333733128,1.,0.999257488591127,0.998872669611196))
REPRESENTATION_ITEM('')
);
#4152=(
BOUNDED_CURVE()
B_SPLINE_CURVE(2,(#265690,#265691,#265692,#265693,#265694,#265695,#265696),
 .UNSPECIFIED.,.F.,.F.)
B_SPLINE_CURVE_WITH_KNOTS((3,2,2,3),(0.,0.025,0.05,0.0627352828483766),
 .UNSPECIFIED.)
CURVE()
GEOMETRIC_REPRESENTATION_ITEM()
RATIONAL_B_SPLINE_CURVE((1.,0.996917333733128,1.,0.996917333733128,1.,0.998429654926569,
0.998459212947514))
REPRESENTATION_ITEM('')
);
#4153=(
BOUNDED_CURVE()
B_SPLINE_CURVE(2,(#266037,#266038,#266039,#266040,#266041,#266042,#266043),
 .UNSPECIFIED.,.F.,.F.)
B_SPLINE_CURVE_WITH_KNOTS((3,2,2,3),(0.,0.025,0.05,0.0627352828483767),
 .UNSPECIFIED.)
CURVE()
GEOMETRIC_REPRESENTATION_ITEM()
RATIONAL_B_SPLINE_CURVE((1.,0.996917333733128,1.,0.996917333733128,1.,0.998429654926569,
0.998459212947514))
REPRESENTATION_ITEM('')
);
#4154=(
BOUNDED_CURVE()
B_SPLINE_CURVE(2,(#266046,#266047,#266048,#266049,#266050),
 .UNSPECIFIED.,.F.,.F.)
B_SPLINE_CURVE_WITH_KNOTS((3,2,3),(0.,0.025,0.0310216655371729),
 .UNSPECIFIED.)
CURVE()
GEOMETRIC_REPRESENTATION_ITEM()
RATIONAL_B_SPLINE_CURVE((1.,0.996917333733128,1.,0.999257488591127,0.998872669611195))
REPRESENTATION_ITEM('')
);
#4155=(
BOUNDED_CURVE()
B_SPLINE_CURVE(2,(#266216,#266217,#266218,#266219,#266220,#266221,#266222),
 .UNSPECIFIED.,.F.,.F.)
B_SPLINE_CURVE_WITH_KNOTS((3,2,2,3),(0.,0.025,0.05,0.0627352828483775),
 .UNSPECIFIED.)
CURVE()
GEOMETRIC_REPRESENTATION_ITEM()
RATIONAL_B_SPLINE_CURVE((1.,0.996917333733128,1.,0.996917333733128,1.,0.998429654926569,
0.998459212947514))
REPRESENTATION_ITEM('')
);
#4156=(
BOUNDED_CURVE()
B_SPLINE_CURVE(2,(#266396,#266397,#266398,#266399,#266400),
 .UNSPECIFIED.,.F.,.F.)
B_SPLINE_CURVE_WITH_KNOTS((3,2,3),(0.,0.025,0.0310216655371733),
 .UNSPECIFIED.)
CURVE()
GEOMETRIC_REPRESENTATION_ITEM()
RATIONAL_B_SPLINE_CURVE((1.,0.996917333733128,1.,0.999257488591127,0.998872669611195))
REPRESENTATION_ITEM('')
);
#4157=(
BOUNDED_CURVE()
B_SPLINE_CURVE(2,(#267289,#267290,#267291,#267292,#267293,#267294,#267295,
#267296,#267297,#267298,#267299,#267300,#267301,#267302,#267303,#267304,
#267305,#267306,#267307,#267308,#267309,#267310,#267311,#267312,#267313,
#267314,#267315,#267316,#267317,#267318,#267319,#267320,#267321,#267322,
#267323,#267324,#267325,#267326,#267327,#267328,#267329,#267330,#267331,
#267332,#267333,#267334,#267335,#267336,#267337,#267338,#267339,#267340,
#267341,#267342,#267343,#267344,#267345,#267346,#267347,#267348,#267349,
#267350,#267351,#267352,#267353,#267354,#267355,#267356,#267357,#267358,
#267359,#267360,#267361,#267362,#267363,#267364,#267365,#267366,#267367,
#267368,#267369),.UNSPECIFIED.,.F.,.F.)
B_SPLINE_CURVE_WITH_KNOTS((3,2,2,2,2,2,2,2,2,2,2,2,2,2,2,2,2,2,2,2,2,2,
2,2,2,2,2,2,2,2,2,2,2,2,2,2,2,2,2,2,3),(0.0125710582477619,0.025,0.05,0.075,
0.1,0.125,0.15,0.175,0.2,0.225,0.25,0.275,0.3,0.325,0.35,0.375,0.4,0.425,
0.45,0.475,0.5,0.525,0.55,0.575,0.6,0.625,0.65,0.675,0.7,0.725,0.75,0.775,
0.8,0.825,0.85,0.875,0.9,0.925,0.95,0.975,0.996408889531233),
 .UNSPECIFIED.)
CURVE()
GEOMETRIC_REPRESENTATION_ITEM()
RATIONAL_B_SPLINE_CURVE((0.998458716675295,0.998467428821098,1.,0.996917333733128,
1.,0.996917333733128,1.,0.996917333733128,1.,0.996917333733128,1.,0.996917333733128,
1.,0.996917333733128,1.,0.996917333733128,1.,0.996917333733128,1.,0.996917333733128,
1.,0.996917333733128,1.,0.996917333733128,1.,0.996917333733128,1.,0.996917333733128,
1.,0.996917333733128,1.,0.996917333733128,1.,0.996917333733128,1.,0.996917333733128,
1.,0.996917333733128,1.,0.996917333733128,1.,0.996917333733128,1.,0.996917333733128,
1.,0.996917333733128,1.,0.996917333733128,1.,0.996917333733128,1.,0.996917333733128,
1.,0.996917333733128,1.,0.996917333733128,1.,0.996917333733128,1.,0.996917333733128,
1.,0.996917333733128,1.,0.996917333733128,1.,0.996917333733128,1.,0.996917333733128,
1.,0.996917333733128,1.,0.996917333733128,1.,0.996917333733128,1.,0.996917333733128,
1.,0.996917333733128,1.,0.997360141537235,0.999241598131064))
REPRESENTATION_ITEM('')
);
#4158=(
BOUNDED_CURVE()
B_SPLINE_CURVE(2,(#267370,#267371,#267372,#267373,#267374,#267375,#267376,
#267377,#267378,#267379,#267380,#267381,#267382,#267383,#267384,#267385,
#267386,#267387,#267388,#267389,#267390,#267391,#267392,#267393,#267394,
#267395,#267396,#267397,#267398,#267399,#267400,#267401,#267402,#267403,
#267404,#267405,#267406,#267407,#267408,#267409,#267410,#267411,#267412,
#267413,#267414,#267415,#267416,#267417,#267418,#267419,#267420,#267421,
#267422,#267423,#267424,#267425,#267426,#267427,#267428,#267429,#267430,
#267431,#267432,#267433,#267434,#267435,#267436,#267437,#267438,#267439,
#267440,#267441,#267442,#267443,#267444,#267445,#267446,#267447,#267448,
#267449,#267450),.UNSPECIFIED.,.F.,.F.)
B_SPLINE_CURVE_WITH_KNOTS((3,2,2,2,2,2,2,2,2,2,2,2,2,2,2,2,2,2,2,2,2,2,
2,2,2,2,2,2,2,2,2,2,2,2,2,2,2,2,2,2,3),(0.00359111046876693,0.025,0.05,
0.075,0.1,0.125,0.15,0.175,0.2,0.225,0.25,0.275,0.3,0.325,0.35,0.375,0.4,
0.425,0.45,0.475,0.5,0.525,0.55,0.575,0.6,0.625,0.65,0.675,0.7,0.725,0.75,
0.775,0.8,0.825,0.85,0.875,0.9,0.925,0.95,0.975,0.987428941752238),
 .UNSPECIFIED.)
CURVE()
GEOMETRIC_REPRESENTATION_ITEM()
RATIONAL_B_SPLINE_CURVE((0.999241598131064,0.997360141537235,1.,0.996917333733128,
1.,0.996917333733128,1.,0.996917333733128,1.,0.996917333733128,1.,0.996917333733128,
1.,0.996917333733128,1.,0.996917333733128,1.,0.996917333733128,1.,0.996917333733128,
1.,0.996917333733128,1.,0.996917333733128,1.,0.996917333733128,1.,0.996917333733128,
1.,0.996917333733128,1.,0.996917333733128,1.,0.996917333733128,1.,0.996917333733128,
1.,0.996917333733128,1.,0.996917333733128,1.,0.996917333733128,1.,0.996917333733128,
1.,0.996917333733128,1.,0.996917333733128,1.,0.996917333733128,1.,0.996917333733128,
1.,0.996917333733128,1.,0.996917333733128,1.,0.996917333733128,1.,0.996917333733128,
1.,0.996917333733128,1.,0.996917333733128,1.,0.996917333733128,1.,0.996917333733128,
1.,0.996917333733128,1.,0.996917333733128,1.,0.996917333733128,1.,0.996917333733128,
1.,0.996917333733128,1.,0.998467428821098,0.998458716675295))
REPRESENTATION_ITEM('')
);
#4159=(
BOUNDED_CURVE()
B_SPLINE_CURVE(2,(#267613,#267614,#267615,#267616,#267617,#267618,#267619,
#267620,#267621,#267622,#267623,#267624,#267625,#267626,#267627,#267628,
#267629,#267630,#267631,#267632,#267633,#267634,#267635,#267636,#267637,
#267638,#267639,#267640,#267641,#267642,#267643,#267644,#267645,#267646,
#267647,#267648,#267649,#267650,#267651,#267652,#267653,#267654,#267655,
#267656,#267657,#267658,#267659,#267660,#267661,#267662,#267663,#267664,
#267665,#267666,#267667,#267668,#267669,#267670,#267671,#267672,#267673,
#267674,#267675,#267676,#267677,#267678,#267679,#267680,#267681,#267682,
#267683,#267684,#267685,#267686,#267687,#267688,#267689,#267690,#267691,
#267692,#267693),.UNSPECIFIED.,.F.,.F.)
B_SPLINE_CURVE_WITH_KNOTS((3,2,2,2,2,2,2,2,2,2,2,2,2,2,2,2,2,2,2,2,2,2,
2,2,2,2,2,2,2,2,2,2,2,2,2,2,2,2,2,2,3),(0.00288613200956877,0.025,0.05,
0.075,0.1,0.125,0.15,0.175,0.2,0.225,0.25,0.275,0.3,0.325,0.35,0.375,0.4,
0.425,0.45,0.475,0.5,0.525,0.55,0.575,0.6,0.625,0.65,0.675,0.7,0.725,0.75,
0.775,0.8,0.825,0.85,0.875,0.9,0.925,0.95,0.975,0.98954155634899),
 .UNSPECIFIED.)
CURVE()
GEOMETRIC_REPRESENTATION_ITEM()
RATIONAL_B_SPLINE_CURVE((0.999370410621552,0.997273213004633,1.,0.996917333733128,
1.,0.996917333733128,1.,0.996917333733128,1.,0.996917333733128,1.,0.996917333733128,
1.,0.996917333733128,1.,0.996917333733128,1.,0.996917333733128,1.,0.996917333733128,
1.,0.996917333733128,1.,0.996917333733128,1.,0.996917333733128,1.,0.996917333733128,
1.,0.996917333733128,1.,0.996917333733128,1.,0.996917333733128,1.,0.996917333733128,
1.,0.996917333733128,1.,0.996917333733128,1.,0.996917333733128,1.,0.996917333733128,
1.,0.996917333733128,1.,0.996917333733128,1.,0.996917333733128,1.,0.996917333733128,
1.,0.996917333733128,1.,0.996917333733128,1.,0.996917333733128,1.,0.996917333733128,
1.,0.996917333733128,1.,0.996917333733128,1.,0.996917333733128,1.,0.996917333733128,
1.,0.996917333733128,1.,0.996917333733128,1.,0.996917333733128,1.,0.996917333733128,
1.,0.996917333733128,1.,0.998206929391006,0.998499781765884))
REPRESENTATION_ITEM('')
);
#4160=(
BOUNDED_CURVE()
B_SPLINE_CURVE(2,(#267856,#267857,#267858,#267859,#267860,#267861,#267862,
#267863,#267864,#267865,#267866,#267867,#267868,#267869,#267870,#267871,
#267872,#267873,#267874,#267875,#267876,#267877,#267878,#267879,#267880,
#267881,#267882,#267883,#267884,#267885,#267886,#267887,#267888,#267889,
#267890,#267891,#267892,#267893,#267894,#267895,#267896,#267897,#267898,
#267899,#267900,#267901,#267902,#267903,#267904,#267905,#267906,#267907,
#267908,#267909,#267910,#267911,#267912,#267913,#267914,#267915,#267916,
#267917,#267918,#267919,#267920,#267921,#267922,#267923,#267924,#267925,
#267926,#267927,#267928,#267929,#267930,#267931,#267932,#267933,#267934,
#267935,#267936),.UNSPECIFIED.,.F.,.F.)
B_SPLINE_CURVE_WITH_KNOTS((3,2,2,2,2,2,2,2,2,2,2,2,2,2,2,2,2,2,2,2,2,2,
2,2,2,2,2,2,2,2,2,2,2,2,2,2,2,2,2,2,3),(0.0104584436510098,0.025,0.05,0.075,
0.1,0.125,0.15,0.175,0.2,0.225,0.25,0.275,0.3,0.325,0.35,0.375,0.4,0.425,
0.45,0.475,0.5,0.525,0.55,0.575,0.6,0.625,0.65,0.675,0.7,0.725,0.75,0.775,
0.8,0.825,0.85,0.875,0.9,0.925,0.95,0.975,0.997113867990431),
 .UNSPECIFIED.)
CURVE()
GEOMETRIC_REPRESENTATION_ITEM()
RATIONAL_B_SPLINE_CURVE((0.998499781765884,0.998206929391006,1.,0.996917333733128,
1.,0.996917333733128,1.,0.996917333733128,1.,0.996917333733128,1.,0.996917333733128,
1.,0.996917333733128,1.,0.996917333733128,1.,0.996917333733128,1.,0.996917333733128,
1.,0.996917333733128,1.,0.996917333733128,1.,0.996917333733128,1.,0.996917333733128,
1.,0.996917333733128,1.,0.996917333733128,1.,0.996917333733128,1.,0.996917333733128,
1.,0.996917333733128,1.,0.996917333733128,1.,0.996917333733128,1.,0.996917333733128,
1.,0.996917333733128,1.,0.996917333733128,1.,0.996917333733128,1.,0.996917333733128,
1.,0.996917333733128,1.,0.996917333733128,1.,0.996917333733128,1.,0.996917333733128,
1.,0.996917333733128,1.,0.996917333733128,1.,0.996917333733128,1.,0.996917333733128,
1.,0.996917333733128,1.,0.996917333733128,1.,0.996917333733128,1.,0.996917333733128,
1.,0.996917333733128,1.,0.997273213004633,0.999370410621552))
REPRESENTATION_ITEM('')
);
#4161=(
BOUNDED_CURVE()
B_SPLINE_CURVE(2,(#268941,#268942,#268943,#268944,#268945,#268946,#268947,
#268948,#268949,#268950,#268951,#268952,#268953,#268954,#268955,#268956,
#268957,#268958,#268959,#268960,#268961,#268962,#268963,#268964,#268965,
#268966,#268967,#268968,#268969,#268970,#268971,#268972,#268973,#268974,
#268975,#268976,#268977,#268978,#268979,#268980,#268981,#268982,#268983,
#268984,#268985,#268986,#268987,#268988,#268989,#268990,#268991,#268992,
#268993,#268994,#268995,#268996,#268997,#268998,#268999,#269000,#269001,
#269002,#269003,#269004,#269005,#269006,#269007,#269008,#269009,#269010,
#269011,#269012,#269013,#269014,#269015,#269016,#269017,#269018,#269019,
#269020,#269021),.UNSPECIFIED.,.F.,.F.)
B_SPLINE_CURVE_WITH_KNOTS((3,2,2,2,2,2,2,2,2,2,2,2,2,2,2,2,2,2,2,2,2,2,
2,2,2,2,2,2,2,2,2,2,2,2,2,2,2,2,2,2,3),(0.00359111046876831,0.025,0.05,
0.075,0.1,0.125,0.15,0.175,0.2,0.225,0.25,0.275,0.3,0.325,0.35,0.375,0.4,
0.425,0.45,0.475,0.5,0.525,0.55,0.575,0.6,0.625,0.65,0.675,0.7,0.725,0.75,
0.775,0.8,0.825,0.85,0.875,0.9,0.925,0.95,0.975,0.987428941752238),
 .UNSPECIFIED.)
CURVE()
GEOMETRIC_REPRESENTATION_ITEM()
RATIONAL_B_SPLINE_CURVE((0.999241598131064,0.997360141537235,1.,0.996917333733128,
1.,0.996917333733128,1.,0.996917333733128,1.,0.996917333733128,1.,0.996917333733128,
1.,0.996917333733128,1.,0.996917333733128,1.,0.996917333733128,1.,0.996917333733128,
1.,0.996917333733128,1.,0.996917333733128,1.,0.996917333733128,1.,0.996917333733128,
1.,0.996917333733128,1.,0.996917333733128,1.,0.996917333733128,1.,0.996917333733128,
1.,0.996917333733128,1.,0.996917333733128,1.,0.996917333733128,1.,0.996917333733128,
1.,0.996917333733128,1.,0.996917333733128,1.,0.996917333733128,1.,0.996917333733128,
1.,0.996917333733128,1.,0.996917333733128,1.,0.996917333733128,1.,0.996917333733128,
1.,0.996917333733128,1.,0.996917333733128,1.,0.996917333733128,1.,0.996917333733128,
1.,0.996917333733128,1.,0.996917333733128,1.,0.996917333733128,1.,0.996917333733128,
1.,0.996917333733128,1.,0.998467428821098,0.998458716675295))
REPRESENTATION_ITEM('')
);
#4162=(
BOUNDED_CURVE()
B_SPLINE_CURVE(2,(#269022,#269023,#269024,#269025,#269026,#269027,#269028,
#269029,#269030,#269031,#269032,#269033,#269034,#269035,#269036,#269037,
#269038,#269039,#269040,#269041,#269042,#269043,#269044,#269045,#269046,
#269047,#269048,#269049,#269050,#269051,#269052,#269053,#269054,#269055,
#269056,#269057,#269058,#269059,#269060,#269061,#269062,#269063,#269064,
#269065,#269066,#269067,#269068,#269069,#269070,#269071,#269072,#269073,
#269074,#269075,#269076,#269077,#269078,#269079,#269080,#269081,#269082,
#269083,#269084,#269085,#269086,#269087,#269088,#269089,#269090,#269091,
#269092,#269093,#269094,#269095,#269096,#269097,#269098,#269099,#269100,
#269101,#269102),.UNSPECIFIED.,.F.,.F.)
B_SPLINE_CURVE_WITH_KNOTS((3,2,2,2,2,2,2,2,2,2,2,2,2,2,2,2,2,2,2,2,2,2,
2,2,2,2,2,2,2,2,2,2,2,2,2,2,2,2,2,2,3),(0.0125710582477632,0.025,0.05,0.075,
0.1,0.125,0.15,0.175,0.2,0.225,0.25,0.275,0.3,0.325,0.35,0.375,0.4,0.425,
0.45,0.475,0.5,0.525,0.55,0.575,0.6,0.625,0.65,0.675,0.7,0.725,0.75,0.775,
0.8,0.825,0.85,0.875,0.9,0.925,0.95,0.975,0.996408889531233),
 .UNSPECIFIED.)
CURVE()
GEOMETRIC_REPRESENTATION_ITEM()
RATIONAL_B_SPLINE_CURVE((0.998458716675295,0.998467428821098,1.,0.996917333733128,
1.,0.996917333733128,1.,0.996917333733128,1.,0.996917333733128,1.,0.996917333733128,
1.,0.996917333733128,1.,0.996917333733128,1.,0.996917333733128,1.,0.996917333733128,
1.,0.996917333733128,1.,0.996917333733128,1.,0.996917333733128,1.,0.996917333733128,
1.,0.996917333733128,1.,0.996917333733128,1.,0.996917333733128,1.,0.996917333733128,
1.,0.996917333733128,1.,0.996917333733128,1.,0.996917333733128,1.,0.996917333733128,
1.,0.996917333733128,1.,0.996917333733128,1.,0.996917333733128,1.,0.996917333733128,
1.,0.996917333733128,1.,0.996917333733128,1.,0.996917333733128,1.,0.996917333733128,
1.,0.996917333733128,1.,0.996917333733128,1.,0.996917333733128,1.,0.996917333733128,
1.,0.996917333733128,1.,0.996917333733128,1.,0.996917333733128,1.,0.996917333733128,
1.,0.996917333733128,1.,0.997360141537235,0.999241598131064))
REPRESENTATION_ITEM('')
);
#4163=(
BOUNDED_CURVE()
B_SPLINE_CURVE(2,(#269265,#269266,#269267,#269268,#269269,#269270,#269271,
#269272,#269273,#269274,#269275,#269276,#269277,#269278,#269279,#269280,
#269281,#269282,#269283,#269284,#269285,#269286,#269287,#269288,#269289,
#269290,#269291,#269292,#269293,#269294,#269295,#269296,#269297,#269298,
#269299,#269300,#269301,#269302,#269303,#269304,#269305,#269306,#269307,
#269308,#269309,#269310,#269311,#269312,#269313,#269314,#269315,#269316,
#269317,#269318,#269319,#269320,#269321,#269322,#269323,#269324,#269325,
#269326,#269327,#269328,#269329,#269330,#269331,#269332,#269333,#269334,
#269335,#269336,#269337,#269338,#269339,#269340,#269341,#269342,#269343,
#269344,#269345),.UNSPECIFIED.,.F.,.F.)
B_SPLINE_CURVE_WITH_KNOTS((3,2,2,2,2,2,2,2,2,2,2,2,2,2,2,2,2,2,2,2,2,2,
2,2,2,2,2,2,2,2,2,2,2,2,2,2,2,2,2,2,3),(0.00288613200956991,0.025,0.05,
0.075,0.1,0.125,0.15,0.175,0.2,0.225,0.25,0.275,0.3,0.325,0.35,0.375,0.4,
0.425,0.45,0.475,0.5,0.525,0.55,0.575,0.6,0.625,0.65,0.675,0.7,0.725,0.75,
0.775,0.8,0.825,0.85,0.875,0.9,0.925,0.95,0.975,0.98954155634899),
 .UNSPECIFIED.)
CURVE()
GEOMETRIC_REPRESENTATION_ITEM()
RATIONAL_B_SPLINE_CURVE((0.999370410621551,0.997273213004634,1.,0.996917333733128,
1.,0.996917333733128,1.,0.996917333733128,1.,0.996917333733128,1.,0.996917333733128,
1.,0.996917333733128,1.,0.996917333733128,1.,0.996917333733128,1.,0.996917333733128,
1.,0.996917333733128,1.,0.996917333733128,1.,0.996917333733128,1.,0.996917333733128,
1.,0.996917333733128,1.,0.996917333733128,1.,0.996917333733128,1.,0.996917333733128,
1.,0.996917333733128,1.,0.996917333733128,1.,0.996917333733128,1.,0.996917333733128,
1.,0.996917333733128,1.,0.996917333733128,1.,0.996917333733128,1.,0.996917333733128,
1.,0.996917333733128,1.,0.996917333733128,1.,0.996917333733128,1.,0.996917333733128,
1.,0.996917333733128,1.,0.996917333733128,1.,0.996917333733128,1.,0.996917333733128,
1.,0.996917333733128,1.,0.996917333733128,1.,0.996917333733128,1.,0.996917333733128,
1.,0.996917333733128,1.,0.998206929391006,0.998499781765884))
REPRESENTATION_ITEM('')
);
#4164=(
BOUNDED_CURVE()
B_SPLINE_CURVE(2,(#269508,#269509,#269510,#269511,#269512,#269513,#269514,
#269515,#269516,#269517,#269518,#269519,#269520,#269521,#269522,#269523,
#269524,#269525,#269526,#269527,#269528,#269529,#269530,#269531,#269532,
#269533,#269534,#269535,#269536,#269537,#269538,#269539,#269540,#269541,
#269542,#269543,#269544,#269545,#269546,#269547,#269548,#269549,#269550,
#269551,#269552,#269553,#269554,#269555,#269556,#269557,#269558,#269559,
#269560,#269561,#269562,#269563,#269564,#269565,#269566,#269567,#269568,
#269569,#269570,#269571,#269572,#269573,#269574,#269575,#269576,#269577,
#269578,#269579,#269580,#269581,#269582,#269583,#269584,#269585,#269586,
#269587,#269588),.UNSPECIFIED.,.F.,.F.)
B_SPLINE_CURVE_WITH_KNOTS((3,2,2,2,2,2,2,2,2,2,2,2,2,2,2,2,2,2,2,2,2,2,
2,2,2,2,2,2,2,2,2,2,2,2,2,2,2,2,2,2,3),(0.0104584436510109,0.025,0.05,0.075,
0.1,0.125,0.15,0.175,0.2,0.225,0.25,0.275,0.3,0.325,0.35,0.375,0.4,0.425,
0.45,0.475,0.5,0.525,0.55,0.575,0.6,0.625,0.65,0.675,0.7,0.725,0.75,0.775,
0.8,0.825,0.85,0.875,0.9,0.925,0.95,0.975,0.997113867990431),
 .UNSPECIFIED.)
CURVE()
GEOMETRIC_REPRESENTATION_ITEM()
RATIONAL_B_SPLINE_CURVE((0.998499781765884,0.998206929391006,1.,0.996917333733128,
1.,0.996917333733128,1.,0.996917333733128,1.,0.996917333733128,1.,0.996917333733128,
1.,0.996917333733128,1.,0.996917333733128,1.,0.996917333733128,1.,0.996917333733128,
1.,0.996917333733128,1.,0.996917333733128,1.,0.996917333733128,1.,0.996917333733128,
1.,0.996917333733128,1.,0.996917333733128,1.,0.996917333733128,1.,0.996917333733128,
1.,0.996917333733128,1.,0.996917333733128,1.,0.996917333733128,1.,0.996917333733128,
1.,0.996917333733128,1.,0.996917333733128,1.,0.996917333733128,1.,0.996917333733128,
1.,0.996917333733128,1.,0.996917333733128,1.,0.996917333733128,1.,0.996917333733128,
1.,0.996917333733128,1.,0.996917333733128,1.,0.996917333733128,1.,0.996917333733128,
1.,0.996917333733128,1.,0.996917333733128,1.,0.996917333733128,1.,0.996917333733128,
1.,0.996917333733128,1.,0.997273213004633,0.999370410621552))
REPRESENTATION_ITEM('')
);
#4165=(
BOUNDED_CURVE()
B_SPLINE_CURVE(2,(#269913,#269914,#269915,#269916,#269917,#269918,#269919,
#269920,#269921,#269922,#269923,#269924,#269925,#269926,#269927,#269928,
#269929,#269930,#269931,#269932,#269933,#269934,#269935,#269936,#269937,
#269938,#269939,#269940,#269941,#269942,#269943,#269944,#269945,#269946,
#269947,#269948,#269949,#269950,#269951,#269952,#269953,#269954,#269955,
#269956,#269957,#269958,#269959,#269960,#269961,#269962,#269963,#269964,
#269965,#269966,#269967,#269968,#269969,#269970,#269971,#269972,#269973,
#269974,#269975,#269976,#269977,#269978,#269979,#269980,#269981,#269982,
#269983,#269984,#269985,#269986,#269987,#269988,#269989,#269990,#269991,
#269992,#269993),.UNSPECIFIED.,.F.,.F.)
B_SPLINE_CURVE_WITH_KNOTS((3,2,2,2,2,2,2,2,2,2,2,2,2,2,2,2,2,2,2,2,2,2,
2,2,2,2,2,2,2,2,2,2,2,2,2,2,2,2,2,2,3),(0.0104584436510113,0.025,0.05,0.075,
0.1,0.125,0.15,0.175,0.2,0.225,0.25,0.275,0.3,0.325,0.35,0.375,0.4,0.425,
0.45,0.475,0.5,0.525,0.55,0.575,0.6,0.625,0.65,0.675,0.7,0.725,0.75,0.775,
0.8,0.825,0.85,0.875,0.9,0.925,0.95,0.975,0.997113867990431),
 .UNSPECIFIED.)
CURVE()
GEOMETRIC_REPRESENTATION_ITEM()
RATIONAL_B_SPLINE_CURVE((0.998499781765884,0.998206929391006,1.,0.996917333733128,
1.,0.996917333733128,1.,0.996917333733128,1.,0.996917333733128,1.,0.996917333733128,
1.,0.996917333733128,1.,0.996917333733128,1.,0.996917333733128,1.,0.996917333733128,
1.,0.996917333733128,1.,0.996917333733128,1.,0.996917333733128,1.,0.996917333733128,
1.,0.996917333733128,1.,0.996917333733128,1.,0.996917333733128,1.,0.996917333733128,
1.,0.996917333733128,1.,0.996917333733128,1.,0.996917333733128,1.,0.996917333733128,
1.,0.996917333733128,1.,0.996917333733128,1.,0.996917333733128,1.,0.996917333733128,
1.,0.996917333733128,1.,0.996917333733128,1.,0.996917333733128,1.,0.996917333733128,
1.,0.996917333733128,1.,0.996917333733128,1.,0.996917333733128,1.,0.996917333733128,
1.,0.996917333733128,1.,0.996917333733128,1.,0.996917333733128,1.,0.996917333733128,
1.,0.996917333733128,1.,0.997273213004634,0.999370410621552))
REPRESENTATION_ITEM('')
);
#4166=(
BOUNDED_CURVE()
B_SPLINE_CURVE(2,(#269994,#269995,#269996,#269997,#269998,#269999,#270000,
#270001,#270002,#270003,#270004,#270005,#270006,#270007,#270008,#270009,
#270010,#270011,#270012,#270013,#270014,#270015,#270016,#270017,#270018,
#270019,#270020,#270021,#270022,#270023,#270024,#270025,#270026,#270027,
#270028,#270029,#270030,#270031,#270032,#270033,#270034,#270035,#270036,
#270037,#270038,#270039,#270040,#270041,#270042,#270043,#270044,#270045,
#270046,#270047,#270048,#270049,#270050,#270051,#270052,#270053,#270054,
#270055,#270056,#270057,#270058,#270059,#270060,#270061,#270062,#270063,
#270064,#270065,#270066,#270067,#270068,#270069,#270070,#270071,#270072,
#270073,#270074),.UNSPECIFIED.,.F.,.F.)
B_SPLINE_CURVE_WITH_KNOTS((3,2,2,2,2,2,2,2,2,2,2,2,2,2,2,2,2,2,2,2,2,2,
2,2,2,2,2,2,2,2,2,2,2,2,2,2,2,2,2,2,3),(0.00288613200957066,0.025,0.05,
0.075,0.1,0.125,0.15,0.175,0.2,0.225,0.25,0.275,0.3,0.325,0.35,0.375,0.4,
0.425,0.45,0.475,0.5,0.525,0.55,0.575,0.6,0.625,0.65,0.675,0.7,0.725,0.75,
0.775,0.8,0.825,0.85,0.875,0.9,0.925,0.95,0.975,0.98954155634899),
 .UNSPECIFIED.)
CURVE()
GEOMETRIC_REPRESENTATION_ITEM()
RATIONAL_B_SPLINE_CURVE((0.999370410621551,0.997273213004634,1.,0.996917333733128,
1.,0.996917333733128,1.,0.996917333733128,1.,0.996917333733128,1.,0.996917333733128,
1.,0.996917333733128,1.,0.996917333733128,1.,0.996917333733128,1.,0.996917333733128,
1.,0.996917333733128,1.,0.996917333733128,1.,0.996917333733128,1.,0.996917333733128,
1.,0.996917333733128,1.,0.996917333733128,1.,0.996917333733128,1.,0.996917333733128,
1.,0.996917333733128,1.,0.996917333733128,1.,0.996917333733128,1.,0.996917333733128,
1.,0.996917333733128,1.,0.996917333733128,1.,0.996917333733128,1.,0.996917333733128,
1.,0.996917333733128,1.,0.996917333733128,1.,0.996917333733128,1.,0.996917333733128,
1.,0.996917333733128,1.,0.996917333733128,1.,0.996917333733128,1.,0.996917333733128,
1.,0.996917333733128,1.,0.996917333733128,1.,0.996917333733128,1.,0.996917333733128,
1.,0.996917333733128,1.,0.998206929391006,0.998499781765884))
REPRESENTATION_ITEM('')
);
#4167=(
BOUNDED_CURVE()
B_SPLINE_CURVE(2,(#270237,#270238,#270239,#270240,#270241,#270242,#270243,
#270244,#270245,#270246,#270247,#270248,#270249,#270250,#270251,#270252,
#270253,#270254,#270255,#270256,#270257,#270258,#270259,#270260,#270261,
#270262,#270263,#270264,#270265,#270266,#270267,#270268,#270269,#270270,
#270271,#270272,#270273,#270274,#270275,#270276,#270277,#270278,#270279,
#270280,#270281,#270282,#270283,#270284,#270285,#270286,#270287,#270288,
#270289,#270290,#270291,#270292,#270293,#270294,#270295,#270296,#270297,
#270298,#270299,#270300,#270301,#270302,#270303,#270304,#270305,#270306,
#270307,#270308,#270309,#270310,#270311,#270312,#270313,#270314,#270315,
#270316,#270317),.UNSPECIFIED.,.F.,.F.)
B_SPLINE_CURVE_WITH_KNOTS((3,2,2,2,2,2,2,2,2,2,2,2,2,2,2,2,2,2,2,2,2,2,
2,2,2,2,2,2,2,2,2,2,2,2,2,2,2,2,2,2,3),(0.0125710582477639,0.025,0.05,0.075,
0.1,0.125,0.15,0.175,0.2,0.225,0.25,0.275,0.3,0.325,0.35,0.375,0.4,0.425,
0.45,0.475,0.5,0.525,0.55,0.575,0.6,0.625,0.65,0.675,0.7,0.725,0.75,0.775,
0.8,0.825,0.85,0.875,0.9,0.925,0.95,0.975,0.996408889531232),
 .UNSPECIFIED.)
CURVE()
GEOMETRIC_REPRESENTATION_ITEM()
RATIONAL_B_SPLINE_CURVE((0.998458716675295,0.998467428821099,1.,0.996917333733128,
1.,0.996917333733128,1.,0.996917333733128,1.,0.996917333733128,1.,0.996917333733128,
1.,0.996917333733128,1.,0.996917333733128,1.,0.996917333733128,1.,0.996917333733128,
1.,0.996917333733128,1.,0.996917333733128,1.,0.996917333733128,1.,0.996917333733128,
1.,0.996917333733128,1.,0.996917333733128,1.,0.996917333733128,1.,0.996917333733128,
1.,0.996917333733128,1.,0.996917333733128,1.,0.996917333733128,1.,0.996917333733128,
1.,0.996917333733128,1.,0.996917333733128,1.,0.996917333733128,1.,0.996917333733128,
1.,0.996917333733128,1.,0.996917333733128,1.,0.996917333733128,1.,0.996917333733128,
1.,0.996917333733128,1.,0.996917333733128,1.,0.996917333733128,1.,0.996917333733128,
1.,0.996917333733128,1.,0.996917333733128,1.,0.996917333733128,1.,0.996917333733128,
1.,0.996917333733128,1.,0.997360141537235,0.999241598131064))
REPRESENTATION_ITEM('')
);
#4168=(
BOUNDED_CURVE()
B_SPLINE_CURVE(2,(#270480,#270481,#270482,#270483,#270484,#270485,#270486,
#270487,#270488,#270489,#270490,#270491,#270492,#270493,#270494,#270495,
#270496,#270497,#270498,#270499,#270500,#270501,#270502,#270503,#270504,
#270505,#270506,#270507,#270508,#270509,#270510,#270511,#270512,#270513,
#270514,#270515,#270516,#270517,#270518,#270519,#270520,#270521,#270522,
#270523,#270524,#270525,#270526,#270527,#270528,#270529,#270530,#270531,
#270532,#270533,#270534,#270535,#270536,#270537,#270538,#270539,#270540,
#270541,#270542,#270543,#270544,#270545,#270546,#270547,#270548,#270549,
#270550,#270551,#270552,#270553,#270554,#270555,#270556,#270557,#270558,
#270559,#270560),.UNSPECIFIED.,.F.,.F.)
B_SPLINE_CURVE_WITH_KNOTS((3,2,2,2,2,2,2,2,2,2,2,2,2,2,2,2,2,2,2,2,2,2,
2,2,2,2,2,2,2,2,2,2,2,2,2,2,2,2,2,2,3),(0.00359111046876932,0.025,0.05,
0.075,0.1,0.125,0.15,0.175,0.2,0.225,0.25,0.275,0.3,0.325,0.35,0.375,0.4,
0.425,0.45,0.475,0.5,0.525,0.55,0.575,0.6,0.625,0.65,0.675,0.7,0.725,0.75,
0.775,0.8,0.825,0.85,0.875,0.9,0.925,0.95,0.975,0.987428941752237),
 .UNSPECIFIED.)
CURVE()
GEOMETRIC_REPRESENTATION_ITEM()
RATIONAL_B_SPLINE_CURVE((0.999241598131064,0.997360141537235,1.,0.996917333733128,
1.,0.996917333733128,1.,0.996917333733128,1.,0.996917333733128,1.,0.996917333733128,
1.,0.996917333733128,1.,0.996917333733128,1.,0.996917333733128,1.,0.996917333733128,
1.,0.996917333733128,1.,0.996917333733128,1.,0.996917333733128,1.,0.996917333733128,
1.,0.996917333733128,1.,0.996917333733128,1.,0.996917333733128,1.,0.996917333733128,
1.,0.996917333733128,1.,0.996917333733128,1.,0.996917333733128,1.,0.996917333733128,
1.,0.996917333733128,1.,0.996917333733128,1.,0.996917333733128,1.,0.996917333733128,
1.,0.996917333733128,1.,0.996917333733128,1.,0.996917333733128,1.,0.996917333733128,
1.,0.996917333733128,1.,0.996917333733128,1.,0.996917333733128,1.,0.996917333733128,
1.,0.996917333733128,1.,0.996917333733128,1.,0.996917333733128,1.,0.996917333733128,
1.,0.996917333733128,1.,0.998467428821098,0.998458716675295))
REPRESENTATION_ITEM('')
);
#4169=(
BOUNDED_CURVE()
B_SPLINE_CURVE(2,(#270885,#270886,#270887,#270888,#270889,#270890,#270891,
#270892,#270893,#270894,#270895,#270896,#270897,#270898,#270899,#270900,
#270901,#270902,#270903,#270904,#270905,#270906,#270907,#270908,#270909,
#270910,#270911,#270912,#270913,#270914,#270915,#270916,#270917,#270918,
#270919,#270920,#270921,#270922,#270923,#270924,#270925,#270926,#270927,
#270928,#270929,#270930,#270931,#270932,#270933,#270934,#270935,#270936,
#270937,#270938,#270939,#270940,#270941,#270942,#270943,#270944,#270945,
#270946,#270947,#270948,#270949,#270950,#270951,#270952,#270953,#270954,
#270955,#270956,#270957,#270958,#270959,#270960,#270961,#270962,#270963,
#270964,#270965),.UNSPECIFIED.,.F.,.F.)
B_SPLINE_CURVE_WITH_KNOTS((3,2,2,2,2,2,2,2,2,2,2,2,2,2,2,2,2,2,2,2,2,2,
2,2,2,2,2,2,2,2,2,2,2,2,2,2,2,2,2,2,3),(0.0125710582477628,0.025,0.05,0.075,
0.1,0.125,0.15,0.175,0.2,0.225,0.25,0.275,0.3,0.325,0.35,0.375,0.4,0.425,
0.45,0.475,0.5,0.525,0.55,0.575,0.6,0.625,0.65,0.675,0.7,0.725,0.75,0.775,
0.8,0.825,0.85,0.875,0.9,0.925,0.95,0.975,0.996408889531232),
 .UNSPECIFIED.)
CURVE()
GEOMETRIC_REPRESENTATION_ITEM()
RATIONAL_B_SPLINE_CURVE((0.998458716675295,0.998467428821098,1.,0.996917333733128,
1.,0.996917333733128,1.,0.996917333733128,1.,0.996917333733128,1.,0.996917333733128,
1.,0.996917333733128,1.,0.996917333733128,1.,0.996917333733128,1.,0.996917333733128,
1.,0.996917333733128,1.,0.996917333733128,1.,0.996917333733128,1.,0.996917333733128,
1.,0.996917333733128,1.,0.996917333733128,1.,0.996917333733128,1.,0.996917333733128,
1.,0.996917333733128,1.,0.996917333733128,1.,0.996917333733128,1.,0.996917333733128,
1.,0.996917333733128,1.,0.996917333733128,1.,0.996917333733128,1.,0.996917333733128,
1.,0.996917333733128,1.,0.996917333733128,1.,0.996917333733128,1.,0.996917333733128,
1.,0.996917333733128,1.,0.996917333733128,1.,0.996917333733128,1.,0.996917333733128,
1.,0.996917333733128,1.,0.996917333733128,1.,0.996917333733128,1.,0.996917333733128,
1.,0.996917333733128,1.,0.997360141537235,0.999241598131064))
REPRESENTATION_ITEM('')
);
#4170=(
BOUNDED_CURVE()
B_SPLINE_CURVE(2,(#270966,#270967,#270968,#270969,#270970,#270971,#270972,
#270973,#270974,#270975,#270976,#270977,#270978,#270979,#270980,#270981,
#270982,#270983,#270984,#270985,#270986,#270987,#270988,#270989,#270990,
#270991,#270992,#270993,#270994,#270995,#270996,#270997,#270998,#270999,
#271000,#271001,#271002,#271003,#271004,#271005,#271006,#271007,#271008,
#271009,#271010,#271011,#271012,#271013,#271014,#271015,#271016,#271017,
#271018,#271019,#271020,#271021,#271022,#271023,#271024,#271025,#271026,
#271027,#271028,#271029,#271030,#271031,#271032,#271033,#271034,#271035,
#271036,#271037,#271038,#271039,#271040,#271041,#271042,#271043,#271044,
#271045,#271046),.UNSPECIFIED.,.F.,.F.)
B_SPLINE_CURVE_WITH_KNOTS((3,2,2,2,2,2,2,2,2,2,2,2,2,2,2,2,2,2,2,2,2,2,
2,2,2,2,2,2,2,2,2,2,2,2,2,2,2,2,2,2,3),(0.00359111046876783,0.025,0.05,
0.075,0.1,0.125,0.15,0.175,0.2,0.225,0.25,0.275,0.3,0.325,0.35,0.375,0.4,
0.425,0.45,0.475,0.5,0.525,0.55,0.575,0.6,0.625,0.65,0.675,0.7,0.725,0.75,
0.775,0.8,0.825,0.85,0.875,0.9,0.925,0.95,0.975,0.987428941752237),
 .UNSPECIFIED.)
CURVE()
GEOMETRIC_REPRESENTATION_ITEM()
RATIONAL_B_SPLINE_CURVE((0.999241598131064,0.997360141537235,1.,0.996917333733128,
1.,0.996917333733128,1.,0.996917333733128,1.,0.996917333733128,1.,0.996917333733128,
1.,0.996917333733128,1.,0.996917333733128,1.,0.996917333733128,1.,0.996917333733128,
1.,0.996917333733128,1.,0.996917333733128,1.,0.996917333733128,1.,0.996917333733128,
1.,0.996917333733128,1.,0.996917333733128,1.,0.996917333733128,1.,0.996917333733128,
1.,0.996917333733128,1.,0.996917333733128,1.,0.996917333733128,1.,0.996917333733128,
1.,0.996917333733128,1.,0.996917333733128,1.,0.996917333733128,1.,0.996917333733128,
1.,0.996917333733128,1.,0.996917333733128,1.,0.996917333733128,1.,0.996917333733128,
1.,0.996917333733128,1.,0.996917333733128,1.,0.996917333733128,1.,0.996917333733128,
1.,0.996917333733128,1.,0.996917333733128,1.,0.996917333733128,1.,0.996917333733128,
1.,0.996917333733128,1.,0.998467428821098,0.998458716675295))
REPRESENTATION_ITEM('')
);
#4171=(
BOUNDED_CURVE()
B_SPLINE_CURVE(2,(#271209,#271210,#271211,#271212,#271213,#271214,#271215,
#271216,#271217,#271218,#271219,#271220,#271221,#271222,#271223,#271224,
#271225,#271226,#271227,#271228,#271229,#271230,#271231,#271232,#271233,
#271234,#271235,#271236,#271237,#271238,#271239,#271240,#271241,#271242,
#271243,#271244,#271245,#271246,#271247,#271248,#271249,#271250,#271251,
#271252,#271253,#271254,#271255,#271256,#271257,#271258,#271259,#271260,
#271261,#271262,#271263,#271264,#271265,#271266,#271267,#271268,#271269,
#271270,#271271,#271272,#271273,#271274,#271275,#271276,#271277,#271278,
#271279,#271280,#271281,#271282,#271283,#271284,#271285,#271286,#271287,
#271288,#271289),.UNSPECIFIED.,.F.,.F.)
B_SPLINE_CURVE_WITH_KNOTS((3,2,2,2,2,2,2,2,2,2,2,2,2,2,2,2,2,2,2,2,2,2,
2,2,2,2,2,2,2,2,2,2,2,2,2,2,2,2,2,2,3),(0.0104584436510103,0.025,0.05,0.075,
0.1,0.125,0.15,0.175,0.2,0.225,0.25,0.275,0.3,0.325,0.35,0.375,0.4,0.425,
0.45,0.475,0.5,0.525,0.55,0.575,0.6,0.625,0.65,0.675,0.7,0.725,0.75,0.775,
0.8,0.825,0.85,0.875,0.9,0.925,0.95,0.975,0.997113867990431),
 .UNSPECIFIED.)
CURVE()
GEOMETRIC_REPRESENTATION_ITEM()
RATIONAL_B_SPLINE_CURVE((0.998499781765884,0.998206929391006,1.,0.996917333733128,
1.,0.996917333733128,1.,0.996917333733128,1.,0.996917333733128,1.,0.996917333733128,
1.,0.996917333733128,1.,0.996917333733128,1.,0.996917333733128,1.,0.996917333733128,
1.,0.996917333733128,1.,0.996917333733128,1.,0.996917333733128,1.,0.996917333733128,
1.,0.996917333733128,1.,0.996917333733128,1.,0.996917333733128,1.,0.996917333733128,
1.,0.996917333733128,1.,0.996917333733128,1.,0.996917333733128,1.,0.996917333733128,
1.,0.996917333733128,1.,0.996917333733128,1.,0.996917333733128,1.,0.996917333733128,
1.,0.996917333733128,1.,0.996917333733128,1.,0.996917333733128,1.,0.996917333733128,
1.,0.996917333733128,1.,0.996917333733128,1.,0.996917333733128,1.,0.996917333733128,
1.,0.996917333733128,1.,0.996917333733128,1.,0.996917333733128,1.,0.996917333733128,
1.,0.996917333733128,1.,0.997273213004634,0.999370410621552))
REPRESENTATION_ITEM('')
);
#4172=(
BOUNDED_CURVE()
B_SPLINE_CURVE(2,(#271452,#271453,#271454,#271455,#271456,#271457,#271458,
#271459,#271460,#271461,#271462,#271463,#271464,#271465,#271466,#271467,
#271468,#271469,#271470,#271471,#271472,#271473,#271474,#271475,#271476,
#271477,#271478,#271479,#271480,#271481,#271482,#271483,#271484,#271485,
#271486,#271487,#271488,#271489,#271490,#271491,#271492,#271493,#271494,
#271495,#271496,#271497,#271498,#271499,#271500,#271501,#271502,#271503,
#271504,#271505,#271506,#271507,#271508,#271509,#271510,#271511,#271512,
#271513,#271514,#271515,#271516,#271517,#271518,#271519,#271520,#271521,
#271522,#271523,#271524,#271525,#271526,#271527,#271528,#271529,#271530,
#271531,#271532),.UNSPECIFIED.,.F.,.F.)
B_SPLINE_CURVE_WITH_KNOTS((3,2,2,2,2,2,2,2,2,2,2,2,2,2,2,2,2,2,2,2,2,2,
2,2,2,2,2,2,2,2,2,2,2,2,2,2,2,2,2,2,3),(0.00288613200956948,0.025,0.05,
0.075,0.1,0.125,0.15,0.175,0.2,0.225,0.25,0.275,0.3,0.325,0.35,0.375,0.4,
0.425,0.45,0.475,0.5,0.525,0.55,0.575,0.6,0.625,0.65,0.675,0.7,0.725,0.75,
0.775,0.8,0.825,0.85,0.875,0.9,0.925,0.95,0.975,0.98954155634899),
 .UNSPECIFIED.)
CURVE()
GEOMETRIC_REPRESENTATION_ITEM()
RATIONAL_B_SPLINE_CURVE((0.999370410621552,0.997273213004634,1.,0.996917333733128,
1.,0.996917333733128,1.,0.996917333733128,1.,0.996917333733128,1.,0.996917333733128,
1.,0.996917333733128,1.,0.996917333733128,1.,0.996917333733128,1.,0.996917333733128,
1.,0.996917333733128,1.,0.996917333733128,1.,0.996917333733128,1.,0.996917333733128,
1.,0.996917333733128,1.,0.996917333733128,1.,0.996917333733128,1.,0.996917333733128,
1.,0.996917333733128,1.,0.996917333733128,1.,0.996917333733128,1.,0.996917333733128,
1.,0.996917333733128,1.,0.996917333733128,1.,0.996917333733128,1.,0.996917333733128,
1.,0.996917333733128,1.,0.996917333733128,1.,0.996917333733128,1.,0.996917333733128,
1.,0.996917333733128,1.,0.996917333733128,1.,0.996917333733128,1.,0.996917333733128,
1.,0.996917333733128,1.,0.996917333733128,1.,0.996917333733128,1.,0.996917333733128,
1.,0.996917333733128,1.,0.998206929391006,0.998499781765884))
REPRESENTATION_ITEM('')
);
#5393=B_SPLINE_CURVE_WITH_KNOTS('',3,(#265324,#265325,#265326,#265327,#265328,
#265329,#265330,#265331),.UNSPECIFIED.,.F.,.F.,(4,2,2,4),(0.,2.02488294737315,
3.03870599509108,4.05123165236865),.UNSPECIFIED.);
#5394=B_SPLINE_CURVE_WITH_KNOTS('',3,(#265681,#265682,#265683,#265684,#265685,
#265686,#265687,#265688),.UNSPECIFIED.,.F.,.F.,(4,2,2,4),(0.,0.862850707214511,
1.72670633018526,3.45306151607852),.UNSPECIFIED.);
#5395=B_SPLINE_CURVE_WITH_KNOTS('',3,(#266028,#266029,#266030,#266031,#266032,
#266033,#266034,#266035),.UNSPECIFIED.,.F.,.F.,(4,2,2,4),(0.,0.862850707214148,
1.72670633018495,3.45306151607877),.UNSPECIFIED.);
#5396=B_SPLINE_CURVE_WITH_KNOTS('',3,(#266387,#266388,#266389,#266390,#266391,
#266392,#266393,#266394),.UNSPECIFIED.,.F.,.F.,(4,2,2,4),(0.,2.02488294737321,
3.03870599509107,4.05123165236849),.UNSPECIFIED.);
#5397=B_SPLINE_CURVE_WITH_KNOTS('',3,(#266579,#266580,#266581,#266582,#266583,
#266584,#266585,#266586,#266587,#266588,#266589,#266590,#266591,#266592,
#266593,#266594,#266595,#266596,#266597,#266598,#266599,#266600,#266601,
#266602,#266603,#266604,#266605,#266606,#266607,#266608,#266609,#266610,
#266611,#266612),.UNSPECIFIED.,.T.,.F.,(4,2,2,2,2,2,2,2,2,2,2,2,2,2,2,2,
4),(-4.61268662524521,-4.32400022458411,-4.03531382392301,-3.74741439642846,
-3.4595149689339,-3.17161554143936,-2.88371611394482,-2.59502971328371,
-2.30634331262261,-2.0176569119615,-1.7289705113004,-1.44107108380585,-1.15317165631131,
-0.865272228816758,-0.577372801322204,-0.288686400661102,0.),
 .UNSPECIFIED.);
#5398=B_SPLINE_CURVE_WITH_KNOTS('',3,(#266618,#266619,#266620,#266621,#266622,
#266623),.UNSPECIFIED.,.F.,.F.,(4,2,4),(0.,1.49684231771425,2.9926077413886),
 .UNSPECIFIED.);
#5399=B_SPLINE_CURVE_WITH_KNOTS('',3,(#266625,#266626,#266627,#266628,#266629,
#266630,#266631,#266632,#266633,#266634),.UNSPECIFIED.,.F.,.F.,(4,2,2,2,
4),(0.,0.176967107626664,0.344626505766095,0.512071202888707,0.688806050530056),
 .UNSPECIFIED.);
#5400=B_SPLINE_CURVE_WITH_KNOTS('',3,(#266636,#266637,#266638,#266639,#266640,
#266641),.UNSPECIFIED.,.F.,.F.,(4,2,4),(0.,1.49683920424661,2.99526264517898),
 .UNSPECIFIED.);
#5401=B_SPLINE_CURVE_WITH_KNOTS('',3,(#266642,#266643,#266644,#266645,#266646,
#266647,#266648,#266649,#266650,#266651),.UNSPECIFIED.,.F.,.F.,(4,2,2,2,
4),(0.,0.168709295937694,0.329326671396797,0.489872998360341,0.65852259063737),
 .UNSPECIFIED.);
#5402=B_SPLINE_CURVE_WITH_KNOTS('',3,(#266655,#266656,#266657,#266658,#266659,
#266660,#266661,#266662,#266663,#266664,#266665,#266666,#266667,#266668,
#266669,#266670,#266671,#266672,#266673),.UNSPECIFIED.,.F.,.F.,(4,2,2,2,
3,2,2,2,4),(-1.1531716563113,-0.86527222881675,-0.577372801322203,-0.288686400661101,
1.77635683940025E-15,0.288686400661104,0.577372801322206,0.865272228816754,
1.1531716563113),.UNSPECIFIED.);
#5403=B_SPLINE_CURVE_WITH_KNOTS('',3,(#266677,#266678,#266679,#266680,#266681,
#266682,#266683,#266684,#266685,#266686,#266687,#266688,#266689,#266690,
#266691,#266692,#266693,#266694),.UNSPECIFIED.,.F.,.F.,(4,2,2,2,2,2,2,2,
4),(1.1531716563113,1.44107108380585,1.7289705113004,2.0176569119615,2.3063433126226,
2.59502971328371,2.88371611394481,3.17161554143936,3.45951496893391),
 .UNSPECIFIED.);
#5404=B_SPLINE_CURVE_WITH_KNOTS('',3,(#266697,#266698,#266699,#266700,#266701,
#266702),.UNSPECIFIED.,.F.,.F.,(4,2,4),(0.,1.496842317777,2.99260774148207),
 .UNSPECIFIED.);
#5405=B_SPLINE_CURVE_WITH_KNOTS('',3,(#266704,#266705,#266706,#266707,#266708,
#266709,#266710,#266711,#266712,#266713),.UNSPECIFIED.,.F.,.F.,(4,2,2,2,
4),(0.,0.176967107626414,0.34462650576522,0.512071202887293,0.688806050528579),
 .UNSPECIFIED.);
#5406=B_SPLINE_CURVE_WITH_KNOTS('',3,(#266715,#266716,#266717,#266718,#266719,
#266720),.UNSPECIFIED.,.F.,.F.,(4,2,4),(0.,1.49683920424566,2.99526264511799),
 .UNSPECIFIED.);
#5407=B_SPLINE_CURVE_WITH_KNOTS('',3,(#266721,#266722,#266723,#266724,#266725,
#266726,#266727,#266728,#266729,#266730),.UNSPECIFIED.,.F.,.F.,(4,2,2,2,
4),(0.,0.168709295937647,0.329326671396668,0.489872998360253,0.658522590637766),
 .UNSPECIFIED.);
#5408=B_SPLINE_CURVE_WITH_KNOTS('',3,(#266734,#266735,#266736,#266737,#266738,
#266739,#266740,#266741,#266742,#266743,#266744,#266745,#266746,#266747,
#266748,#266749,#266750,#266751),.UNSPECIFIED.,.F.,.F.,(4,2,2,2,2,2,2,2,
4),(1.1531716563113,1.44107108380585,1.7289705113004,2.01765691196151,2.30634331262261,
2.59502971328371,2.88371611394481,3.17161554143937,3.45951496893392),
 .UNSPECIFIED.);
#5409=B_SPLINE_CURVE_WITH_KNOTS('',3,(#266755,#266756,#266757,#266758,#266759,
#266760,#266761,#266762,#266763,#266764,#266765,#266766,#266767,#266768,
#266769,#266770,#266771,#266772,#266773),.UNSPECIFIED.,.F.,.F.,(4,2,2,2,
3,2,2,2,4),(3.45951496893392,3.74741439642846,4.035313823923,4.32400022458411,
4.61268662524521,4.90137302590632,5.19005942656742,5.47795885406197,5.76585828155651),
 .UNSPECIFIED.);
#5410=B_SPLINE_CURVE_WITH_KNOTS('',3,(#266776,#266777,#266778,#266779,#266780,
#266781,#266782,#266783,#266784,#266785),.UNSPECIFIED.,.F.,.F.,(4,2,2,2,
4),(-0.658522598895983,-0.489809349878546,-0.32920232171901,-0.168645651361104,
0.),.UNSPECIFIED.);
#5411=B_SPLINE_CURVE_WITH_KNOTS('',3,(#266787,#266788,#266789,#266790,#266791,
#266792),.UNSPECIFIED.,.F.,.F.,(4,2,4),(-2.99260774139286,-1.49684228178934,
0.),.UNSPECIFIED.);
#5412=B_SPLINE_CURVE_WITH_KNOTS('',3,(#266794,#266795,#266796,#266797,#266798,
#266799,#266800,#266801,#266802,#266803),.UNSPECIFIED.,.F.,.F.,(4,2,2,2,
4),(-0.688806220570509,-0.51183539502754,-0.344166623478192,-0.176731189784664,
0.),.UNSPECIFIED.);
#5413=B_SPLINE_CURVE_WITH_KNOTS('',3,(#266804,#266805,#266806,#266807,#266808,
#266809),.UNSPECIFIED.,.F.,.F.,(4,2,4),(-2.99526264006051,-1.49683924471816,
0.),.UNSPECIFIED.);
#5414=B_SPLINE_CURVE_WITH_KNOTS('',3,(#266813,#266814,#266815,#266816,#266817,
#266818,#266819,#266820,#266821,#266822,#266823,#266824,#266825,#266826,
#266827,#266828,#266829,#266830),.UNSPECIFIED.,.F.,.F.,(4,2,2,2,2,2,2,2,
4),(1.15317165631131,1.44107108380585,1.7289705113004,2.0176569119615,2.30634331262261,
2.59502971328371,2.88371611394481,3.17161554143936,3.4595149689339),
 .UNSPECIFIED.);
#5415=B_SPLINE_CURVE_WITH_KNOTS('',3,(#266834,#266835,#266836,#266837,#266838,
#266839,#266840,#266841,#266842,#266843,#266844,#266845,#266846,#266847,
#266848,#266849,#266850,#266851,#266852),.UNSPECIFIED.,.F.,.F.,(4,2,2,2,
3,2,2,2,4),(-1.1531716563113,-0.865272228816753,-0.577372801322205,-0.288686400661102,
1.55431223447522E-15,0.288686400661105,0.577372801322209,0.865272228816757,
1.15317165631131),.UNSPECIFIED.);
#5416=B_SPLINE_CURVE_WITH_KNOTS('',3,(#266855,#266856,#266857,#266858,#266859,
#266860,#266861,#266862,#266863,#266864),.UNSPECIFIED.,.F.,.F.,(4,2,2,2,
4),(-0.688806220570527,-0.511835395027638,-0.344166623478395,-0.17673118978486,
0.),.UNSPECIFIED.);
#5417=B_SPLINE_CURVE_WITH_KNOTS('',3,(#266866,#266867,#266868,#266869,#266870,
#266871),.UNSPECIFIED.,.F.,.F.,(4,2,4),(-2.99526263988214,-1.49683924469841,
0.),.UNSPECIFIED.);
#5418=B_SPLINE_CURVE_WITH_KNOTS('',3,(#266873,#266874,#266875,#266876,#266877,
#266878,#266879,#266880,#266881,#266882),.UNSPECIFIED.,.F.,.F.,(4,2,2,2,
4),(-0.658522598898453,-0.489809349881006,-0.3292023217204,-0.168645651361312,
0.),.UNSPECIFIED.);
#5419=B_SPLINE_CURVE_WITH_KNOTS('',3,(#266883,#266884,#266885,#266886,#266887,
#266888),.UNSPECIFIED.,.F.,.F.,(4,2,4),(-2.99260774142664,-1.49684228180428,
0.),.UNSPECIFIED.);
#5420=B_SPLINE_CURVE_WITH_KNOTS('',3,(#266892,#266893,#266894,#266895,#266896,
#266897,#266898,#266899,#266900,#266901,#266902,#266903,#266904,#266905,
#266906,#266907,#266908,#266909),.UNSPECIFIED.,.F.,.F.,(4,2,2,2,2,2,2,2,
4),(-3.4595149689339,-3.17161554143936,-2.88371611394481,-2.59502971328371,
-2.3063433126226,-2.0176569119615,-1.7289705113004,-1.44107108380585,-1.1531716563113),
 .UNSPECIFIED.);
#5421=B_SPLINE_CURVE_WITH_KNOTS('',3,(#266913,#266914,#266915,#266916,#266917,
#266918,#266919,#266920,#266921,#266922,#266923,#266924,#266925,#266926,
#266927,#266928,#266929,#266930,#266931),.UNSPECIFIED.,.F.,.F.,(4,2,2,2,
3,2,2,2,4),(-1.1531716563113,-0.865272228816754,-0.577372801322206,-0.288686400661103,
0.,0.288686400661104,0.577372801322206,0.865272228816754,1.1531716563113),
 .UNSPECIFIED.);
#5422=B_SPLINE_CURVE_WITH_KNOTS('',3,(#266934,#266935,#266936,#266937,#266938,
#266939),.UNSPECIFIED.,.F.,.F.,(4,2,4),(0.,1.49683920421981,2.99526264506199),
 .UNSPECIFIED.);
#5423=B_SPLINE_CURVE_WITH_KNOTS('',3,(#266941,#266942,#266943,#266944,#266945,
#266946,#266947,#266948,#266949,#266950),.UNSPECIFIED.,.F.,.F.,(4,2,2,2,
4),(0.,0.168709295937734,0.329326671397018,0.48987299836074,0.658522590638148),
 .UNSPECIFIED.);
#5424=B_SPLINE_CURVE_WITH_KNOTS('',3,(#266952,#266953,#266954,#266955,#266956,
#266957),.UNSPECIFIED.,.F.,.F.,(4,2,4),(0.,1.49684231774429,2.99260774143943),
 .UNSPECIFIED.);
#5425=B_SPLINE_CURVE_WITH_KNOTS('',3,(#266958,#266959,#266960,#266961,#266962,
#266963,#266964,#266965,#266966,#266967),.UNSPECIFIED.,.F.,.F.,(4,2,2,2,
4),(0.,0.176967107626893,0.344626505766581,0.512071202889326,0.688806050530784),
 .UNSPECIFIED.);
#5426=B_SPLINE_CURVE_WITH_KNOTS('',3,(#266970,#266971,#266972,#266973,#266974,
#266975,#266976,#266977,#266978,#266979),.UNSPECIFIED.,.F.,.F.,(4,2,2,2,
4),(-0.658522598896504,-0.489809349878851,-0.329202321719165,-0.168645651361139,
0.),.UNSPECIFIED.);
#5427=B_SPLINE_CURVE_WITH_KNOTS('',3,(#266981,#266982,#266983,#266984,#266985,
#266986),.UNSPECIFIED.,.F.,.F.,(4,2,4),(-2.99260774147142,-1.49684228182412,
0.),.UNSPECIFIED.);
#5428=B_SPLINE_CURVE_WITH_KNOTS('',3,(#266988,#266989,#266990,#266991,#266992,
#266993,#266994,#266995,#266996,#266997),.UNSPECIFIED.,.F.,.F.,(4,2,2,2,
4),(-0.688806220566902,-0.511835395024936,-0.344166623476774,-0.176731189784255,
0.),.UNSPECIFIED.);
#5429=B_SPLINE_CURVE_WITH_KNOTS('',3,(#266998,#266999,#267000,#267001,#267002,
#267003),.UNSPECIFIED.,.F.,.F.,(4,2,4),(-2.9952626398682,-1.49683924471003,
0.),.UNSPECIFIED.);
#5430=B_SPLINE_CURVE_WITH_KNOTS('',3,(#267007,#267008,#267009,#267010,#267011,
#267012,#267013,#267014,#267015,#267016,#267017,#267018,#267019,#267020,
#267021,#267022,#267023,#267024,#267025),.UNSPECIFIED.,.F.,.F.,(4,2,2,2,
3,2,2,2,4),(3.4595149689339,3.74741439642845,4.035313823923,4.3240002245841,
4.61268662524521,4.90137302590631,5.19005942656741,5.47795885406196,5.76585828155651),
 .UNSPECIFIED.);
#5431=B_SPLINE_CURVE_WITH_KNOTS('',3,(#267029,#267030,#267031,#267032,#267033,
#267034,#267035,#267036,#267037,#267038,#267039,#267040,#267041,#267042,
#267043,#267044,#267045,#267046),.UNSPECIFIED.,.F.,.F.,(4,2,2,2,2,2,2,2,
4),(5.76585828155651,6.05375770905105,6.3416571365456,6.6303435372067,6.91902993786781,
7.20771633852891,7.49640273919001,7.78430216668456,8.07220159417911),
 .UNSPECIFIED.);
#5432=B_SPLINE_CURVE_WITH_KNOTS('',3,(#267049,#267050,#267051,#267052,#267053,
#267054),.UNSPECIFIED.,.F.,.F.,(4,2,4),(0.,1.49684231777726,2.99260774149539),
 .UNSPECIFIED.);
#5433=B_SPLINE_CURVE_WITH_KNOTS('',3,(#267056,#267057,#267058,#267059,#267060,
#267061,#267062,#267063,#267064,#267065),.UNSPECIFIED.,.F.,.F.,(4,2,2,2,
4),(0.,0.176967107626481,0.344626505765638,0.512071202888007,0.688806050529249),
 .UNSPECIFIED.);
#5434=B_SPLINE_CURVE_WITH_KNOTS('',3,(#267067,#267068,#267069,#267070,#267071,
#267072),.UNSPECIFIED.,.F.,.F.,(4,2,4),(0.,1.49683920427303,2.9952626452325),
 .UNSPECIFIED.);
#5435=B_SPLINE_CURVE_WITH_KNOTS('',3,(#267073,#267074,#267075,#267076,#267077,
#267078,#267079,#267080,#267081,#267082),.UNSPECIFIED.,.F.,.F.,(4,2,2,2,
4),(0.,0.168709295937688,0.329326671396385,0.489872998359487,0.658522590636729),
 .UNSPECIFIED.);
#5436=B_SPLINE_CURVE_WITH_KNOTS('',3,(#267085,#267086,#267087,#267088,#267089,
#267090,#267091,#267092,#267093,#267094),.UNSPECIFIED.,.F.,.F.,(4,2,2,2,
4),(-0.688806220572771,-0.511835395028998,-0.34416662347923,-0.176731189785183,
0.),.UNSPECIFIED.);
#5437=B_SPLINE_CURVE_WITH_KNOTS('',3,(#267096,#267097,#267098,#267099,#267100,
#267101),.UNSPECIFIED.,.F.,.F.,(4,2,4),(-2.99526263994789,-1.49683924471765,
0.),.UNSPECIFIED.);
#5438=B_SPLINE_CURVE_WITH_KNOTS('',3,(#267103,#267104,#267105,#267106,#267107,
#267108,#267109,#267110,#267111,#267112),.UNSPECIFIED.,.F.,.F.,(4,2,2,2,
4),(-0.658522598893829,-0.489809349877018,-0.329202321717993,-0.168645651360644,
0.),.UNSPECIFIED.);
#5439=B_SPLINE_CURVE_WITH_KNOTS('',3,(#267113,#267114,#267115,#267116,#267117,
#267118),.UNSPECIFIED.,.F.,.F.,(4,2,4),(-2.99260774145968,-1.496842281811,
0.),.UNSPECIFIED.);
#5440=B_SPLINE_CURVE_WITH_KNOTS('',3,(#268102,#268103,#268104,#268105,#268106,
#268107,#268108),.UNSPECIFIED.,.F.,.F.,(4,3,4),(-8.06482196325813E-5,0.,
0.00573600054306479),.UNSPECIFIED.);
#5441=B_SPLINE_CURVE_WITH_KNOTS('',3,(#268112,#268113,#268114,#268115),
 .UNSPECIFIED.,.F.,.F.,(4,4),(0.,0.00872457834628637),.UNSPECIFIED.);
#5442=B_SPLINE_CURVE_WITH_KNOTS('',3,(#268116,#268117,#268118,#268119,#268120,
#268121,#268122),.UNSPECIFIED.,.F.,.F.,(4,3,4),(4.79067216416971E-16,0.00573600054306518,
0.00581664876269783),.UNSPECIFIED.);
#5443=B_SPLINE_CURVE_WITH_KNOTS('',3,(#268125,#268126,#268127,#268128),
 .UNSPECIFIED.,.F.,.F.,(4,4),(0.,0.0087245783462611),.UNSPECIFIED.);
#5444=B_SPLINE_CURVE_WITH_KNOTS('',3,(#271700,#271701,#271702,#271703),
 .UNSPECIFIED.,.F.,.F.,(4,4),(0.,0.00872457834628661),.UNSPECIFIED.);
#5445=B_SPLINE_CURVE_WITH_KNOTS('',3,(#271704,#271705,#271706,#271707,#271708,
#271709,#271710),.UNSPECIFIED.,.F.,.F.,(4,3,4),(-8.0648219632873E-5,0.,
0.00573600054306445),.UNSPECIFIED.);
#5446=B_SPLINE_CURVE_WITH_KNOTS('',3,(#271714,#271715,#271716,#271717),
 .UNSPECIFIED.,.F.,.F.,(4,4),(0.,0.008724578346262),.UNSPECIFIED.);
#5447=B_SPLINE_CURVE_WITH_KNOTS('',3,(#271718,#271719,#271720,#271721,#271722,
#271723,#271724),.UNSPECIFIED.,.F.,.F.,(4,3,4),(1.81429262580847E-14,0.00573600054306257,
0.00581664876269541),.UNSPECIFIED.);
#5448=B_SPLINE_CURVE_WITH_KNOTS('',3,(#272380,#272381,#272382,#272383),
 .UNSPECIFIED.,.F.,.F.,(4,4),(9.54097911787244E-18,0.00872457834626197),
 .UNSPECIFIED.);
#5449=B_SPLINE_CURVE_WITH_KNOTS('',3,(#272384,#272385,#272386,#272387,#272388,
#272389,#272390),.UNSPECIFIED.,.F.,.F.,(4,3,4),(0.,0.00573600054306478,
0.00581664876269765),.UNSPECIFIED.);
#5450=B_SPLINE_CURVE_WITH_KNOTS('',3,(#272719,#272720,#272721,#272722),
 .UNSPECIFIED.,.F.,.F.,(4,4),(0.,0.00872457834628667),.UNSPECIFIED.);
#5451=B_SPLINE_CURVE_WITH_KNOTS('',3,(#272724,#272725,#272726,#272727,#272728,
#272729,#272730),.UNSPECIFIED.,.F.,.F.,(4,3,4),(6.2375853683061E-16,0.00573600054306585,
0.00581664876269842),.UNSPECIFIED.);
#5452=B_SPLINE_CURVE_WITH_KNOTS('',3,(#273060,#273061,#273062,#273063,#273064,
#273065,#273066),.UNSPECIFIED.,.F.,.F.,(4,3,4),(-8.06482196327907E-5,0.,
0.00573600054306464),.UNSPECIFIED.);
#5453=B_SPLINE_CURVE_WITH_KNOTS('',3,(#273069,#273070,#273071,#273072),
 .UNSPECIFIED.,.F.,.F.,(4,4),(0.,0.0087245783462611),.UNSPECIFIED.);
#5454=B_SPLINE_CURVE_WITH_KNOTS('',3,(#273401,#273402,#273403,#273404,#273405,
#273406,#273407),.UNSPECIFIED.,.F.,.F.,(4,3,4),(-8.06482196325413E-5,0.,
0.00573600054306597),.UNSPECIFIED.);
#5455=B_SPLINE_CURVE_WITH_KNOTS('',3,(#273410,#273411,#273412,#273413),
 .UNSPECIFIED.,.F.,.F.,(4,4),(0.,0.00872457834628645),.UNSPECIFIED.);
#5463=SHAPE_REPRESENTATION_RELATIONSHIP('SRR','None',#276491,#5469);
#5469=ADVANCED_BREP_SHAPE_REPRESENTATION('',(#5525,#5526,#5527),#276459);
#5496=STYLED_ITEM('',(#276530),#5525);
#5497=STYLED_ITEM('',(#276530),#5526);
#5498=STYLED_ITEM('',(#276530),#5527);
#5525=MANIFOLD_SOLID_BREP('Body1',#98721);
#5526=MANIFOLD_SOLID_BREP('Body2',#98722);
#5527=MANIFOLD_SOLID_BREP('Body3',#98723);
#6425=FACE_BOUND('',#19429,.T.);
#6426=FACE_BOUND('',#19431,.T.);
#6427=FACE_BOUND('',#19433,.T.);
#6428=FACE_BOUND('',#19435,.T.);
#6429=FACE_BOUND('',#19437,.T.);
#6430=FACE_BOUND('',#19438,.T.);
#6431=FACE_BOUND('',#19440,.T.);
#6432=FACE_BOUND('',#19441,.T.);
#6433=FACE_BOUND('',#19443,.T.);
#6434=FACE_BOUND('',#19444,.T.);
#6435=FACE_BOUND('',#19450,.T.);
#6436=FACE_BOUND('',#19468,.T.);
#6437=FACE_BOUND('',#19474,.T.);
#6438=FACE_BOUND('',#19478,.T.);
#6439=FACE_BOUND('',#19482,.T.);
#6440=FACE_BOUND('',#19486,.T.);
#6441=FACE_BOUND('',#19490,.T.);
#7316=PLANE('',#110835);
#7317=PLANE('',#110836);
#7318=PLANE('',#110837);
#7319=PLANE('',#110838);
#7320=PLANE('',#110859);
#7321=PLANE('',#110862);
#7322=PLANE('',#110865);
#7323=PLANE('',#110867);
#7324=PLANE('',#110869);
#7325=PLANE('',#110871);
#7326=PLANE('',#110873);
#7327=PLANE('',#110874);
#13201=FACE_OUTER_BOUND('',#19414,.T.);
#13202=FACE_OUTER_BOUND('',#19415,.T.);
#13203=FACE_OUTER_BOUND('',#19416,.T.);
#13204=FACE_OUTER_BOUND('',#19417,.T.);
#13205=FACE_OUTER_BOUND('',#19418,.T.);
#13206=FACE_OUTER_BOUND('',#19419,.T.);
#13207=FACE_OUTER_BOUND('',#19420,.T.);
#13208=FACE_OUTER_BOUND('',#19421,.T.);
#13209=FACE_OUTER_BOUND('',#19422,.T.);
#13210=FACE_OUTER_BOUND('',#19423,.T.);
#13211=FACE_OUTER_BOUND('',#19424,.T.);
#13212=FACE_OUTER_BOUND('',#19425,.T.);
#13213=FACE_OUTER_BOUND('',#19426,.T.);
#13214=FACE_OUTER_BOUND('',#19427,.T.);
#13215=FACE_OUTER_BOUND('',#19428,.T.);
#13216=FACE_OUTER_BOUND('',#19430,.T.);
#13217=FACE_OUTER_BOUND('',#19432,.T.);
#13218=FACE_OUTER_BOUND('',#19434,.T.);
#13219=FACE_OUTER_BOUND('',#19436,.T.);
#13220=FACE_OUTER_BOUND('',#19439,.T.);
#13221=FACE_OUTER_BOUND('',#19442,.T.);
#13222=FACE_OUTER_BOUND('',#19445,.T.);
#13223=FACE_OUTER_BOUND('',#19446,.T.);
#13224=FACE_OUTER_BOUND('',#19447,.T.);
#13225=FACE_OUTER_BOUND('',#19448,.T.);
#13226=FACE_OUTER_BOUND('',#19449,.T.);
#13227=FACE_OUTER_BOUND('',#19451,.T.);
#13228=FACE_OUTER_BOUND('',#19452,.T.);
#13229=FACE_OUTER_BOUND('',#19453,.T.);
#13230=FACE_OUTER_BOUND('',#19454,.T.);
#13231=FACE_OUTER_BOUND('',#19455,.T.);
#13232=FACE_OUTER_BOUND('',#19456,.T.);
#13233=FACE_OUTER_BOUND('',#19457,.T.);
#13234=FACE_OUTER_BOUND('',#19458,.T.);
#13235=FACE_OUTER_BOUND('',#19459,.T.);
#13236=FACE_OUTER_BOUND('',#19460,.T.);
#13237=FACE_OUTER_BOUND('',#19461,.T.);
#13238=FACE_OUTER_BOUND('',#19462,.T.);
#13239=FACE_OUTER_BOUND('',#19463,.T.);
#13240=FACE_OUTER_BOUND('',#19464,.T.);
#13241=FACE_OUTER_BOUND('',#19465,.T.);
#13242=FACE_OUTER_BOUND('',#19466,.T.);
#13243=FACE_OUTER_BOUND('',#19467,.T.);
#13244=FACE_OUTER_BOUND('',#19469,.T.);
#13245=FACE_OUTER_BOUND('',#19470,.T.);
#13246=FACE_OUTER_BOUND('',#19471,.T.);
#13247=FACE_OUTER_BOUND('',#19472,.T.);
#13248=FACE_OUTER_BOUND('',#19473,.T.);
#13249=FACE_OUTER_BOUND('',#19475,.T.);
#13250=FACE_OUTER_BOUND('',#19476,.T.);
#13251=FACE_OUTER_BOUND('',#19477,.T.);
#13252=FACE_OUTER_BOUND('',#19479,.T.);
#13253=FACE_OUTER_BOUND('',#19480,.T.);
#13254=FACE_OUTER_BOUND('',#19481,.T.);
#13255=FACE_OUTER_BOUND('',#19483,.T.);
#13256=FACE_OUTER_BOUND('',#19484,.T.);
#13257=FACE_OUTER_BOUND('',#19485,.T.);
#13258=FACE_OUTER_BOUND('',#19487,.T.);
#13259=FACE_OUTER_BOUND('',#19488,.T.);
#13260=FACE_OUTER_BOUND('',#19489,.T.);
#13261=FACE_OUTER_BOUND('',#19491,.T.);
#19414=EDGE_LOOP('',(#87459,#87460,#87461,#87462));
#19415=EDGE_LOOP('',(#87463,#87464,#87465,#87466));
#19416=EDGE_LOOP('',(#87467,#87468,#87469,#87470));
#19417=EDGE_LOOP('',(#87471,#87472,#87473,#87474));
#19418=EDGE_LOOP('',(#87475,#87476,#87477,#87478));
#19419=EDGE_LOOP('',(#87479,#87480,#87481,#87482));
#19420=EDGE_LOOP('',(#87483,#87484,#87485,#87486));
#19421=EDGE_LOOP('',(#87487,#87488,#87489,#87490));
#19422=EDGE_LOOP('',(#87491,#87492,#87493,#87494));
#19423=EDGE_LOOP('',(#87495,#87496,#87497,#87498));
#19424=EDGE_LOOP('',(#87499,#87500,#87501,#87502));
#19425=EDGE_LOOP('',(#87503,#87504,#87505,#87506));
#19426=EDGE_LOOP('',(#87507,#87508,#87509,#87510));
#19427=EDGE_LOOP('',(#87511,#87512,#87513));
#19428=EDGE_LOOP('',(#87514,#87515,#87516,#87517));
#19429=EDGE_LOOP('',(#87518,#87519,#87520,#87521));
#19430=EDGE_LOOP('',(#87522,#87523,#87524,#87525,#87526));
#19431=EDGE_LOOP('',(#87527,#87528,#87529,#87530));
#19432=EDGE_LOOP('',(#87531,#87532,#87533,#87534,#87535));
#19433=EDGE_LOOP('',(#87536,#87537,#87538,#87539));
#19434=EDGE_LOOP('',(#87540,#87541,#87542,#87543,#87544));
#19435=EDGE_LOOP('',(#87545,#87546,#87547,#87548));
#19436=EDGE_LOOP('',(#87549,#87550,#87551,#87552,#87553));
#19437=EDGE_LOOP('',(#87554,#87555,#87556,#87557));
#19438=EDGE_LOOP('',(#87558,#87559,#87560,#87561));
#19439=EDGE_LOOP('',(#87562,#87563,#87564,#87565,#87566));
#19440=EDGE_LOOP('',(#87567,#87568,#87569,#87570));
#19441=EDGE_LOOP('',(#87571,#87572,#87573,#87574));
#19442=EDGE_LOOP('',(#87575,#87576,#87577,#87578,#87579,#87580,#87581,#87582,
#87583,#87584,#87585,#87586,#87587,#87588,#87589,#87590,#87591));
#19443=EDGE_LOOP('',(#87592));
#19444=EDGE_LOOP('',(#87593,#87594));
#19445=EDGE_LOOP('',(#87595,#87596,#87597,#87598));
#19446=EDGE_LOOP('',(#87599,#87600,#87601,#87602));
#19447=EDGE_LOOP('',(#87603,#87604,#87605,#87606));
#19448=EDGE_LOOP('',(#87607,#87608,#87609,#87610));
#19449=EDGE_LOOP('',(#87611));
#19450=EDGE_LOOP('',(#87612,#87613,#87614,#87615,#87616,#87617));
#19451=EDGE_LOOP('',(#87618,#87619,#87620));
#19452=EDGE_LOOP('',(#87621,#87622));
#19453=EDGE_LOOP('',(#87623,#87624));
#19454=EDGE_LOOP('',(#87625,#87626,#87627));
#19455=EDGE_LOOP('',(#87628,#87629,#87630,#87631));
#19456=EDGE_LOOP('',(#87632,#87633,#87634,#87635));
#19457=EDGE_LOOP('',(#87636,#87637,#87638,#87639));
#19458=EDGE_LOOP('',(#87640,#87641,#87642,#87643));
#19459=EDGE_LOOP('',(#87644,#87645,#87646,#87647));
#19460=EDGE_LOOP('',(#87648,#87649,#87650,#87651));
#19461=EDGE_LOOP('',(#87652,#87653,#87654,#87655));
#19462=EDGE_LOOP('',(#87656,#87657,#87658,#87659));
#19463=EDGE_LOOP('',(#87660,#87661,#87662,#87663));
#19464=EDGE_LOOP('',(#87664,#87665,#87666,#87667));
#19465=EDGE_LOOP('',(#87668,#87669,#87670,#87671));
#19466=EDGE_LOOP('',(#87672,#87673,#87674,#87675));
#19467=EDGE_LOOP('',(#87676));
#19468=EDGE_LOOP('',(#87677,#87678,#87679,#87680,#87681,#87682));
#19469=EDGE_LOOP('',(#87683,#87684));
#19470=EDGE_LOOP('',(#87685,#87686,#87687));
#19471=EDGE_LOOP('',(#87688,#87689));
#19472=EDGE_LOOP('',(#87690,#87691,#87692));
#19473=EDGE_LOOP('',(#87693));
#19474=EDGE_LOOP('',(#87694,#87695,#87696));
#19475=EDGE_LOOP('',(#87697,#87698,#87699));
#19476=EDGE_LOOP('',(#87700,#87701));
#19477=EDGE_LOOP('',(#87702));
#19478=EDGE_LOOP('',(#87703,#87704,#87705));
#19479=EDGE_LOOP('',(#87706,#87707,#87708));
#19480=EDGE_LOOP('',(#87709,#87710));
#19481=EDGE_LOOP('',(#87711));
#19482=EDGE_LOOP('',(#87712,#87713,#87714));
#19483=EDGE_LOOP('',(#87715,#87716,#87717));
#19484=EDGE_LOOP('',(#87718,#87719));
#19485=EDGE_LOOP('',(#87720));
#19486=EDGE_LOOP('',(#87721,#87722,#87723));
#19487=EDGE_LOOP('',(#87724,#87725));
#19488=EDGE_LOOP('',(#87726,#87727,#87728));
#19489=EDGE_LOOP('',(#87729));
#19490=EDGE_LOOP('',(#87730));
#19491=EDGE_LOOP('',(#87731,#87732));
#24214=LINE('',#265339,#29441);
#24215=LINE('',#265510,#29442);
#24216=LINE('',#265517,#29443);
#24217=LINE('',#265697,#29444);
#24218=LINE('',#265860,#29445);
#24219=LINE('',#265861,#29446);
#24220=LINE('',#266045,#29447);
#24221=LINE('',#266214,#29448);
#24222=LINE('',#266223,#29449);
#24223=LINE('',#266401,#29450);
#24224=LINE('',#266564,#29451);
#24225=LINE('',#266565,#29452);
#24226=LINE('',#266572,#29453);
#24227=LINE('',#266576,#29454);
#24228=LINE('',#266614,#29455);
#24229=LINE('',#266675,#29456);
#24230=LINE('',#266753,#29457);
#24231=LINE('',#266832,#29458);
#24232=LINE('',#266911,#29459);
#24233=LINE('',#267027,#29460);
#24234=LINE('',#267121,#29461);
#24235=LINE('',#267122,#29462);
#24236=LINE('',#267124,#29463);
#24237=LINE('',#268110,#29464);
#24238=LINE('',#268124,#29465);
#24239=LINE('',#271698,#29466);
#24240=LINE('',#271712,#29467);
#24241=LINE('',#272378,#29468);
#24242=LINE('',#272731,#29469);
#24243=LINE('',#273068,#29470);
#24244=LINE('',#273409,#29471);
#29441=VECTOR('',#139995,1000.);
#29442=VECTOR('',#139996,10.);
#29443=VECTOR('',#139997,1000.);
#29444=VECTOR('',#139998,1000.);
#29445=VECTOR('',#139999,10.);
#29446=VECTOR('',#140000,1000.);
#29447=VECTOR('',#140005,1000.);
#29448=VECTOR('',#140006,10.);
#29449=VECTOR('',#140007,1000.);
#29450=VECTOR('',#140008,1000.);
#29451=VECTOR('',#140009,10.);
#29452=VECTOR('',#140010,1000.);
#29453=VECTOR('',#140019,3.4);
#29454=VECTOR('',#140024,3.4);
#29455=VECTOR('',#140027,7.49999999999995);
#29456=VECTOR('',#140032,7.49999999999995);
#29457=VECTOR('',#140037,7.49999999999995);
#29458=VECTOR('',#140042,7.49999999999995);
#29459=VECTOR('',#140047,7.49999999999995);
#29460=VECTOR('',#140052,7.49999999999995);
#29461=VECTOR('',#140059,15.);
#29462=VECTOR('',#140060,15.);
#29463=VECTOR('',#140061,15.);
#29464=VECTOR('',#140068,1000.);
#29465=VECTOR('',#140069,1000.);
#29466=VECTOR('',#140076,1000.);
#29467=VECTOR('',#140077,1000.);
#29468=VECTOR('',#140084,1000.);
#29469=VECTOR('',#140089,1000.);
#29470=VECTOR('',#140094,1000.);
#29471=VECTOR('',#140099,1000.);
#36204=CIRCLE('',#110840,3.4);
#36205=CIRCLE('',#110841,3.4);
#36206=CIRCLE('',#110844,7.49999999999995);
#36207=CIRCLE('',#110846,7.49999999999995);
#36208=CIRCLE('',#110848,7.49999999999995);
#36209=CIRCLE('',#110850,7.49999999999995);
#36210=CIRCLE('',#110852,7.49999999999995);
#36211=CIRCLE('',#110854,7.49999999999995);
#36212=CIRCLE('',#110856,15.);
#36213=CIRCLE('',#110857,15.);
#36214=CIRCLE('',#110858,15.);
#36215=CIRCLE('',#110860,164.1007636766);
#36216=CIRCLE('',#110861,164.100763676616);
#36217=CIRCLE('',#110863,164.100763676451);
#36218=CIRCLE('',#110864,164.100763676573);
#36219=CIRCLE('',#110866,164.100763676568);
#36220=CIRCLE('',#110868,164.100763676577);
#36221=CIRCLE('',#110870,164.100763676601);
#36222=CIRCLE('',#110872,164.100763676567);
#44556=VERTEX_POINT('',#265322);
#44557=VERTEX_POINT('',#265323);
#44558=VERTEX_POINT('',#265332);
#44559=VERTEX_POINT('',#265338);
#44560=VERTEX_POINT('',#265509);
#44561=VERTEX_POINT('',#265511);
#44562=VERTEX_POINT('',#265680);
#44563=VERTEX_POINT('',#265689);
#44564=VERTEX_POINT('',#266026);
#44565=VERTEX_POINT('',#266027);
#44566=VERTEX_POINT('',#266036);
#44567=VERTEX_POINT('',#266044);
#44568=VERTEX_POINT('',#266213);
#44569=VERTEX_POINT('',#266215);
#44570=VERTEX_POINT('',#266386);
#44571=VERTEX_POINT('',#266395);
#44572=VERTEX_POINT('',#266569);
#44573=VERTEX_POINT('',#266571);
#44574=VERTEX_POINT('',#266575);
#44575=VERTEX_POINT('',#266578);
#44576=VERTEX_POINT('',#266613);
#44577=VERTEX_POINT('',#266616);
#44578=VERTEX_POINT('',#266617);
#44579=VERTEX_POINT('',#266624);
#44580=VERTEX_POINT('',#266635);
#44581=VERTEX_POINT('',#266653);
#44582=VERTEX_POINT('',#266654);
#44583=VERTEX_POINT('',#266674);
#44584=VERTEX_POINT('',#266695);
#44585=VERTEX_POINT('',#266696);
#44586=VERTEX_POINT('',#266703);
#44587=VERTEX_POINT('',#266714);
#44588=VERTEX_POINT('',#266732);
#44589=VERTEX_POINT('',#266733);
#44590=VERTEX_POINT('',#266752);
#44591=VERTEX_POINT('',#266774);
#44592=VERTEX_POINT('',#266775);
#44593=VERTEX_POINT('',#266786);
#44594=VERTEX_POINT('',#266793);
#44595=VERTEX_POINT('',#266811);
#44596=VERTEX_POINT('',#266812);
#44597=VERTEX_POINT('',#266831);
#44598=VERTEX_POINT('',#266853);
#44599=VERTEX_POINT('',#266854);
#44600=VERTEX_POINT('',#266865);
#44601=VERTEX_POINT('',#266872);
#44602=VERTEX_POINT('',#266890);
#44603=VERTEX_POINT('',#266891);
#44604=VERTEX_POINT('',#266910);
#44605=VERTEX_POINT('',#266932);
#44606=VERTEX_POINT('',#266933);
#44607=VERTEX_POINT('',#266940);
#44608=VERTEX_POINT('',#266951);
#44609=VERTEX_POINT('',#266968);
#44610=VERTEX_POINT('',#266969);
#44611=VERTEX_POINT('',#266980);
#44612=VERTEX_POINT('',#266987);
#44613=VERTEX_POINT('',#267005);
#44614=VERTEX_POINT('',#267006);
#44615=VERTEX_POINT('',#267026);
#44616=VERTEX_POINT('',#267047);
#44617=VERTEX_POINT('',#267048);
#44618=VERTEX_POINT('',#267055);
#44619=VERTEX_POINT('',#267066);
#44620=VERTEX_POINT('',#267083);
#44621=VERTEX_POINT('',#267084);
#44622=VERTEX_POINT('',#267095);
#44623=VERTEX_POINT('',#267102);
#44624=VERTEX_POINT('',#267123);
#44625=VERTEX_POINT('',#268100);
#44626=VERTEX_POINT('',#268101);
#44627=VERTEX_POINT('',#268109);
#44628=VERTEX_POINT('',#268111);
#44629=VERTEX_POINT('',#268123);
#44630=VERTEX_POINT('',#271696);
#44631=VERTEX_POINT('',#271697);
#44632=VERTEX_POINT('',#271699);
#44633=VERTEX_POINT('',#271711);
#44634=VERTEX_POINT('',#271713);
#44635=VERTEX_POINT('',#272376);
#44636=VERTEX_POINT('',#272377);
#44637=VERTEX_POINT('',#272379);
#44638=VERTEX_POINT('',#272717);
#44639=VERTEX_POINT('',#272718);
#44640=VERTEX_POINT('',#272723);
#44641=VERTEX_POINT('',#273058);
#44642=VERTEX_POINT('',#273059);
#44643=VERTEX_POINT('',#273067);
#44644=VERTEX_POINT('',#273399);
#44645=VERTEX_POINT('',#273400);
#44646=VERTEX_POINT('',#273408);
#59008=EDGE_CURVE('',#44556,#44557,#5393,.T.);
#59009=EDGE_CURVE('',#44558,#44556,#4149,.T.);
#59010=EDGE_CURVE('',#44558,#44559,#24214,.T.);
#59011=EDGE_CURVE('',#44559,#44557,#4150,.T.);
#59012=EDGE_CURVE('',#44560,#44556,#24215,.T.);
#59013=EDGE_CURVE('',#44561,#44560,#4151,.T.);
#59014=EDGE_CURVE('',#44561,#44558,#24216,.T.);
#59015=EDGE_CURVE('',#44562,#44560,#5394,.T.);
#59016=EDGE_CURVE('',#44563,#44562,#4152,.T.);
#59017=EDGE_CURVE('',#44563,#44561,#24217,.T.);
#59018=EDGE_CURVE('',#44557,#44562,#24218,.T.);
#59019=EDGE_CURVE('',#44559,#44563,#24219,.T.);
#59020=EDGE_CURVE('',#44564,#44565,#5395,.T.);
#59021=EDGE_CURVE('',#44566,#44564,#4153,.T.);
#59022=EDGE_CURVE('',#44566,#44567,#24220,.T.);
#59023=EDGE_CURVE('',#44567,#44565,#4154,.T.);
#59024=EDGE_CURVE('',#44568,#44564,#24221,.T.);
#59025=EDGE_CURVE('',#44569,#44568,#4155,.T.);
#59026=EDGE_CURVE('',#44569,#44566,#24222,.T.);
#59027=EDGE_CURVE('',#44570,#44568,#5396,.T.);
#59028=EDGE_CURVE('',#44571,#44570,#4156,.T.);
#59029=EDGE_CURVE('',#44571,#44569,#24223,.T.);
#59030=EDGE_CURVE('',#44565,#44570,#24224,.T.);
#59031=EDGE_CURVE('',#44567,#44571,#24225,.T.);
#59032=EDGE_CURVE('',#44572,#44572,#36204,.T.);
#59033=EDGE_CURVE('',#44572,#44573,#24226,.T.);
#59034=EDGE_CURVE('',#44573,#44573,#36205,.T.);
#59035=EDGE_CURVE('',#44574,#44572,#24227,.T.);
#59036=EDGE_CURVE('',#44575,#44575,#5397,.T.);
#59037=EDGE_CURVE('',#44575,#44576,#24228,.T.);
#59038=EDGE_CURVE('',#44576,#44576,#36206,.T.);
#59039=EDGE_CURVE('',#44577,#44578,#5398,.T.);
#59040=EDGE_CURVE('',#44578,#44579,#5399,.T.);
#59041=EDGE_CURVE('',#44579,#44580,#5400,.T.);
#59042=EDGE_CURVE('',#44580,#44577,#5401,.T.);
#59043=EDGE_CURVE('',#44581,#44582,#5402,.T.);
#59044=EDGE_CURVE('',#44581,#44583,#24229,.T.);
#59045=EDGE_CURVE('',#44583,#44583,#36207,.T.);
#59046=EDGE_CURVE('',#44582,#44581,#5403,.T.);
#59047=EDGE_CURVE('',#44584,#44585,#5404,.T.);
#59048=EDGE_CURVE('',#44585,#44586,#5405,.T.);
#59049=EDGE_CURVE('',#44586,#44587,#5406,.T.);
#59050=EDGE_CURVE('',#44587,#44584,#5407,.T.);
#59051=EDGE_CURVE('',#44588,#44589,#5408,.T.);
#59052=EDGE_CURVE('',#44589,#44590,#24230,.T.);
#59053=EDGE_CURVE('',#44590,#44590,#36208,.T.);
#59054=EDGE_CURVE('',#44589,#44588,#5409,.T.);
#59055=EDGE_CURVE('',#44591,#44592,#5410,.T.);
#59056=EDGE_CURVE('',#44593,#44591,#5411,.T.);
#59057=EDGE_CURVE('',#44594,#44593,#5412,.T.);
#59058=EDGE_CURVE('',#44592,#44594,#5413,.T.);
#59059=EDGE_CURVE('',#44595,#44596,#5414,.T.);
#59060=EDGE_CURVE('',#44596,#44597,#24231,.T.);
#59061=EDGE_CURVE('',#44597,#44597,#36209,.T.);
#59062=EDGE_CURVE('',#44596,#44595,#5415,.T.);
#59063=EDGE_CURVE('',#44598,#44599,#5416,.T.);
#59064=EDGE_CURVE('',#44600,#44598,#5417,.T.);
#59065=EDGE_CURVE('',#44601,#44600,#5418,.T.);
#59066=EDGE_CURVE('',#44599,#44601,#5419,.T.);
#59067=EDGE_CURVE('',#44602,#44603,#5420,.T.);
#59068=EDGE_CURVE('',#44602,#44604,#24232,.T.);
#59069=EDGE_CURVE('',#44604,#44604,#36210,.T.);
#59070=EDGE_CURVE('',#44603,#44602,#5421,.T.);
#59071=EDGE_CURVE('',#44605,#44606,#5422,.T.);
#59072=EDGE_CURVE('',#44606,#44607,#5423,.T.);
#59073=EDGE_CURVE('',#44607,#44608,#5424,.T.);
#59074=EDGE_CURVE('',#44608,#44605,#5425,.T.);
#59075=EDGE_CURVE('',#44609,#44610,#5426,.T.);
#59076=EDGE_CURVE('',#44611,#44609,#5427,.T.);
#59077=EDGE_CURVE('',#44612,#44611,#5428,.T.);
#59078=EDGE_CURVE('',#44610,#44612,#5429,.T.);
#59079=EDGE_CURVE('',#44613,#44614,#5430,.T.);
#59080=EDGE_CURVE('',#44614,#44615,#24233,.T.);
#59081=EDGE_CURVE('',#44615,#44615,#36211,.T.);
#59082=EDGE_CURVE('',#44614,#44613,#5431,.T.);
#59083=EDGE_CURVE('',#44616,#44617,#5432,.T.);
#59084=EDGE_CURVE('',#44617,#44618,#5433,.T.);
#59085=EDGE_CURVE('',#44618,#44619,#5434,.T.);
#59086=EDGE_CURVE('',#44619,#44616,#5435,.T.);
#59087=EDGE_CURVE('',#44620,#44621,#5436,.T.);
#59088=EDGE_CURVE('',#44622,#44620,#5437,.T.);
#59089=EDGE_CURVE('',#44623,#44622,#5438,.T.);
#59090=EDGE_CURVE('',#44621,#44623,#5439,.T.);
#59091=EDGE_CURVE('',#44582,#44596,#36212,.T.);
#59092=EDGE_CURVE('',#44595,#44602,#24234,.T.);
#59093=EDGE_CURVE('',#44603,#44589,#24235,.T.);
#59094=EDGE_CURVE('',#44588,#44624,#24236,.T.);
#59095=EDGE_CURVE('',#44624,#44624,#36213,.T.);
#59096=EDGE_CURVE('',#44596,#44582,#36214,.T.);
#59097=EDGE_CURVE('',#44578,#44618,#4157,.T.);
#59098=EDGE_CURVE('',#44579,#44617,#4158,.T.);
#59099=EDGE_CURVE('',#44580,#44616,#4159,.T.);
#59100=EDGE_CURVE('',#44577,#44619,#4160,.T.);
#59101=EDGE_CURVE('',#44625,#44626,#5440,.T.);
#59102=EDGE_CURVE('',#44627,#44625,#24237,.T.);
#59103=EDGE_CURVE('',#44627,#44628,#5441,.T.);
#59104=EDGE_CURVE('',#44628,#44625,#5442,.T.);
#59105=EDGE_CURVE('',#44629,#44625,#24238,.T.);
#59106=EDGE_CURVE('',#44626,#44629,#5443,.T.);
#59107=EDGE_CURVE('',#44626,#44629,#36215,.T.);
#59108=EDGE_CURVE('',#44627,#44628,#36216,.T.);
#59109=EDGE_CURVE('',#44620,#44585,#4161,.T.);
#59110=EDGE_CURVE('',#44621,#44586,#4162,.T.);
#59111=EDGE_CURVE('',#44622,#44584,#4163,.T.);
#59112=EDGE_CURVE('',#44623,#44587,#4164,.T.);
#59113=EDGE_CURVE('',#44591,#44610,#4165,.T.);
#59114=EDGE_CURVE('',#44592,#44609,#4166,.T.);
#59115=EDGE_CURVE('',#44593,#44612,#4167,.T.);
#59116=EDGE_CURVE('',#44594,#44611,#4168,.T.);
#59117=EDGE_CURVE('',#44608,#44598,#4169,.T.);
#59118=EDGE_CURVE('',#44605,#44599,#4170,.T.);
#59119=EDGE_CURVE('',#44607,#44600,#4171,.T.);
#59120=EDGE_CURVE('',#44606,#44601,#4172,.T.);
#59121=EDGE_CURVE('',#44630,#44631,#24239,.T.);
#59122=EDGE_CURVE('',#44632,#44630,#5444,.T.);
#59123=EDGE_CURVE('',#44631,#44632,#5445,.T.);
#59124=EDGE_CURVE('',#44633,#44631,#24240,.T.);
#59125=EDGE_CURVE('',#44633,#44634,#5446,.T.);
#59126=EDGE_CURVE('',#44634,#44631,#5447,.T.);
#59127=EDGE_CURVE('',#44634,#44633,#36217,.T.);
#59128=EDGE_CURVE('',#44630,#44632,#36218,.T.);
#59129=EDGE_CURVE('',#44635,#44636,#24241,.T.);
#59130=EDGE_CURVE('',#44635,#44637,#5448,.T.);
#59131=EDGE_CURVE('',#44637,#44636,#5449,.T.);
#59132=EDGE_CURVE('',#44637,#44635,#36219,.T.);
#59133=EDGE_CURVE('',#44638,#44639,#5450,.T.);
#59134=EDGE_CURVE('',#44639,#44640,#5451,.T.);
#59135=EDGE_CURVE('',#44638,#44640,#24242,.T.);
#59136=EDGE_CURVE('',#44638,#44639,#36220,.T.);
#59137=EDGE_CURVE('',#44641,#44642,#5452,.T.);
#59138=EDGE_CURVE('',#44643,#44641,#24243,.T.);
#59139=EDGE_CURVE('',#44642,#44643,#5453,.T.);
#59140=EDGE_CURVE('',#44642,#44643,#36221,.T.);
#59141=EDGE_CURVE('',#44644,#44645,#5454,.T.);
#59142=EDGE_CURVE('',#44646,#44644,#24244,.T.);
#59143=EDGE_CURVE('',#44645,#44646,#5455,.T.);
#59144=EDGE_CURVE('',#44646,#44645,#36222,.T.);
#87459=ORIENTED_EDGE('',*,*,#59008,.F.);
#87460=ORIENTED_EDGE('',*,*,#59009,.F.);
#87461=ORIENTED_EDGE('',*,*,#59010,.T.);
#87462=ORIENTED_EDGE('',*,*,#59011,.T.);
#87463=ORIENTED_EDGE('',*,*,#59012,.F.);
#87464=ORIENTED_EDGE('',*,*,#59013,.F.);
#87465=ORIENTED_EDGE('',*,*,#59014,.T.);
#87466=ORIENTED_EDGE('',*,*,#59009,.T.);
#87467=ORIENTED_EDGE('',*,*,#59015,.F.);
#87468=ORIENTED_EDGE('',*,*,#59016,.F.);
#87469=ORIENTED_EDGE('',*,*,#59017,.T.);
#87470=ORIENTED_EDGE('',*,*,#59013,.T.);
#87471=ORIENTED_EDGE('',*,*,#59018,.F.);
#87472=ORIENTED_EDGE('',*,*,#59011,.F.);
#87473=ORIENTED_EDGE('',*,*,#59019,.T.);
#87474=ORIENTED_EDGE('',*,*,#59016,.T.);
#87475=ORIENTED_EDGE('',*,*,#59010,.F.);
#87476=ORIENTED_EDGE('',*,*,#59014,.F.);
#87477=ORIENTED_EDGE('',*,*,#59017,.F.);
#87478=ORIENTED_EDGE('',*,*,#59019,.F.);
#87479=ORIENTED_EDGE('',*,*,#59008,.T.);
#87480=ORIENTED_EDGE('',*,*,#59018,.T.);
#87481=ORIENTED_EDGE('',*,*,#59015,.T.);
#87482=ORIENTED_EDGE('',*,*,#59012,.T.);
#87483=ORIENTED_EDGE('',*,*,#59020,.F.);
#87484=ORIENTED_EDGE('',*,*,#59021,.F.);
#87485=ORIENTED_EDGE('',*,*,#59022,.T.);
#87486=ORIENTED_EDGE('',*,*,#59023,.T.);
#87487=ORIENTED_EDGE('',*,*,#59024,.F.);
#87488=ORIENTED_EDGE('',*,*,#59025,.F.);
#87489=ORIENTED_EDGE('',*,*,#59026,.T.);
#87490=ORIENTED_EDGE('',*,*,#59021,.T.);
#87491=ORIENTED_EDGE('',*,*,#59027,.F.);
#87492=ORIENTED_EDGE('',*,*,#59028,.F.);
#87493=ORIENTED_EDGE('',*,*,#59029,.T.);
#87494=ORIENTED_EDGE('',*,*,#59025,.T.);
#87495=ORIENTED_EDGE('',*,*,#59030,.F.);
#87496=ORIENTED_EDGE('',*,*,#59023,.F.);
#87497=ORIENTED_EDGE('',*,*,#59031,.T.);
#87498=ORIENTED_EDGE('',*,*,#59028,.T.);
#87499=ORIENTED_EDGE('',*,*,#59022,.F.);
#87500=ORIENTED_EDGE('',*,*,#59026,.F.);
#87501=ORIENTED_EDGE('',*,*,#59029,.F.);
#87502=ORIENTED_EDGE('',*,*,#59031,.F.);
#87503=ORIENTED_EDGE('',*,*,#59020,.T.);
#87504=ORIENTED_EDGE('',*,*,#59030,.T.);
#87505=ORIENTED_EDGE('',*,*,#59027,.T.);
#87506=ORIENTED_EDGE('',*,*,#59024,.T.);
#87507=ORIENTED_EDGE('',*,*,#59032,.F.);
#87508=ORIENTED_EDGE('',*,*,#59033,.T.);
#87509=ORIENTED_EDGE('',*,*,#59034,.T.);
#87510=ORIENTED_EDGE('',*,*,#59033,.F.);
#87511=ORIENTED_EDGE('',*,*,#59035,.T.);
#87512=ORIENTED_EDGE('',*,*,#59032,.T.);
#87513=ORIENTED_EDGE('',*,*,#59035,.F.);
#87514=ORIENTED_EDGE('',*,*,#59036,.F.);
#87515=ORIENTED_EDGE('',*,*,#59037,.T.);
#87516=ORIENTED_EDGE('',*,*,#59038,.T.);
#87517=ORIENTED_EDGE('',*,*,#59037,.F.);
#87518=ORIENTED_EDGE('',*,*,#59039,.T.);
#87519=ORIENTED_EDGE('',*,*,#59040,.T.);
#87520=ORIENTED_EDGE('',*,*,#59041,.T.);
#87521=ORIENTED_EDGE('',*,*,#59042,.T.);
#87522=ORIENTED_EDGE('',*,*,#59043,.F.);
#87523=ORIENTED_EDGE('',*,*,#59044,.T.);
#87524=ORIENTED_EDGE('',*,*,#59045,.T.);
#87525=ORIENTED_EDGE('',*,*,#59044,.F.);
#87526=ORIENTED_EDGE('',*,*,#59046,.F.);
#87527=ORIENTED_EDGE('',*,*,#59047,.T.);
#87528=ORIENTED_EDGE('',*,*,#59048,.T.);
#87529=ORIENTED_EDGE('',*,*,#59049,.T.);
#87530=ORIENTED_EDGE('',*,*,#59050,.T.);
#87531=ORIENTED_EDGE('',*,*,#59051,.T.);
#87532=ORIENTED_EDGE('',*,*,#59052,.T.);
#87533=ORIENTED_EDGE('',*,*,#59053,.F.);
#87534=ORIENTED_EDGE('',*,*,#59052,.F.);
#87535=ORIENTED_EDGE('',*,*,#59054,.T.);
#87536=ORIENTED_EDGE('',*,*,#59055,.F.);
#87537=ORIENTED_EDGE('',*,*,#59056,.F.);
#87538=ORIENTED_EDGE('',*,*,#59057,.F.);
#87539=ORIENTED_EDGE('',*,*,#59058,.F.);
#87540=ORIENTED_EDGE('',*,*,#59059,.T.);
#87541=ORIENTED_EDGE('',*,*,#59060,.T.);
#87542=ORIENTED_EDGE('',*,*,#59061,.F.);
#87543=ORIENTED_EDGE('',*,*,#59060,.F.);
#87544=ORIENTED_EDGE('',*,*,#59062,.T.);
#87545=ORIENTED_EDGE('',*,*,#59063,.F.);
#87546=ORIENTED_EDGE('',*,*,#59064,.F.);
#87547=ORIENTED_EDGE('',*,*,#59065,.F.);
#87548=ORIENTED_EDGE('',*,*,#59066,.F.);
#87549=ORIENTED_EDGE('',*,*,#59067,.F.);
#87550=ORIENTED_EDGE('',*,*,#59068,.T.);
#87551=ORIENTED_EDGE('',*,*,#59069,.F.);
#87552=ORIENTED_EDGE('',*,*,#59068,.F.);
#87553=ORIENTED_EDGE('',*,*,#59070,.F.);
#87554=ORIENTED_EDGE('',*,*,#59071,.T.);
#87555=ORIENTED_EDGE('',*,*,#59072,.T.);
#87556=ORIENTED_EDGE('',*,*,#59073,.T.);
#87557=ORIENTED_EDGE('',*,*,#59074,.T.);
#87558=ORIENTED_EDGE('',*,*,#59075,.F.);
#87559=ORIENTED_EDGE('',*,*,#59076,.F.);
#87560=ORIENTED_EDGE('',*,*,#59077,.F.);
#87561=ORIENTED_EDGE('',*,*,#59078,.F.);
#87562=ORIENTED_EDGE('',*,*,#59079,.T.);
#87563=ORIENTED_EDGE('',*,*,#59080,.T.);
#87564=ORIENTED_EDGE('',*,*,#59081,.T.);
#87565=ORIENTED_EDGE('',*,*,#59080,.F.);
#87566=ORIENTED_EDGE('',*,*,#59082,.T.);
#87567=ORIENTED_EDGE('',*,*,#59083,.T.);
#87568=ORIENTED_EDGE('',*,*,#59084,.T.);
#87569=ORIENTED_EDGE('',*,*,#59085,.T.);
#87570=ORIENTED_EDGE('',*,*,#59086,.T.);
#87571=ORIENTED_EDGE('',*,*,#59087,.F.);
#87572=ORIENTED_EDGE('',*,*,#59088,.F.);
#87573=ORIENTED_EDGE('',*,*,#59089,.F.);
#87574=ORIENTED_EDGE('',*,*,#59090,.F.);
#87575=ORIENTED_EDGE('',*,*,#59043,.T.);
#87576=ORIENTED_EDGE('',*,*,#59091,.T.);
#87577=ORIENTED_EDGE('',*,*,#59059,.F.);
#87578=ORIENTED_EDGE('',*,*,#59092,.T.);
#87579=ORIENTED_EDGE('',*,*,#59067,.T.);
#87580=ORIENTED_EDGE('',*,*,#59093,.T.);
#87581=ORIENTED_EDGE('',*,*,#59051,.F.);
#87582=ORIENTED_EDGE('',*,*,#59094,.T.);
#87583=ORIENTED_EDGE('',*,*,#59095,.T.);
#87584=ORIENTED_EDGE('',*,*,#59094,.F.);
#87585=ORIENTED_EDGE('',*,*,#59054,.F.);
#87586=ORIENTED_EDGE('',*,*,#59093,.F.);
#87587=ORIENTED_EDGE('',*,*,#59070,.T.);
#87588=ORIENTED_EDGE('',*,*,#59092,.F.);
#87589=ORIENTED_EDGE('',*,*,#59062,.F.);
#87590=ORIENTED_EDGE('',*,*,#59096,.T.);
#87591=ORIENTED_EDGE('',*,*,#59046,.T.);
#87592=ORIENTED_EDGE('',*,*,#59036,.T.);
#87593=ORIENTED_EDGE('',*,*,#59079,.F.);
#87594=ORIENTED_EDGE('',*,*,#59082,.F.);
#87595=ORIENTED_EDGE('',*,*,#59040,.F.);
#87596=ORIENTED_EDGE('',*,*,#59097,.T.);
#87597=ORIENTED_EDGE('',*,*,#59084,.F.);
#87598=ORIENTED_EDGE('',*,*,#59098,.F.);
#87599=ORIENTED_EDGE('',*,*,#59041,.F.);
#87600=ORIENTED_EDGE('',*,*,#59098,.T.);
#87601=ORIENTED_EDGE('',*,*,#59083,.F.);
#87602=ORIENTED_EDGE('',*,*,#59099,.F.);
#87603=ORIENTED_EDGE('',*,*,#59042,.F.);
#87604=ORIENTED_EDGE('',*,*,#59099,.T.);
#87605=ORIENTED_EDGE('',*,*,#59086,.F.);
#87606=ORIENTED_EDGE('',*,*,#59100,.F.);
#87607=ORIENTED_EDGE('',*,*,#59039,.F.);
#87608=ORIENTED_EDGE('',*,*,#59100,.T.);
#87609=ORIENTED_EDGE('',*,*,#59085,.F.);
#87610=ORIENTED_EDGE('',*,*,#59097,.F.);
#87611=ORIENTED_EDGE('',*,*,#59081,.F.);
#87612=ORIENTED_EDGE('',*,*,#59101,.F.);
#87613=ORIENTED_EDGE('',*,*,#59102,.F.);
#87614=ORIENTED_EDGE('',*,*,#59103,.T.);
#87615=ORIENTED_EDGE('',*,*,#59104,.T.);
#87616=ORIENTED_EDGE('',*,*,#59105,.F.);
#87617=ORIENTED_EDGE('',*,*,#59106,.F.);
#87618=ORIENTED_EDGE('',*,*,#59105,.T.);
#87619=ORIENTED_EDGE('',*,*,#59101,.T.);
#87620=ORIENTED_EDGE('',*,*,#59107,.T.);
#87621=ORIENTED_EDGE('',*,*,#59107,.F.);
#87622=ORIENTED_EDGE('',*,*,#59106,.T.);
#87623=ORIENTED_EDGE('',*,*,#59103,.F.);
#87624=ORIENTED_EDGE('',*,*,#59108,.T.);
#87625=ORIENTED_EDGE('',*,*,#59104,.F.);
#87626=ORIENTED_EDGE('',*,*,#59108,.F.);
#87627=ORIENTED_EDGE('',*,*,#59102,.T.);
#87628=ORIENTED_EDGE('',*,*,#59048,.F.);
#87629=ORIENTED_EDGE('',*,*,#59109,.F.);
#87630=ORIENTED_EDGE('',*,*,#59087,.T.);
#87631=ORIENTED_EDGE('',*,*,#59110,.T.);
#87632=ORIENTED_EDGE('',*,*,#59047,.F.);
#87633=ORIENTED_EDGE('',*,*,#59111,.F.);
#87634=ORIENTED_EDGE('',*,*,#59088,.T.);
#87635=ORIENTED_EDGE('',*,*,#59109,.T.);
#87636=ORIENTED_EDGE('',*,*,#59050,.F.);
#87637=ORIENTED_EDGE('',*,*,#59112,.F.);
#87638=ORIENTED_EDGE('',*,*,#59089,.T.);
#87639=ORIENTED_EDGE('',*,*,#59111,.T.);
#87640=ORIENTED_EDGE('',*,*,#59049,.F.);
#87641=ORIENTED_EDGE('',*,*,#59110,.F.);
#87642=ORIENTED_EDGE('',*,*,#59090,.T.);
#87643=ORIENTED_EDGE('',*,*,#59112,.T.);
#87644=ORIENTED_EDGE('',*,*,#59113,.F.);
#87645=ORIENTED_EDGE('',*,*,#59055,.T.);
#87646=ORIENTED_EDGE('',*,*,#59114,.T.);
#87647=ORIENTED_EDGE('',*,*,#59075,.T.);
#87648=ORIENTED_EDGE('',*,*,#59115,.F.);
#87649=ORIENTED_EDGE('',*,*,#59056,.T.);
#87650=ORIENTED_EDGE('',*,*,#59113,.T.);
#87651=ORIENTED_EDGE('',*,*,#59078,.T.);
#87652=ORIENTED_EDGE('',*,*,#59116,.F.);
#87653=ORIENTED_EDGE('',*,*,#59057,.T.);
#87654=ORIENTED_EDGE('',*,*,#59115,.T.);
#87655=ORIENTED_EDGE('',*,*,#59077,.T.);
#87656=ORIENTED_EDGE('',*,*,#59114,.F.);
#87657=ORIENTED_EDGE('',*,*,#59058,.T.);
#87658=ORIENTED_EDGE('',*,*,#59116,.T.);
#87659=ORIENTED_EDGE('',*,*,#59076,.T.);
#87660=ORIENTED_EDGE('',*,*,#59117,.T.);
#87661=ORIENTED_EDGE('',*,*,#59063,.T.);
#87662=ORIENTED_EDGE('',*,*,#59118,.F.);
#87663=ORIENTED_EDGE('',*,*,#59074,.F.);
#87664=ORIENTED_EDGE('',*,*,#59119,.T.);
#87665=ORIENTED_EDGE('',*,*,#59064,.T.);
#87666=ORIENTED_EDGE('',*,*,#59117,.F.);
#87667=ORIENTED_EDGE('',*,*,#59073,.F.);
#87668=ORIENTED_EDGE('',*,*,#59118,.T.);
#87669=ORIENTED_EDGE('',*,*,#59066,.T.);
#87670=ORIENTED_EDGE('',*,*,#59120,.F.);
#87671=ORIENTED_EDGE('',*,*,#59071,.F.);
#87672=ORIENTED_EDGE('',*,*,#59120,.T.);
#87673=ORIENTED_EDGE('',*,*,#59065,.T.);
#87674=ORIENTED_EDGE('',*,*,#59119,.F.);
#87675=ORIENTED_EDGE('',*,*,#59072,.F.);
#87676=ORIENTED_EDGE('',*,*,#59069,.T.);
#87677=ORIENTED_EDGE('',*,*,#59121,.F.);
#87678=ORIENTED_EDGE('',*,*,#59122,.F.);
#87679=ORIENTED_EDGE('',*,*,#59123,.F.);
#87680=ORIENTED_EDGE('',*,*,#59124,.F.);
#87681=ORIENTED_EDGE('',*,*,#59125,.T.);
#87682=ORIENTED_EDGE('',*,*,#59126,.T.);
#87683=ORIENTED_EDGE('',*,*,#59125,.F.);
#87684=ORIENTED_EDGE('',*,*,#59127,.F.);
#87685=ORIENTED_EDGE('',*,*,#59126,.F.);
#87686=ORIENTED_EDGE('',*,*,#59127,.T.);
#87687=ORIENTED_EDGE('',*,*,#59124,.T.);
#87688=ORIENTED_EDGE('',*,*,#59128,.T.);
#87689=ORIENTED_EDGE('',*,*,#59122,.T.);
#87690=ORIENTED_EDGE('',*,*,#59121,.T.);
#87691=ORIENTED_EDGE('',*,*,#59123,.T.);
#87692=ORIENTED_EDGE('',*,*,#59128,.F.);
#87693=ORIENTED_EDGE('',*,*,#59061,.T.);
#87694=ORIENTED_EDGE('',*,*,#59129,.F.);
#87695=ORIENTED_EDGE('',*,*,#59130,.T.);
#87696=ORIENTED_EDGE('',*,*,#59131,.T.);
#87697=ORIENTED_EDGE('',*,*,#59131,.F.);
#87698=ORIENTED_EDGE('',*,*,#59132,.T.);
#87699=ORIENTED_EDGE('',*,*,#59129,.T.);
#87700=ORIENTED_EDGE('',*,*,#59130,.F.);
#87701=ORIENTED_EDGE('',*,*,#59132,.F.);
#87702=ORIENTED_EDGE('',*,*,#59053,.T.);
#87703=ORIENTED_EDGE('',*,*,#59133,.T.);
#87704=ORIENTED_EDGE('',*,*,#59134,.T.);
#87705=ORIENTED_EDGE('',*,*,#59135,.F.);
#87706=ORIENTED_EDGE('',*,*,#59134,.F.);
#87707=ORIENTED_EDGE('',*,*,#59136,.F.);
#87708=ORIENTED_EDGE('',*,*,#59135,.T.);
#87709=ORIENTED_EDGE('',*,*,#59133,.F.);
#87710=ORIENTED_EDGE('',*,*,#59136,.T.);
#87711=ORIENTED_EDGE('',*,*,#59045,.F.);
#87712=ORIENTED_EDGE('',*,*,#59137,.F.);
#87713=ORIENTED_EDGE('',*,*,#59138,.F.);
#87714=ORIENTED_EDGE('',*,*,#59139,.F.);
#87715=ORIENTED_EDGE('',*,*,#59138,.T.);
#87716=ORIENTED_EDGE('',*,*,#59137,.T.);
#87717=ORIENTED_EDGE('',*,*,#59140,.T.);
#87718=ORIENTED_EDGE('',*,*,#59140,.F.);
#87719=ORIENTED_EDGE('',*,*,#59139,.T.);
#87720=ORIENTED_EDGE('',*,*,#59038,.F.);
#87721=ORIENTED_EDGE('',*,*,#59141,.F.);
#87722=ORIENTED_EDGE('',*,*,#59142,.F.);
#87723=ORIENTED_EDGE('',*,*,#59143,.F.);
#87724=ORIENTED_EDGE('',*,*,#59144,.T.);
#87725=ORIENTED_EDGE('',*,*,#59143,.T.);
#87726=ORIENTED_EDGE('',*,*,#59142,.T.);
#87727=ORIENTED_EDGE('',*,*,#59141,.T.);
#87728=ORIENTED_EDGE('',*,*,#59144,.F.);
#87729=ORIENTED_EDGE('',*,*,#59095,.F.);
#87730=ORIENTED_EDGE('',*,*,#59034,.F.);
#87731=ORIENTED_EDGE('',*,*,#59091,.F.);
#87732=ORIENTED_EDGE('',*,*,#59096,.F.);
#92419=CYLINDRICAL_SURFACE('',#110839,3.4);
#92420=CYLINDRICAL_SURFACE('',#110843,7.49999999999995);
#92421=CYLINDRICAL_SURFACE('',#110845,7.49999999999995);
#92422=CYLINDRICAL_SURFACE('',#110847,7.49999999999995);
#92423=CYLINDRICAL_SURFACE('',#110849,7.49999999999995);
#92424=CYLINDRICAL_SURFACE('',#110851,7.49999999999995);
#92425=CYLINDRICAL_SURFACE('',#110853,7.49999999999995);
#92426=CYLINDRICAL_SURFACE('',#110855,15.);
#98174=ADVANCED_FACE('',(#13201),#4017,.T.);
#98175=ADVANCED_FACE('',(#13202),#4018,.T.);
#98176=ADVANCED_FACE('',(#13203),#4019,.T.);
#98177=ADVANCED_FACE('',(#13204),#4020,.T.);
#98178=ADVANCED_FACE('',(#13205),#7316,.F.);
#98179=ADVANCED_FACE('',(#13206),#7317,.F.);
#98180=ADVANCED_FACE('',(#13207),#4021,.T.);
#98181=ADVANCED_FACE('',(#13208),#4022,.T.);
#98182=ADVANCED_FACE('',(#13209),#4023,.T.);
#98183=ADVANCED_FACE('',(#13210),#4024,.T.);
#98184=ADVANCED_FACE('',(#13211),#7318,.F.);
#98185=ADVANCED_FACE('',(#13212),#7319,.F.);
#98186=ADVANCED_FACE('',(#13213),#92419,.F.);
#98187=ADVANCED_FACE('',(#13214),#335,.F.);
#98188=ADVANCED_FACE('',(#13215,#6425),#92420,.T.);
#98189=ADVANCED_FACE('',(#13216,#6426),#92421,.T.);
#98190=ADVANCED_FACE('',(#13217,#6427),#92422,.T.);
#98191=ADVANCED_FACE('',(#13218,#6428),#92423,.T.);
#98192=ADVANCED_FACE('',(#13219,#6429,#6430),#92424,.T.);
#98193=ADVANCED_FACE('',(#13220,#6431,#6432),#92425,.T.);
#98194=ADVANCED_FACE('',(#13221,#6433,#6434),#92426,.T.);
#98195=ADVANCED_FACE('',(#13222),#4025,.T.);
#98196=ADVANCED_FACE('',(#13223),#4026,.T.);
#98197=ADVANCED_FACE('',(#13224),#4027,.T.);
#98198=ADVANCED_FACE('',(#13225),#4028,.T.);
#98199=ADVANCED_FACE('',(#13226,#6435),#7320,.F.);
#98200=ADVANCED_FACE('',(#13227),#4029,.T.);
#98201=ADVANCED_FACE('',(#13228),#4030,.T.);
#98202=ADVANCED_FACE('',(#13229),#4031,.T.);
#98203=ADVANCED_FACE('',(#13230),#4032,.T.);
#98204=ADVANCED_FACE('',(#13231),#4033,.T.);
#98205=ADVANCED_FACE('',(#13232),#4034,.T.);
#98206=ADVANCED_FACE('',(#13233),#4035,.T.);
#98207=ADVANCED_FACE('',(#13234),#4036,.T.);
#98208=ADVANCED_FACE('',(#13235),#4037,.T.);
#98209=ADVANCED_FACE('',(#13236),#4038,.T.);
#98210=ADVANCED_FACE('',(#13237),#4039,.T.);
#98211=ADVANCED_FACE('',(#13238),#4040,.T.);
#98212=ADVANCED_FACE('',(#13239),#4041,.T.);
#98213=ADVANCED_FACE('',(#13240),#4042,.T.);
#98214=ADVANCED_FACE('',(#13241),#4043,.T.);
#98215=ADVANCED_FACE('',(#13242),#4044,.T.);
#98216=ADVANCED_FACE('',(#13243,#6436),#7321,.T.);
#98217=ADVANCED_FACE('',(#13244),#4045,.T.);
#98218=ADVANCED_FACE('',(#13245),#4046,.T.);
#98219=ADVANCED_FACE('',(#13246),#4047,.T.);
#98220=ADVANCED_FACE('',(#13247),#4048,.T.);
#98221=ADVANCED_FACE('',(#13248,#6437),#7322,.T.);
#98222=ADVANCED_FACE('',(#13249),#4049,.T.);
#98223=ADVANCED_FACE('',(#13250),#4050,.T.);
#98224=ADVANCED_FACE('',(#13251,#6438),#7323,.T.);
#98225=ADVANCED_FACE('',(#13252),#4051,.T.);
#98226=ADVANCED_FACE('',(#13253),#4052,.T.);
#98227=ADVANCED_FACE('',(#13254,#6439),#7324,.F.);
#98228=ADVANCED_FACE('',(#13255),#4053,.T.);
#98229=ADVANCED_FACE('',(#13256),#4054,.T.);
#98230=ADVANCED_FACE('',(#13257,#6440),#7325,.F.);
#98231=ADVANCED_FACE('',(#13258),#4055,.T.);
#98232=ADVANCED_FACE('',(#13259),#4056,.T.);
#98233=ADVANCED_FACE('',(#13260,#6441),#7326,.F.);
#98234=ADVANCED_FACE('',(#13261),#7327,.F.);
#98721=CLOSED_SHELL('',(#98174,#98175,#98176,#98177,#98178,#98179));
#98722=CLOSED_SHELL('',(#98180,#98181,#98182,#98183,#98184,#98185));
#98723=CLOSED_SHELL('',(#98186,#98187,#98188,#98189,#98190,#98191,#98192,
#98193,#98194,#98195,#98196,#98197,#98198,#98199,#98200,#98201,#98202,#98203,
#98204,#98205,#98206,#98207,#98208,#98209,#98210,#98211,#98212,#98213,#98214,
#98215,#98216,#98217,#98218,#98219,#98220,#98221,#98222,#98223,#98224,#98225,
#98226,#98227,#98228,#98229,#98230,#98231,#98232,#98233,#98234));
#110834=AXIS2_PLACEMENT_3D('',#265159,#139993,#139994);
#110835=AXIS2_PLACEMENT_3D('',#265862,#140001,#140002);
#110836=AXIS2_PLACEMENT_3D('',#265863,#140003,#140004);
#110837=AXIS2_PLACEMENT_3D('',#266566,#140011,#140012);
#110838=AXIS2_PLACEMENT_3D('',#266567,#140013,#140014);
#110839=AXIS2_PLACEMENT_3D('',#266568,#140015,#140016);
#110840=AXIS2_PLACEMENT_3D('',#266570,#140017,#140018);
#110841=AXIS2_PLACEMENT_3D('',#266573,#140020,#140021);
#110842=AXIS2_PLACEMENT_3D('',#266574,#140022,#140023);
#110843=AXIS2_PLACEMENT_3D('',#266577,#140025,#140026);
#110844=AXIS2_PLACEMENT_3D('',#266615,#140028,#140029);
#110845=AXIS2_PLACEMENT_3D('',#266652,#140030,#140031);
#110846=AXIS2_PLACEMENT_3D('',#266676,#140033,#140034);
#110847=AXIS2_PLACEMENT_3D('',#266731,#140035,#140036);
#110848=AXIS2_PLACEMENT_3D('',#266754,#140038,#140039);
#110849=AXIS2_PLACEMENT_3D('',#266810,#140040,#140041);
#110850=AXIS2_PLACEMENT_3D('',#266833,#140043,#140044);
#110851=AXIS2_PLACEMENT_3D('',#266889,#140045,#140046);
#110852=AXIS2_PLACEMENT_3D('',#266912,#140048,#140049);
#110853=AXIS2_PLACEMENT_3D('',#267004,#140050,#140051);
#110854=AXIS2_PLACEMENT_3D('',#267028,#140053,#140054);
#110855=AXIS2_PLACEMENT_3D('',#267119,#140055,#140056);
#110856=AXIS2_PLACEMENT_3D('',#267120,#140057,#140058);
#110857=AXIS2_PLACEMENT_3D('',#267125,#140062,#140063);
#110858=AXIS2_PLACEMENT_3D('',#267126,#140064,#140065);
#110859=AXIS2_PLACEMENT_3D('',#268099,#140066,#140067);
#110860=AXIS2_PLACEMENT_3D('',#268291,#140070,#140071);
#110861=AXIS2_PLACEMENT_3D('',#268616,#140072,#140073);
#110862=AXIS2_PLACEMENT_3D('',#271695,#140074,#140075);
#110863=AXIS2_PLACEMENT_3D('',#271887,#140078,#140079);
#110864=AXIS2_PLACEMENT_3D('',#272212,#140080,#140081);
#110865=AXIS2_PLACEMENT_3D('',#272375,#140082,#140083);
#110866=AXIS2_PLACEMENT_3D('',#272553,#140085,#140086);
#110867=AXIS2_PLACEMENT_3D('',#272716,#140087,#140088);
#110868=AXIS2_PLACEMENT_3D('',#272894,#140090,#140091);
#110869=AXIS2_PLACEMENT_3D('',#273057,#140092,#140093);
#110870=AXIS2_PLACEMENT_3D('',#273235,#140095,#140096);
#110871=AXIS2_PLACEMENT_3D('',#273398,#140097,#140098);
#110872=AXIS2_PLACEMENT_3D('',#273576,#140100,#140101);
#110873=AXIS2_PLACEMENT_3D('',#273739,#140102,#140103);
#110874=AXIS2_PLACEMENT_3D('',#273740,#140104,#140105);
#139993=DIRECTION('axis',(0.,0.,1.));
#139994=DIRECTION('refdir',(1.,0.,0.));
#139995=DIRECTION('',(0.,-0.861627801655617,0.507540669714367));
#139996=DIRECTION('',(0.981067125781876,-0.193668001254952,0.));
#139997=DIRECTION('',(1.,3.18032637262414E-16,0.));
#139998=DIRECTION('',(0.,0.861627801655617,-0.507540669714367));
#139999=DIRECTION('',(-0.923312500482147,0.384049510419433,-4.73695157173399E-15));
#140000=DIRECTION('',(-1.,-3.18032637262414E-16,0.));
#140001=DIRECTION('center_axis',(1.61414497707192E-16,-0.507540669714368,
-0.861627801655617));
#140002=DIRECTION('ref_axis',(1.4032263518717E-32,0.861627801655617,-0.507540669714367));
#140003=DIRECTION('center_axis',(0.,0.,1.));
#140004=DIRECTION('ref_axis',(1.,0.,0.));
#140005=DIRECTION('',(0.,-0.861627801655622,-0.507540669714359));
#140006=DIRECTION('',(0.923312500482125,-0.384049510419485,0.));
#140007=DIRECTION('',(1.,2.13949228703806E-15,-3.70074341541719E-15));
#140008=DIRECTION('',(0.,0.861627801655622,0.507540669714359));
#140009=DIRECTION('',(-0.981067125781872,0.193668001254975,2.368475785867E-15));
#140010=DIRECTION('',(-1.,-2.13949228703806E-15,3.70074341541719E-15));
#140011=DIRECTION('center_axis',(-4.27454276172943E-15,0.507540669714359,
-0.861627801655622));
#140012=DIRECTION('ref_axis',(-3.1205381319799E-31,0.861627801655622,0.507540669714359));
#140013=DIRECTION('center_axis',(0.,0.,1.));
#140014=DIRECTION('ref_axis',(1.,0.,0.));
#140015=DIRECTION('center_axis',(0.,0.,1.));
#140016=DIRECTION('ref_axis',(1.,0.,0.));
#140017=DIRECTION('center_axis',(0.,0.,1.));
#140018=DIRECTION('ref_axis',(1.,0.,0.));
#140019=DIRECTION('',(0.,0.,1.));
#140020=DIRECTION('center_axis',(0.,0.,1.));
#140021=DIRECTION('ref_axis',(1.,0.,0.));
#140022=DIRECTION('center_axis',(0.,0.,1.));
#140023=DIRECTION('ref_axis',(1.,0.,0.));
#140024=DIRECTION('',(-0.857167300702112,-1.04972719113862E-16,0.515038074910054));
#140025=DIRECTION('center_axis',(1.,0.,0.));
#140026=DIRECTION('ref_axis',(0.,0.,-1.));
#140027=DIRECTION('',(-1.,0.,0.));
#140028=DIRECTION('center_axis',(1.,0.,0.));
#140029=DIRECTION('ref_axis',(0.,0.,-1.));
#140030=DIRECTION('center_axis',(1.,0.,0.));
#140031=DIRECTION('ref_axis',(0.,0.,-1.));
#140032=DIRECTION('',(-1.,0.,0.));
#140033=DIRECTION('center_axis',(1.,0.,0.));
#140034=DIRECTION('ref_axis',(0.,0.,-1.));
#140035=DIRECTION('center_axis',(-1.,0.,0.));
#140036=DIRECTION('ref_axis',(0.,0.,1.));
#140037=DIRECTION('',(1.,0.,0.));
#140038=DIRECTION('center_axis',(1.,0.,0.));
#140039=DIRECTION('ref_axis',(0.,0.,-1.));
#140040=DIRECTION('center_axis',(-1.,0.,0.));
#140041=DIRECTION('ref_axis',(0.,0.,1.));
#140042=DIRECTION('',(1.,0.,0.));
#140043=DIRECTION('center_axis',(1.,0.,0.));
#140044=DIRECTION('ref_axis',(0.,0.,-1.));
#140045=DIRECTION('center_axis',(-1.,0.,0.));
#140046=DIRECTION('ref_axis',(0.,0.,1.));
#140047=DIRECTION('',(1.,0.,0.));
#140048=DIRECTION('center_axis',(1.,0.,0.));
#140049=DIRECTION('ref_axis',(0.,0.,-1.));
#140050=DIRECTION('center_axis',(1.,0.,0.));
#140051=DIRECTION('ref_axis',(0.,0.,-1.));
#140052=DIRECTION('',(-1.,0.,0.));
#140053=DIRECTION('center_axis',(1.,0.,0.));
#140054=DIRECTION('ref_axis',(0.,0.,-1.));
#140055=DIRECTION('center_axis',(0.,0.,-1.));
#140056=DIRECTION('ref_axis',(-1.,0.,0.));
#140057=DIRECTION('center_axis',(0.,0.,1.));
#140058=DIRECTION('ref_axis',(1.,0.,0.));
#140059=DIRECTION('',(0.,0.,1.));
#140060=DIRECTION('',(0.,0.,1.));
#140061=DIRECTION('',(0.,0.,1.));
#140062=DIRECTION('center_axis',(0.,0.,-1.));
#140063=DIRECTION('ref_axis',(-1.,0.,0.));
#140064=DIRECTION('center_axis',(0.,0.,1.));
#140065=DIRECTION('ref_axis',(1.,0.,0.));
#140066=DIRECTION('center_axis',(1.,0.,0.));
#140067=DIRECTION('ref_axis',(0.,0.,-1.));
#140068=DIRECTION('',(0.,0.861627801655622,0.507540669714359));
#140069=DIRECTION('',(0.,-0.861627801655622,-0.507540669714359));
#140070=DIRECTION('center_axis',(0.0081151995614808,-0.157069337498387,
-0.987554234841761));
#140071=DIRECTION('ref_axis',(-0.999613692707062,0.0249787695829795,-0.0121871416941057));
#140072=DIRECTION('center_axis',(-0.00811519956086331,-0.157069337498389,
-0.987554234841765));
#140073=DIRECTION('ref_axis',(-0.999613692707067,0.0275272506419769,0.00383612104018571));
#140074=DIRECTION('center_axis',(1.,0.,0.));
#140075=DIRECTION('ref_axis',(0.,0.,-1.));
#140076=DIRECTION('',(0.,-0.861627801655617,0.507540669714367));
#140077=DIRECTION('',(0.,0.861627801655617,-0.507540669714367));
#140078=DIRECTION('center_axis',(-0.00811519956275127,0.157069337498393,
-0.987554234841749));
#140079=DIRECTION('ref_axis',(0.999613692707052,-0.0249787695827683,-0.0121871416953586));
#140080=DIRECTION('center_axis',(0.0081151995614462,0.15706933749836,-0.987554234841765));
#140081=DIRECTION('ref_axis',(0.99961369270706,-0.027527250642151,0.0038361210407496));
#140082=DIRECTION('center_axis',(1.,0.,0.));
#140083=DIRECTION('ref_axis',(0.,0.,-1.));
#140084=DIRECTION('',(0.,0.861627801655617,-0.507540669714367));
#140085=DIRECTION('center_axis',(-0.00811519956150803,0.157069337498411,
-0.987554234841757));
#140086=DIRECTION('ref_axis',(0.999613692707061,-0.0249787695829988,-0.012187141694134));
#140087=DIRECTION('center_axis',(1.,0.,0.));
#140088=DIRECTION('ref_axis',(0.,0.,-1.));
#140089=DIRECTION('',(0.,-0.861627801655617,0.507540669714367));
#140090=DIRECTION('center_axis',(0.00811519956086742,0.157069337498383,
-0.987554234841766));
#140091=DIRECTION('ref_axis',(0.999613692707066,-0.027527250642027,0.00383612104018404));
#140092=DIRECTION('center_axis',(1.,0.,0.));
#140093=DIRECTION('ref_axis',(0.,0.,-1.));
#140094=DIRECTION('',(0.,-0.861627801655622,-0.507540669714359));
#140095=DIRECTION('center_axis',(0.00811519956148901,-0.157069337498403,
-0.987554234841758));
#140096=DIRECTION('ref_axis',(-0.999613692707061,0.0249787695830125,-0.012187141694119));
#140097=DIRECTION('center_axis',(1.,0.,0.));
#140098=DIRECTION('ref_axis',(0.,0.,-1.));
#140099=DIRECTION('',(0.,0.861627801655622,0.507540669714359));
#140100=DIRECTION('center_axis',(-0.00811519956206617,-0.157069337498402,
-0.987554234841754));
#140101=DIRECTION('ref_axis',(-0.999613692707057,0.0275272506421834,0.00383612104137151));
#140102=DIRECTION('center_axis',(0.,0.,-1.));
#140103=DIRECTION('ref_axis',(-1.,0.,0.));
#140104=DIRECTION('center_axis',(0.,0.,1.));
#140105=DIRECTION('ref_axis',(1.,0.,0.));
#265159=CARTESIAN_POINT('',(0.,0.,0.));
#265160=CARTESIAN_POINT('Ctrl Pts',(160.,4.30813900827813,372.462296651428));
#265161=CARTESIAN_POINT('Ctrl Pts',(160.339057893189,-8.28413408366083,
370.462296651428));
#265162=CARTESIAN_POINT('Ctrl Pts',(158.704075916301,-20.7744157382975,
368.462296651428));
#265163=CARTESIAN_POINT('Ctrl Pts',(157.069093939413,-33.2646973929343,
366.462296651428));
#265164=CARTESIAN_POINT('Ctrl Pts',(153.500330774912,-45.3454354230633,
364.462296651428));
#265165=CARTESIAN_POINT('Ctrl Pts',(149.931567610412,-57.4261734531924,
362.462296651428));
#265166=CARTESIAN_POINT('Ctrl Pts',(144.516898051455,-68.7998999948413,
360.462296651428));
#265167=CARTESIAN_POINT('Ctrl Pts',(139.102228492497,-80.1736265364901,
358.462296651428));
#265168=CARTESIAN_POINT('Ctrl Pts',(131.974979673883,-90.5602826949691,
356.462296651428));
#265169=CARTESIAN_POINT('Ctrl Pts',(124.847730855269,-100.946938853448,
354.462296651428));
#265170=CARTESIAN_POINT('Ctrl Pts',(116.183399296895,-110.0907706828,352.462296651428));
#265171=CARTESIAN_POINT('Ctrl Pts',(107.519067738521,-119.234602512152,
350.462296651428));
#265172=CARTESIAN_POINT('Ctrl Pts',(97.5309980386224,-126.9104585261,348.462296651428));
#265173=CARTESIAN_POINT('Ctrl Pts',(87.5429283387234,-134.586314540048,
346.462296651428));
#265174=CARTESIAN_POINT('Ctrl Pts',(76.4770599218137,-140.605189688823,
344.462296651428));
#265175=CARTESIAN_POINT('Ctrl Pts',(65.4111915049041,-146.624064837599,
342.462296651428));
#265176=CARTESIAN_POINT('Ctrl Pts',(53.5400027769198,-150.837754439537,
340.462296651428));
#265177=CARTESIAN_POINT('Ctrl Pts',(41.6688140489356,-155.051444041475,
338.462296651428));
#265178=CARTESIAN_POINT('Ctrl Pts',(29.2846130745764,-157.356193074143,
336.462296651428));
#265179=CARTESIAN_POINT('Ctrl Pts',(16.9004121002171,-159.660942106811,
334.462296651428));
#265180=CARTESIAN_POINT('Ctrl Pts',(4.30813900827814,-160.,332.462296651428));
#265181=CARTESIAN_POINT('Ctrl Pts',(-8.28413408366082,-160.339057893189,
330.462296651428));
#265182=CARTESIAN_POINT('Ctrl Pts',(-20.7744157382975,-158.704075916301,
328.462296651428));
#265183=CARTESIAN_POINT('Ctrl Pts',(-33.2646973929342,-157.069093939413,
326.462296651428));
#265184=CARTESIAN_POINT('Ctrl Pts',(-45.3454354230633,-153.500330774912,
324.462296651428));
#265185=CARTESIAN_POINT('Ctrl Pts',(-57.4261734531924,-149.931567610412,
322.462296651428));
#265186=CARTESIAN_POINT('Ctrl Pts',(-68.7998999948413,-144.516898051455,
320.462296651428));
#265187=CARTESIAN_POINT('Ctrl Pts',(-80.1736265364901,-139.102228492497,
318.462296651428));
#265188=CARTESIAN_POINT('Ctrl Pts',(-90.5602826949691,-131.974979673883,
316.462296651428));
#265189=CARTESIAN_POINT('Ctrl Pts',(-100.946938853448,-124.847730855269,
314.462296651428));
#265190=CARTESIAN_POINT('Ctrl Pts',(-110.0907706828,-116.183399296895,312.462296651428));
#265191=CARTESIAN_POINT('Ctrl Pts',(-119.234602512152,-107.519067738521,
310.462296651428));
#265192=CARTESIAN_POINT('Ctrl Pts',(-126.9104585261,-97.5309980386224,308.462296651428));
#265193=CARTESIAN_POINT('Ctrl Pts',(-134.586314540048,-87.5429283387234,
306.462296651428));
#265194=CARTESIAN_POINT('Ctrl Pts',(-140.605189688823,-76.4770599218137,
304.462296651428));
#265195=CARTESIAN_POINT('Ctrl Pts',(-146.624064837599,-65.4111915049041,
302.462296651428));
#265196=CARTESIAN_POINT('Ctrl Pts',(-150.837754439537,-53.5400027769199,
300.462296651428));
#265197=CARTESIAN_POINT('Ctrl Pts',(-155.051444041475,-41.6688140489356,
298.462296651428));
#265198=CARTESIAN_POINT('Ctrl Pts',(-157.356193074143,-29.2846130745764,
296.462296651428));
#265199=CARTESIAN_POINT('Ctrl Pts',(-159.660942106811,-16.9004121002171,
294.462296651428));
#265200=CARTESIAN_POINT('Ctrl Pts',(-160.,-4.30813900827815,292.462296651428));
#265201=CARTESIAN_POINT('Ctrl Pts',(-160.339057893189,8.28413408366081,
290.462296651428));
#265202=CARTESIAN_POINT('Ctrl Pts',(-158.704075916301,20.7744157382975,
288.462296651428));
#265203=CARTESIAN_POINT('Ctrl Pts',(-157.069093939413,33.2646973929342,
286.462296651428));
#265204=CARTESIAN_POINT('Ctrl Pts',(-153.500330774912,45.3454354230633,
284.462296651428));
#265205=CARTESIAN_POINT('Ctrl Pts',(-149.931567610412,57.4261734531924,
282.462296651428));
#265206=CARTESIAN_POINT('Ctrl Pts',(-144.516898051455,68.7998999948413,
280.462296651428));
#265207=CARTESIAN_POINT('Ctrl Pts',(-139.102228492497,80.1736265364901,
278.462296651428));
#265208=CARTESIAN_POINT('Ctrl Pts',(-131.974979673883,90.5602826949691,
276.462296651428));
#265209=CARTESIAN_POINT('Ctrl Pts',(-124.847730855269,100.946938853448,
274.462296651428));
#265210=CARTESIAN_POINT('Ctrl Pts',(-116.183399296895,110.0907706828,272.462296651428));
#265211=CARTESIAN_POINT('Ctrl Pts',(-107.519067738521,119.234602512152,
270.462296651428));
#265212=CARTESIAN_POINT('Ctrl Pts',(-97.5309980386224,126.9104585261,268.462296651428));
#265213=CARTESIAN_POINT('Ctrl Pts',(-87.5429283387233,134.586314540048,
266.462296651428));
#265214=CARTESIAN_POINT('Ctrl Pts',(-76.4770599218137,140.605189688823,
264.462296651428));
#265215=CARTESIAN_POINT('Ctrl Pts',(-65.4111915049042,146.624064837599,
262.462296651428));
#265216=CARTESIAN_POINT('Ctrl Pts',(-53.5400027769199,150.837754439537,
260.462296651428));
#265217=CARTESIAN_POINT('Ctrl Pts',(-41.6688140489356,155.051444041475,
258.462296651428));
#265218=CARTESIAN_POINT('Ctrl Pts',(-29.2846130745764,157.356193074143,
256.462296651428));
#265219=CARTESIAN_POINT('Ctrl Pts',(-16.9004121002172,159.660942106811,
254.462296651428));
#265220=CARTESIAN_POINT('Ctrl Pts',(-4.30813900827816,160.,252.462296651428));
#265221=CARTESIAN_POINT('Ctrl Pts',(8.28413408366087,160.339057893189,250.462296651428));
#265222=CARTESIAN_POINT('Ctrl Pts',(20.7744157382975,158.704075916301,248.462296651428));
#265223=CARTESIAN_POINT('Ctrl Pts',(33.2646973929342,157.069093939413,246.462296651428));
#265224=CARTESIAN_POINT('Ctrl Pts',(45.3454354230633,153.500330774912,244.462296651428));
#265225=CARTESIAN_POINT('Ctrl Pts',(57.4261734531925,149.931567610412,242.462296651428));
#265226=CARTESIAN_POINT('Ctrl Pts',(68.7998999948413,144.516898051455,240.462296651428));
#265227=CARTESIAN_POINT('Ctrl Pts',(80.1736265364901,139.102228492498,238.462296651428));
#265228=CARTESIAN_POINT('Ctrl Pts',(90.560282694969,131.974979673883,236.462296651428));
#265229=CARTESIAN_POINT('Ctrl Pts',(100.946938853448,124.847730855269,234.462296651428));
#265230=CARTESIAN_POINT('Ctrl Pts',(110.0907706828,116.183399296895,232.462296651428));
#265231=CARTESIAN_POINT('Ctrl Pts',(119.234602512152,107.519067738521,230.462296651428));
#265232=CARTESIAN_POINT('Ctrl Pts',(126.9104585261,97.5309980386224,228.462296651428));
#265233=CARTESIAN_POINT('Ctrl Pts',(134.586314540048,87.5429283387233,226.462296651428));
#265234=CARTESIAN_POINT('Ctrl Pts',(140.605189688823,76.4770599218137,224.462296651428));
#265235=CARTESIAN_POINT('Ctrl Pts',(146.624064837599,65.4111915049042,222.462296651428));
#265236=CARTESIAN_POINT('Ctrl Pts',(150.837754439537,53.5400027769199,220.462296651428));
#265237=CARTESIAN_POINT('Ctrl Pts',(155.051444041475,41.6688140489356,218.462296651428));
#265238=CARTESIAN_POINT('Ctrl Pts',(157.356193074143,29.2846130745764,216.462296651428));
#265239=CARTESIAN_POINT('Ctrl Pts',(159.660942106811,16.9004121002172,214.462296651428));
#265240=CARTESIAN_POINT('Ctrl Pts',(160.,4.30813900827813,212.462296651428));
#265241=CARTESIAN_POINT('Ctrl Pts',(160.,-4.30813900827805,377.537703348572));
#265242=CARTESIAN_POINT('Ctrl Pts',(159.660942106811,-16.900412100217,375.537703348572));
#265243=CARTESIAN_POINT('Ctrl Pts',(157.356193074143,-29.2846130745763,
373.537703348572));
#265244=CARTESIAN_POINT('Ctrl Pts',(155.051444041475,-41.6688140489355,
371.537703348572));
#265245=CARTESIAN_POINT('Ctrl Pts',(150.837754439537,-53.5400027769198,
369.537703348572));
#265246=CARTESIAN_POINT('Ctrl Pts',(146.624064837599,-65.411191504904,367.537703348572));
#265247=CARTESIAN_POINT('Ctrl Pts',(140.605189688823,-76.4770599218136,
365.537703348572));
#265248=CARTESIAN_POINT('Ctrl Pts',(134.586314540048,-87.5429283387233,
363.537703348572));
#265249=CARTESIAN_POINT('Ctrl Pts',(126.9104585261,-97.5309980386223,361.537703348572));
#265250=CARTESIAN_POINT('Ctrl Pts',(119.234602512152,-107.519067738521,
359.537703348572));
#265251=CARTESIAN_POINT('Ctrl Pts',(110.0907706828,-116.183399296895,357.537703348572));
#265252=CARTESIAN_POINT('Ctrl Pts',(100.946938853448,-124.847730855269,
355.537703348572));
#265253=CARTESIAN_POINT('Ctrl Pts',(90.5602826949691,-131.974979673883,
353.537703348572));
#265254=CARTESIAN_POINT('Ctrl Pts',(80.1736265364902,-139.102228492497,
351.537703348572));
#265255=CARTESIAN_POINT('Ctrl Pts',(68.7998999948414,-144.516898051454,
349.537703348572));
#265256=CARTESIAN_POINT('Ctrl Pts',(57.4261734531925,-149.931567610412,
347.537703348572));
#265257=CARTESIAN_POINT('Ctrl Pts',(45.3454354230634,-153.500330774912,
345.537703348572));
#265258=CARTESIAN_POINT('Ctrl Pts',(33.2646973929343,-157.069093939413,
343.537703348572));
#265259=CARTESIAN_POINT('Ctrl Pts',(20.7744157382976,-158.704075916301,
341.537703348572));
#265260=CARTESIAN_POINT('Ctrl Pts',(8.28413408366091,-160.339057893189,
339.537703348572));
#265261=CARTESIAN_POINT('Ctrl Pts',(-4.30813900827804,-160.,337.537703348572));
#265262=CARTESIAN_POINT('Ctrl Pts',(-16.900412100217,-159.660942106811,
335.537703348572));
#265263=CARTESIAN_POINT('Ctrl Pts',(-29.2846130745763,-157.356193074143,
333.537703348572));
#265264=CARTESIAN_POINT('Ctrl Pts',(-41.6688140489355,-155.051444041475,
331.537703348572));
#265265=CARTESIAN_POINT('Ctrl Pts',(-53.5400027769198,-150.837754439537,
329.537703348572));
#265266=CARTESIAN_POINT('Ctrl Pts',(-65.411191504904,-146.624064837599,
327.537703348572));
#265267=CARTESIAN_POINT('Ctrl Pts',(-76.4770599218136,-140.605189688823,
325.537703348572));
#265268=CARTESIAN_POINT('Ctrl Pts',(-87.5429283387233,-134.586314540048,
323.537703348572));
#265269=CARTESIAN_POINT('Ctrl Pts',(-97.5309980386223,-126.9104585261,321.537703348572));
#265270=CARTESIAN_POINT('Ctrl Pts',(-107.519067738521,-119.234602512152,
319.537703348572));
#265271=CARTESIAN_POINT('Ctrl Pts',(-116.183399296895,-110.0907706828,317.537703348572));
#265272=CARTESIAN_POINT('Ctrl Pts',(-124.847730855269,-100.946938853448,
315.537703348572));
#265273=CARTESIAN_POINT('Ctrl Pts',(-131.974979673883,-90.5602826949692,
313.537703348572));
#265274=CARTESIAN_POINT('Ctrl Pts',(-139.102228492497,-80.1736265364902,
311.537703348572));
#265275=CARTESIAN_POINT('Ctrl Pts',(-144.516898051454,-68.7998999948414,
309.537703348572));
#265276=CARTESIAN_POINT('Ctrl Pts',(-149.931567610412,-57.4261734531925,
307.537703348572));
#265277=CARTESIAN_POINT('Ctrl Pts',(-153.500330774912,-45.3454354230634,
305.537703348572));
#265278=CARTESIAN_POINT('Ctrl Pts',(-157.069093939413,-33.2646973929344,
303.537703348572));
#265279=CARTESIAN_POINT('Ctrl Pts',(-158.704075916301,-20.7744157382976,
301.537703348572));
#265280=CARTESIAN_POINT('Ctrl Pts',(-160.339057893189,-8.28413408366092,
299.537703348572));
#265281=CARTESIAN_POINT('Ctrl Pts',(-160.,4.30813900827803,297.537703348572));
#265282=CARTESIAN_POINT('Ctrl Pts',(-159.660942106811,16.900412100217,295.537703348572));
#265283=CARTESIAN_POINT('Ctrl Pts',(-157.356193074143,29.2846130745763,
293.537703348572));
#265284=CARTESIAN_POINT('Ctrl Pts',(-155.051444041475,41.6688140489355,
291.537703348572));
#265285=CARTESIAN_POINT('Ctrl Pts',(-150.837754439537,53.5400027769198,
289.537703348572));
#265286=CARTESIAN_POINT('Ctrl Pts',(-146.624064837599,65.411191504904,287.537703348572));
#265287=CARTESIAN_POINT('Ctrl Pts',(-140.605189688823,76.4770599218136,
285.537703348572));
#265288=CARTESIAN_POINT('Ctrl Pts',(-134.586314540048,87.5429283387233,
283.537703348572));
#265289=CARTESIAN_POINT('Ctrl Pts',(-126.9104585261,97.5309980386223,281.537703348572));
#265290=CARTESIAN_POINT('Ctrl Pts',(-119.234602512152,107.519067738521,
279.537703348572));
#265291=CARTESIAN_POINT('Ctrl Pts',(-110.0907706828,116.183399296895,277.537703348572));
#265292=CARTESIAN_POINT('Ctrl Pts',(-100.946938853448,124.847730855269,
275.537703348572));
#265293=CARTESIAN_POINT('Ctrl Pts',(-90.5602826949692,131.974979673883,
273.537703348572));
#265294=CARTESIAN_POINT('Ctrl Pts',(-80.1736265364901,139.102228492497,
271.537703348572));
#265295=CARTESIAN_POINT('Ctrl Pts',(-68.7998999948414,144.516898051454,
269.537703348572));
#265296=CARTESIAN_POINT('Ctrl Pts',(-57.4261734531926,149.931567610412,
267.537703348572));
#265297=CARTESIAN_POINT('Ctrl Pts',(-45.3454354230634,153.500330774912,
265.537703348572));
#265298=CARTESIAN_POINT('Ctrl Pts',(-33.2646973929343,157.069093939413,
263.537703348572));
#265299=CARTESIAN_POINT('Ctrl Pts',(-20.7744157382976,158.704075916301,
261.537703348572));
#265300=CARTESIAN_POINT('Ctrl Pts',(-8.284134083661,160.339057893189,259.537703348572));
#265301=CARTESIAN_POINT('Ctrl Pts',(4.30813900827803,160.,257.537703348572));
#265302=CARTESIAN_POINT('Ctrl Pts',(16.9004121002171,159.660942106811,255.537703348572));
#265303=CARTESIAN_POINT('Ctrl Pts',(29.2846130745762,157.356193074143,253.537703348572));
#265304=CARTESIAN_POINT('Ctrl Pts',(41.6688140489354,155.051444041476,251.537703348572));
#265305=CARTESIAN_POINT('Ctrl Pts',(53.5400027769198,150.837754439537,249.537703348572));
#265306=CARTESIAN_POINT('Ctrl Pts',(65.4111915049041,146.624064837599,247.537703348572));
#265307=CARTESIAN_POINT('Ctrl Pts',(76.4770599218136,140.605189688823,245.537703348572));
#265308=CARTESIAN_POINT('Ctrl Pts',(87.5429283387232,134.586314540048,243.537703348572));
#265309=CARTESIAN_POINT('Ctrl Pts',(97.5309980386223,126.9104585261,241.537703348572));
#265310=CARTESIAN_POINT('Ctrl Pts',(107.519067738521,119.234602512152,239.537703348572));
#265311=CARTESIAN_POINT('Ctrl Pts',(116.183399296895,110.0907706828,237.537703348572));
#265312=CARTESIAN_POINT('Ctrl Pts',(124.847730855269,100.946938853448,235.537703348572));
#265313=CARTESIAN_POINT('Ctrl Pts',(131.974979673883,90.5602826949692,233.537703348572));
#265314=CARTESIAN_POINT('Ctrl Pts',(139.102228492497,80.1736265364902,231.537703348572));
#265315=CARTESIAN_POINT('Ctrl Pts',(144.516898051454,68.7998999948414,229.537703348572));
#265316=CARTESIAN_POINT('Ctrl Pts',(149.931567610412,57.4261734531926,227.537703348572));
#265317=CARTESIAN_POINT('Ctrl Pts',(153.500330774912,45.3454354230634,225.537703348572));
#265318=CARTESIAN_POINT('Ctrl Pts',(157.069093939413,33.2646973929343,223.537703348572));
#265319=CARTESIAN_POINT('Ctrl Pts',(158.704075916301,20.7744157382976,221.537703348572));
#265320=CARTESIAN_POINT('Ctrl Pts',(160.339057893189,8.28413408366101,219.537703348572));
#265321=CARTESIAN_POINT('Ctrl Pts',(160.,-4.30813900827805,217.537703348572));
#265322=CARTESIAN_POINT('',(157.805088795962,-26.7603066464731,367.5));
#265323=CARTESIAN_POINT('',(146.075461400194,-65.4256802672709,367.500000000001));
#265324=CARTESIAN_POINT('Ctrl Pts',(157.805088795962,-26.7603066464731,
367.5));
#265325=CARTESIAN_POINT('Ctrl Pts',(156.638532817878,-33.4083424416554,
367.5));
#265326=CARTESIAN_POINT('Ctrl Pts',(155.071407572055,-39.9802096740409,
367.5));
#265327=CARTESIAN_POINT('Ctrl Pts',(152.131501324444,-49.6731919343085,
367.5));
#265328=CARTESIAN_POINT('Ctrl Pts',(151.053085052425,-52.8765297093718,
367.499999999997));
#265329=CARTESIAN_POINT('Ctrl Pts',(148.705612539596,-59.2094688002808,
367.499999999997));
#265330=CARTESIAN_POINT('Ctrl Pts',(147.437304082636,-62.3378048444613,
367.5));
#265331=CARTESIAN_POINT('Ctrl Pts',(146.075461400194,-65.4256802672709,
367.5));
#265332=CARTESIAN_POINT('',(160.,4.30813900827813,372.462296651428));
#265333=CARTESIAN_POINT('Ctrl Pts',(160.,4.30813900827813,372.462296651428));
#265334=CARTESIAN_POINT('Ctrl Pts',(160.339057893189,-8.28413408366083,
370.462296651428));
#265335=CARTESIAN_POINT('Ctrl Pts',(158.704075916301,-20.7744157382975,
368.462296651428));
#265336=CARTESIAN_POINT('Ctrl Pts',(158.311185598564,-23.7758621134173,
367.981691576521));
#265337=CARTESIAN_POINT('Ctrl Pts',(157.805088795962,-26.7603066464731,
367.5));
#265338=CARTESIAN_POINT('',(160.,-4.30813900827805,377.537703348572));
#265339=CARTESIAN_POINT('',(160.,3.64291929955129E-14,375.));
#265340=CARTESIAN_POINT('Ctrl Pts',(160.,-4.30813900827805,377.537703348572));
#265341=CARTESIAN_POINT('Ctrl Pts',(159.660942106811,-16.900412100217,375.537703348572));
#265342=CARTESIAN_POINT('Ctrl Pts',(157.356193074143,-29.2846130745763,
373.537703348572));
#265343=CARTESIAN_POINT('Ctrl Pts',(155.051444041475,-41.6688140489355,
371.537703348572));
#265344=CARTESIAN_POINT('Ctrl Pts',(150.837754439537,-53.5400027769198,
369.537703348572));
#265345=CARTESIAN_POINT('Ctrl Pts',(148.694504587761,-59.5781607537096,
368.520423931127));
#265346=CARTESIAN_POINT('Ctrl Pts',(146.075461400194,-65.4256802672709,
367.5));
#265347=CARTESIAN_POINT('Ctrl Pts',(130.,4.30813900827812,372.462296651428));
#265348=CARTESIAN_POINT('Ctrl Pts',(130.339057893189,-5.92308287892228,
370.462296651428));
#265349=CARTESIAN_POINT('Ctrl Pts',(129.073425698447,-16.0813817870906,
368.462296651428));
#265350=CARTESIAN_POINT('Ctrl Pts',(127.807793503704,-26.2396806952589,
366.462296651428));
#265351=CARTESIAN_POINT('Ctrl Pts',(124.968635286058,-36.0749255918149,
364.462296651428));
#265352=CARTESIAN_POINT('Ctrl Pts',(122.129477068411,-45.9101704883709,
362.462296651428));
#265353=CARTESIAN_POINT('Ctrl Pts',(117.786702325803,-55.1801850026549,
360.462296651428));
#265354=CARTESIAN_POINT('Ctrl Pts',(113.443927583196,-64.4501995169389,
358.462296651428));
#265355=CARTESIAN_POINT('Ctrl Pts',(107.704469842635,-72.9267251261949,
356.462296651428));
#265356=CARTESIAN_POINT('Ctrl Pts',(101.965012102074,-81.4032507354509,
354.462296651428));
#265357=CARTESIAN_POINT('Ctrl Pts',(94.9701958612989,-88.8775672472035,
352.462296651428));
#265358=CARTESIAN_POINT('Ctrl Pts',(87.9753796205242,-96.351883758956,350.462296651428));
#265359=CARTESIAN_POINT('Ctrl Pts',(79.8974404698481,-102.639948694851,
348.462296651428));
#265360=CARTESIAN_POINT('Ctrl Pts',(71.8195013191721,-108.928013630747,
346.462296651428));
#265361=CARTESIAN_POINT('Ctrl Pts',(62.8573449296273,-113.874993963172,
344.462296651428));
#265362=CARTESIAN_POINT('Ctrl Pts',(53.8951885400825,-118.821974295598,
342.462296651428));
#265363=CARTESIAN_POINT('Ctrl Pts',(44.2694929456714,-122.306058950682,
340.462296651428));
#265364=CARTESIAN_POINT('Ctrl Pts',(34.6437973512603,-125.790143605767,
338.462296651428));
#265365=CARTESIAN_POINT('Ctrl Pts',(24.5915791233694,-127.725542856289,
336.462296651428));
#265366=CARTESIAN_POINT('Ctrl Pts',(14.5393608954785,-129.660942106811,
334.462296651428));
#265367=CARTESIAN_POINT('Ctrl Pts',(4.30813900827813,-130.,332.462296651428));
#265368=CARTESIAN_POINT('Ctrl Pts',(-5.92308287892227,-130.339057893189,
330.462296651428));
#265369=CARTESIAN_POINT('Ctrl Pts',(-16.0813817870906,-129.073425698447,
328.462296651428));
#265370=CARTESIAN_POINT('Ctrl Pts',(-26.2396806952589,-127.807793503705,
326.462296651428));
#265371=CARTESIAN_POINT('Ctrl Pts',(-36.0749255918149,-124.968635286058,
324.462296651428));
#265372=CARTESIAN_POINT('Ctrl Pts',(-45.9101704883709,-122.129477068411,
322.462296651428));
#265373=CARTESIAN_POINT('Ctrl Pts',(-55.1801850026549,-117.786702325803,
320.462296651428));
#265374=CARTESIAN_POINT('Ctrl Pts',(-64.4501995169389,-113.443927583196,
318.462296651428));
#265375=CARTESIAN_POINT('Ctrl Pts',(-72.9267251261949,-107.704469842635,
316.462296651428));
#265376=CARTESIAN_POINT('Ctrl Pts',(-81.4032507354509,-101.965012102074,
314.462296651428));
#265377=CARTESIAN_POINT('Ctrl Pts',(-88.8775672472034,-94.9701958612989,
312.462296651428));
#265378=CARTESIAN_POINT('Ctrl Pts',(-96.351883758956,-87.9753796205242,
310.462296651428));
#265379=CARTESIAN_POINT('Ctrl Pts',(-102.639948694851,-79.8974404698482,
308.462296651428));
#265380=CARTESIAN_POINT('Ctrl Pts',(-108.928013630747,-71.8195013191721,
306.462296651428));
#265381=CARTESIAN_POINT('Ctrl Pts',(-113.874993963172,-62.8573449296273,
304.462296651428));
#265382=CARTESIAN_POINT('Ctrl Pts',(-118.821974295598,-53.8951885400825,
302.462296651428));
#265383=CARTESIAN_POINT('Ctrl Pts',(-122.306058950682,-44.2694929456714,
300.462296651428));
#265384=CARTESIAN_POINT('Ctrl Pts',(-125.790143605767,-34.6437973512603,
298.462296651428));
#265385=CARTESIAN_POINT('Ctrl Pts',(-127.725542856289,-24.5915791233694,
296.462296651428));
#265386=CARTESIAN_POINT('Ctrl Pts',(-129.660942106811,-14.5393608954785,
294.462296651428));
#265387=CARTESIAN_POINT('Ctrl Pts',(-130.,-4.30813900827813,292.462296651428));
#265388=CARTESIAN_POINT('Ctrl Pts',(-130.339057893189,5.92308287892227,
290.462296651428));
#265389=CARTESIAN_POINT('Ctrl Pts',(-129.073425698447,16.0813817870906,
288.462296651428));
#265390=CARTESIAN_POINT('Ctrl Pts',(-127.807793503705,26.2396806952589,
286.462296651428));
#265391=CARTESIAN_POINT('Ctrl Pts',(-124.968635286058,36.0749255918149,
284.462296651428));
#265392=CARTESIAN_POINT('Ctrl Pts',(-122.129477068411,45.9101704883709,
282.462296651428));
#265393=CARTESIAN_POINT('Ctrl Pts',(-117.786702325803,55.1801850026549,
280.462296651428));
#265394=CARTESIAN_POINT('Ctrl Pts',(-113.443927583196,64.4501995169388,
278.462296651428));
#265395=CARTESIAN_POINT('Ctrl Pts',(-107.704469842635,72.9267251261949,
276.462296651428));
#265396=CARTESIAN_POINT('Ctrl Pts',(-101.965012102074,81.4032507354509,
274.462296651428));
#265397=CARTESIAN_POINT('Ctrl Pts',(-94.9701958612989,88.8775672472034,
272.462296651428));
#265398=CARTESIAN_POINT('Ctrl Pts',(-87.9753796205243,96.3518837589559,
270.462296651428));
#265399=CARTESIAN_POINT('Ctrl Pts',(-79.8974404698482,102.639948694851,
268.462296651428));
#265400=CARTESIAN_POINT('Ctrl Pts',(-71.819501319172,108.928013630747,266.462296651428));
#265401=CARTESIAN_POINT('Ctrl Pts',(-62.8573449296273,113.874993963172,
264.462296651428));
#265402=CARTESIAN_POINT('Ctrl Pts',(-53.8951885400826,118.821974295598,
262.462296651428));
#265403=CARTESIAN_POINT('Ctrl Pts',(-44.2694929456714,122.306058950682,
260.462296651428));
#265404=CARTESIAN_POINT('Ctrl Pts',(-34.6437973512603,125.790143605767,
258.462296651428));
#265405=CARTESIAN_POINT('Ctrl Pts',(-24.5915791233694,127.725542856289,
256.462296651428));
#265406=CARTESIAN_POINT('Ctrl Pts',(-14.5393608954786,129.660942106811,
254.462296651428));
#265407=CARTESIAN_POINT('Ctrl Pts',(-4.30813900827814,130.,252.462296651428));
#265408=CARTESIAN_POINT('Ctrl Pts',(5.92308287892232,130.339057893189,250.462296651428));
#265409=CARTESIAN_POINT('Ctrl Pts',(16.0813817870906,129.073425698447,248.462296651428));
#265410=CARTESIAN_POINT('Ctrl Pts',(26.2396806952589,127.807793503705,246.462296651428));
#265411=CARTESIAN_POINT('Ctrl Pts',(36.0749255918149,124.968635286058,244.462296651428));
#265412=CARTESIAN_POINT('Ctrl Pts',(45.9101704883709,122.129477068411,242.462296651428));
#265413=CARTESIAN_POINT('Ctrl Pts',(55.1801850026549,117.786702325803,240.462296651428));
#265414=CARTESIAN_POINT('Ctrl Pts',(64.4501995169388,113.443927583196,238.462296651428));
#265415=CARTESIAN_POINT('Ctrl Pts',(72.9267251261949,107.704469842635,236.462296651428));
#265416=CARTESIAN_POINT('Ctrl Pts',(81.4032507354509,101.965012102074,234.462296651428));
#265417=CARTESIAN_POINT('Ctrl Pts',(88.8775672472034,94.9701958612989,232.462296651428));
#265418=CARTESIAN_POINT('Ctrl Pts',(96.3518837589559,87.9753796205243,230.462296651428));
#265419=CARTESIAN_POINT('Ctrl Pts',(102.639948694851,79.8974404698482,228.462296651428));
#265420=CARTESIAN_POINT('Ctrl Pts',(108.928013630747,71.819501319172,226.462296651428));
#265421=CARTESIAN_POINT('Ctrl Pts',(113.874993963172,62.8573449296273,224.462296651428));
#265422=CARTESIAN_POINT('Ctrl Pts',(118.821974295598,53.8951885400826,222.462296651428));
#265423=CARTESIAN_POINT('Ctrl Pts',(122.306058950682,44.2694929456714,220.462296651428));
#265424=CARTESIAN_POINT('Ctrl Pts',(125.790143605767,34.6437973512603,218.462296651428));
#265425=CARTESIAN_POINT('Ctrl Pts',(127.725542856289,24.5915791233694,216.462296651428));
#265426=CARTESIAN_POINT('Ctrl Pts',(129.660942106811,14.5393608954786,214.462296651428));
#265427=CARTESIAN_POINT('Ctrl Pts',(130.,4.30813900827812,212.462296651428));
#265428=CARTESIAN_POINT('Ctrl Pts',(160.,4.30813900827813,372.462296651428));
#265429=CARTESIAN_POINT('Ctrl Pts',(160.339057893189,-8.28413408366083,
370.462296651428));
#265430=CARTESIAN_POINT('Ctrl Pts',(158.704075916301,-20.7744157382975,
368.462296651428));
#265431=CARTESIAN_POINT('Ctrl Pts',(157.069093939413,-33.2646973929343,
366.462296651428));
#265432=CARTESIAN_POINT('Ctrl Pts',(153.500330774912,-45.3454354230633,
364.462296651428));
#265433=CARTESIAN_POINT('Ctrl Pts',(149.931567610412,-57.4261734531924,
362.462296651428));
#265434=CARTESIAN_POINT('Ctrl Pts',(144.516898051455,-68.7998999948413,
360.462296651428));
#265435=CARTESIAN_POINT('Ctrl Pts',(139.102228492497,-80.1736265364901,
358.462296651428));
#265436=CARTESIAN_POINT('Ctrl Pts',(131.974979673883,-90.5602826949691,
356.462296651428));
#265437=CARTESIAN_POINT('Ctrl Pts',(124.847730855269,-100.946938853448,
354.462296651428));
#265438=CARTESIAN_POINT('Ctrl Pts',(116.183399296895,-110.0907706828,352.462296651428));
#265439=CARTESIAN_POINT('Ctrl Pts',(107.519067738521,-119.234602512152,
350.462296651428));
#265440=CARTESIAN_POINT('Ctrl Pts',(97.5309980386224,-126.9104585261,348.462296651428));
#265441=CARTESIAN_POINT('Ctrl Pts',(87.5429283387234,-134.586314540048,
346.462296651428));
#265442=CARTESIAN_POINT('Ctrl Pts',(76.4770599218137,-140.605189688823,
344.462296651428));
#265443=CARTESIAN_POINT('Ctrl Pts',(65.4111915049041,-146.624064837599,
342.462296651428));
#265444=CARTESIAN_POINT('Ctrl Pts',(53.5400027769198,-150.837754439537,
340.462296651428));
#265445=CARTESIAN_POINT('Ctrl Pts',(41.6688140489356,-155.051444041475,
338.462296651428));
#265446=CARTESIAN_POINT('Ctrl Pts',(29.2846130745764,-157.356193074143,
336.462296651428));
#265447=CARTESIAN_POINT('Ctrl Pts',(16.9004121002171,-159.660942106811,
334.462296651428));
#265448=CARTESIAN_POINT('Ctrl Pts',(4.30813900827814,-160.,332.462296651428));
#265449=CARTESIAN_POINT('Ctrl Pts',(-8.28413408366082,-160.339057893189,
330.462296651428));
#265450=CARTESIAN_POINT('Ctrl Pts',(-20.7744157382975,-158.704075916301,
328.462296651428));
#265451=CARTESIAN_POINT('Ctrl Pts',(-33.2646973929342,-157.069093939413,
326.462296651428));
#265452=CARTESIAN_POINT('Ctrl Pts',(-45.3454354230633,-153.500330774912,
324.462296651428));
#265453=CARTESIAN_POINT('Ctrl Pts',(-57.4261734531924,-149.931567610412,
322.462296651428));
#265454=CARTESIAN_POINT('Ctrl Pts',(-68.7998999948413,-144.516898051455,
320.462296651428));
#265455=CARTESIAN_POINT('Ctrl Pts',(-80.1736265364901,-139.102228492497,
318.462296651428));
#265456=CARTESIAN_POINT('Ctrl Pts',(-90.5602826949691,-131.974979673883,
316.462296651428));
#265457=CARTESIAN_POINT('Ctrl Pts',(-100.946938853448,-124.847730855269,
314.462296651428));
#265458=CARTESIAN_POINT('Ctrl Pts',(-110.0907706828,-116.183399296895,312.462296651428));
#265459=CARTESIAN_POINT('Ctrl Pts',(-119.234602512152,-107.519067738521,
310.462296651428));
#265460=CARTESIAN_POINT('Ctrl Pts',(-126.9104585261,-97.5309980386224,308.462296651428));
#265461=CARTESIAN_POINT('Ctrl Pts',(-134.586314540048,-87.5429283387234,
306.462296651428));
#265462=CARTESIAN_POINT('Ctrl Pts',(-140.605189688823,-76.4770599218137,
304.462296651428));
#265463=CARTESIAN_POINT('Ctrl Pts',(-146.624064837599,-65.4111915049041,
302.462296651428));
#265464=CARTESIAN_POINT('Ctrl Pts',(-150.837754439537,-53.5400027769199,
300.462296651428));
#265465=CARTESIAN_POINT('Ctrl Pts',(-155.051444041475,-41.6688140489356,
298.462296651428));
#265466=CARTESIAN_POINT('Ctrl Pts',(-157.356193074143,-29.2846130745764,
296.462296651428));
#265467=CARTESIAN_POINT('Ctrl Pts',(-159.660942106811,-16.9004121002171,
294.462296651428));
#265468=CARTESIAN_POINT('Ctrl Pts',(-160.,-4.30813900827815,292.462296651428));
#265469=CARTESIAN_POINT('Ctrl Pts',(-160.339057893189,8.28413408366081,
290.462296651428));
#265470=CARTESIAN_POINT('Ctrl Pts',(-158.704075916301,20.7744157382975,
288.462296651428));
#265471=CARTESIAN_POINT('Ctrl Pts',(-157.069093939413,33.2646973929342,
286.462296651428));
#265472=CARTESIAN_POINT('Ctrl Pts',(-153.500330774912,45.3454354230633,
284.462296651428));
#265473=CARTESIAN_POINT('Ctrl Pts',(-149.931567610412,57.4261734531924,
282.462296651428));
#265474=CARTESIAN_POINT('Ctrl Pts',(-144.516898051455,68.7998999948413,
280.462296651428));
#265475=CARTESIAN_POINT('Ctrl Pts',(-139.102228492497,80.1736265364901,
278.462296651428));
#265476=CARTESIAN_POINT('Ctrl Pts',(-131.974979673883,90.5602826949691,
276.462296651428));
#265477=CARTESIAN_POINT('Ctrl Pts',(-124.847730855269,100.946938853448,
274.462296651428));
#265478=CARTESIAN_POINT('Ctrl Pts',(-116.183399296895,110.0907706828,272.462296651428));
#265479=CARTESIAN_POINT('Ctrl Pts',(-107.519067738521,119.234602512152,
270.462296651428));
#265480=CARTESIAN_POINT('Ctrl Pts',(-97.5309980386224,126.9104585261,268.462296651428));
#265481=CARTESIAN_POINT('Ctrl Pts',(-87.5429283387233,134.586314540048,
266.462296651428));
#265482=CARTESIAN_POINT('Ctrl Pts',(-76.4770599218137,140.605189688823,
264.462296651428));
#265483=CARTESIAN_POINT('Ctrl Pts',(-65.4111915049042,146.624064837599,
262.462296651428));
#265484=CARTESIAN_POINT('Ctrl Pts',(-53.5400027769199,150.837754439537,
260.462296651428));
#265485=CARTESIAN_POINT('Ctrl Pts',(-41.6688140489356,155.051444041475,
258.462296651428));
#265486=CARTESIAN_POINT('Ctrl Pts',(-29.2846130745764,157.356193074143,
256.462296651428));
#265487=CARTESIAN_POINT('Ctrl Pts',(-16.9004121002172,159.660942106811,
254.462296651428));
#265488=CARTESIAN_POINT('Ctrl Pts',(-4.30813900827816,160.,252.462296651428));
#265489=CARTESIAN_POINT('Ctrl Pts',(8.28413408366087,160.339057893189,250.462296651428));
#265490=CARTESIAN_POINT('Ctrl Pts',(20.7744157382975,158.704075916301,248.462296651428));
#265491=CARTESIAN_POINT('Ctrl Pts',(33.2646973929342,157.069093939413,246.462296651428));
#265492=CARTESIAN_POINT('Ctrl Pts',(45.3454354230633,153.500330774912,244.462296651428));
#265493=CARTESIAN_POINT('Ctrl Pts',(57.4261734531925,149.931567610412,242.462296651428));
#265494=CARTESIAN_POINT('Ctrl Pts',(68.7998999948413,144.516898051455,240.462296651428));
#265495=CARTESIAN_POINT('Ctrl Pts',(80.1736265364901,139.102228492498,238.462296651428));
#265496=CARTESIAN_POINT('Ctrl Pts',(90.560282694969,131.974979673883,236.462296651428));
#265497=CARTESIAN_POINT('Ctrl Pts',(100.946938853448,124.847730855269,234.462296651428));
#265498=CARTESIAN_POINT('Ctrl Pts',(110.0907706828,116.183399296895,232.462296651428));
#265499=CARTESIAN_POINT('Ctrl Pts',(119.234602512152,107.519067738521,230.462296651428));
#265500=CARTESIAN_POINT('Ctrl Pts',(126.9104585261,97.5309980386224,228.462296651428));
#265501=CARTESIAN_POINT('Ctrl Pts',(134.586314540048,87.5429283387233,226.462296651428));
#265502=CARTESIAN_POINT('Ctrl Pts',(140.605189688823,76.4770599218137,224.462296651428));
#265503=CARTESIAN_POINT('Ctrl Pts',(146.624064837599,65.4111915049042,222.462296651428));
#265504=CARTESIAN_POINT('Ctrl Pts',(150.837754439537,53.5400027769199,220.462296651428));
#265505=CARTESIAN_POINT('Ctrl Pts',(155.051444041475,41.6688140489356,218.462296651428));
#265506=CARTESIAN_POINT('Ctrl Pts',(157.356193074143,29.2846130745764,216.462296651428));
#265507=CARTESIAN_POINT('Ctrl Pts',(159.660942106811,16.9004121002172,214.462296651428));
#265508=CARTESIAN_POINT('Ctrl Pts',(160.,4.30813900827813,212.462296651428));
#265509=CARTESIAN_POINT('',(128.373075022505,-20.9502666088245,367.5));
#265510=CARTESIAN_POINT('',(128.373075022505,-20.9502666088245,367.5));
#265511=CARTESIAN_POINT('',(130.,4.30813900827812,372.462296651428));
#265512=CARTESIAN_POINT('Ctrl Pts',(130.,4.30813900827812,372.462296651428));
#265513=CARTESIAN_POINT('Ctrl Pts',(130.339057893189,-5.92308287892229,
370.462296651428));
#265514=CARTESIAN_POINT('Ctrl Pts',(129.073425698447,-16.0813817870906,
368.462296651428));
#265515=CARTESIAN_POINT('Ctrl Pts',(128.769291070567,-18.522446790936,367.981691576521));
#265516=CARTESIAN_POINT('Ctrl Pts',(128.373075022505,-20.9502666088245,
367.5));
#265517=CARTESIAN_POINT('',(145.,4.30813900827812,372.462296651428));
#265518=CARTESIAN_POINT('Ctrl Pts',(130.,-4.30813900827807,377.537703348572));
#265519=CARTESIAN_POINT('Ctrl Pts',(129.660942106811,-14.5393608954785,
375.537703348572));
#265520=CARTESIAN_POINT('Ctrl Pts',(127.725542856289,-24.5915791233694,
373.537703348572));
#265521=CARTESIAN_POINT('Ctrl Pts',(125.790143605767,-34.6437973512603,
371.537703348572));
#265522=CARTESIAN_POINT('Ctrl Pts',(122.306058950682,-44.2694929456714,
369.537703348572));
#265523=CARTESIAN_POINT('Ctrl Pts',(118.821974295598,-53.8951885400825,
367.537703348572));
#265524=CARTESIAN_POINT('Ctrl Pts',(113.874993963172,-62.8573449296272,
365.537703348572));
#265525=CARTESIAN_POINT('Ctrl Pts',(108.928013630747,-71.819501319172,363.537703348572));
#265526=CARTESIAN_POINT('Ctrl Pts',(102.639948694851,-79.8974404698481,
361.537703348572));
#265527=CARTESIAN_POINT('Ctrl Pts',(96.351883758956,-87.9753796205242,359.537703348572));
#265528=CARTESIAN_POINT('Ctrl Pts',(88.8775672472035,-94.9701958612989,
357.537703348572));
#265529=CARTESIAN_POINT('Ctrl Pts',(81.403250735451,-101.965012102074,355.537703348572));
#265530=CARTESIAN_POINT('Ctrl Pts',(72.9267251261949,-107.704469842635,
353.537703348572));
#265531=CARTESIAN_POINT('Ctrl Pts',(64.4501995169389,-113.443927583196,
351.537703348572));
#265532=CARTESIAN_POINT('Ctrl Pts',(55.1801850026549,-117.786702325803,
349.537703348572));
#265533=CARTESIAN_POINT('Ctrl Pts',(45.910170488371,-122.129477068411,347.537703348572));
#265534=CARTESIAN_POINT('Ctrl Pts',(36.074925591815,-124.968635286058,345.537703348572));
#265535=CARTESIAN_POINT('Ctrl Pts',(26.239680695259,-127.807793503704,343.537703348572));
#265536=CARTESIAN_POINT('Ctrl Pts',(16.0813817870907,-129.073425698447,
341.537703348572));
#265537=CARTESIAN_POINT('Ctrl Pts',(5.92308287892234,-130.339057893189,
339.537703348572));
#265538=CARTESIAN_POINT('Ctrl Pts',(-4.30813900827806,-130.,337.537703348572));
#265539=CARTESIAN_POINT('Ctrl Pts',(-14.5393608954785,-129.660942106811,
335.537703348572));
#265540=CARTESIAN_POINT('Ctrl Pts',(-24.5915791233694,-127.725542856289,
333.537703348572));
#265541=CARTESIAN_POINT('Ctrl Pts',(-34.6437973512603,-125.790143605767,
331.537703348572));
#265542=CARTESIAN_POINT('Ctrl Pts',(-44.2694929456713,-122.306058950682,
329.537703348572));
#265543=CARTESIAN_POINT('Ctrl Pts',(-53.8951885400825,-118.821974295598,
327.537703348572));
#265544=CARTESIAN_POINT('Ctrl Pts',(-62.8573449296272,-113.874993963172,
325.537703348572));
#265545=CARTESIAN_POINT('Ctrl Pts',(-71.819501319172,-108.928013630747,
323.537703348572));
#265546=CARTESIAN_POINT('Ctrl Pts',(-79.8974404698481,-102.639948694851,
321.537703348572));
#265547=CARTESIAN_POINT('Ctrl Pts',(-87.9753796205242,-96.351883758956,
319.537703348572));
#265548=CARTESIAN_POINT('Ctrl Pts',(-94.9701958612989,-88.8775672472035,
317.537703348572));
#265549=CARTESIAN_POINT('Ctrl Pts',(-101.965012102074,-81.403250735451,
315.537703348572));
#265550=CARTESIAN_POINT('Ctrl Pts',(-107.704469842635,-72.9267251261949,
313.537703348572));
#265551=CARTESIAN_POINT('Ctrl Pts',(-113.443927583196,-64.4501995169389,
311.537703348572));
#265552=CARTESIAN_POINT('Ctrl Pts',(-117.786702325803,-55.1801850026549,
309.537703348572));
#265553=CARTESIAN_POINT('Ctrl Pts',(-122.129477068411,-45.910170488371,
307.537703348572));
#265554=CARTESIAN_POINT('Ctrl Pts',(-124.968635286058,-36.074925591815,
305.537703348572));
#265555=CARTESIAN_POINT('Ctrl Pts',(-127.807793503704,-26.239680695259,
303.537703348572));
#265556=CARTESIAN_POINT('Ctrl Pts',(-129.073425698447,-16.0813817870907,
301.537703348572));
#265557=CARTESIAN_POINT('Ctrl Pts',(-130.339057893189,-5.92308287892235,
299.537703348572));
#265558=CARTESIAN_POINT('Ctrl Pts',(-130.,4.30813900827805,297.537703348572));
#265559=CARTESIAN_POINT('Ctrl Pts',(-129.660942106811,14.5393608954784,
295.537703348572));
#265560=CARTESIAN_POINT('Ctrl Pts',(-127.725542856289,24.5915791233693,
293.537703348572));
#265561=CARTESIAN_POINT('Ctrl Pts',(-125.790143605767,34.6437973512602,
291.537703348572));
#265562=CARTESIAN_POINT('Ctrl Pts',(-122.306058950682,44.2694929456713,
289.537703348572));
#265563=CARTESIAN_POINT('Ctrl Pts',(-118.821974295598,53.8951885400825,
287.537703348572));
#265564=CARTESIAN_POINT('Ctrl Pts',(-113.874993963172,62.8573449296272,
285.537703348572));
#265565=CARTESIAN_POINT('Ctrl Pts',(-108.928013630747,71.819501319172,283.537703348572));
#265566=CARTESIAN_POINT('Ctrl Pts',(-102.639948694851,79.8974404698481,
281.537703348572));
#265567=CARTESIAN_POINT('Ctrl Pts',(-96.3518837589561,87.9753796205242,
279.537703348572));
#265568=CARTESIAN_POINT('Ctrl Pts',(-88.8775672472035,94.9701958612989,
277.537703348572));
#265569=CARTESIAN_POINT('Ctrl Pts',(-81.403250735451,101.965012102074,275.537703348572));
#265570=CARTESIAN_POINT('Ctrl Pts',(-72.9267251261949,107.704469842635,
273.537703348572));
#265571=CARTESIAN_POINT('Ctrl Pts',(-64.4501995169389,113.443927583196,
271.537703348572));
#265572=CARTESIAN_POINT('Ctrl Pts',(-55.1801850026549,117.786702325803,
269.537703348572));
#265573=CARTESIAN_POINT('Ctrl Pts',(-45.910170488371,122.129477068411,267.537703348572));
#265574=CARTESIAN_POINT('Ctrl Pts',(-36.074925591815,124.968635286058,265.537703348572));
#265575=CARTESIAN_POINT('Ctrl Pts',(-26.239680695259,127.807793503704,263.537703348572));
#265576=CARTESIAN_POINT('Ctrl Pts',(-16.0813817870907,129.073425698447,
261.537703348572));
#265577=CARTESIAN_POINT('Ctrl Pts',(-5.92308287892242,130.339057893189,
259.537703348572));
#265578=CARTESIAN_POINT('Ctrl Pts',(4.30813900827804,130.,257.537703348572));
#265579=CARTESIAN_POINT('Ctrl Pts',(14.5393608954785,129.660942106811,255.537703348572));
#265580=CARTESIAN_POINT('Ctrl Pts',(24.5915791233693,127.725542856289,253.537703348572));
#265581=CARTESIAN_POINT('Ctrl Pts',(34.6437973512602,125.790143605767,251.537703348572));
#265582=CARTESIAN_POINT('Ctrl Pts',(44.2694929456713,122.306058950682,249.537703348572));
#265583=CARTESIAN_POINT('Ctrl Pts',(53.8951885400825,118.821974295598,247.537703348572));
#265584=CARTESIAN_POINT('Ctrl Pts',(62.8573449296272,113.874993963172,245.537703348572));
#265585=CARTESIAN_POINT('Ctrl Pts',(71.819501319172,108.928013630747,243.537703348572));
#265586=CARTESIAN_POINT('Ctrl Pts',(79.8974404698481,102.639948694851,241.537703348572));
#265587=CARTESIAN_POINT('Ctrl Pts',(87.9753796205242,96.351883758956,239.537703348572));
#265588=CARTESIAN_POINT('Ctrl Pts',(94.9701958612989,88.8775672472035,237.537703348572));
#265589=CARTESIAN_POINT('Ctrl Pts',(101.965012102074,81.403250735451,235.537703348572));
#265590=CARTESIAN_POINT('Ctrl Pts',(107.704469842635,72.926725126195,233.537703348572));
#265591=CARTESIAN_POINT('Ctrl Pts',(113.443927583196,64.4501995169389,231.537703348572));
#265592=CARTESIAN_POINT('Ctrl Pts',(117.786702325803,55.1801850026549,229.537703348572));
#265593=CARTESIAN_POINT('Ctrl Pts',(122.129477068411,45.910170488371,227.537703348572));
#265594=CARTESIAN_POINT('Ctrl Pts',(124.968635286058,36.074925591815,225.537703348572));
#265595=CARTESIAN_POINT('Ctrl Pts',(127.807793503704,26.239680695259,223.537703348572));
#265596=CARTESIAN_POINT('Ctrl Pts',(129.073425698447,16.0813817870907,221.537703348572));
#265597=CARTESIAN_POINT('Ctrl Pts',(130.339057893189,5.92308287892242,219.537703348572));
#265598=CARTESIAN_POINT('Ctrl Pts',(130.,-4.30813900827807,217.537703348572));
#265599=CARTESIAN_POINT('Ctrl Pts',(130.,4.30813900827812,372.462296651428));
#265600=CARTESIAN_POINT('Ctrl Pts',(130.339057893189,-5.92308287892228,
370.462296651428));
#265601=CARTESIAN_POINT('Ctrl Pts',(129.073425698447,-16.0813817870906,
368.462296651428));
#265602=CARTESIAN_POINT('Ctrl Pts',(127.807793503704,-26.2396806952589,
366.462296651428));
#265603=CARTESIAN_POINT('Ctrl Pts',(124.968635286058,-36.0749255918149,
364.462296651428));
#265604=CARTESIAN_POINT('Ctrl Pts',(122.129477068411,-45.9101704883709,
362.462296651428));
#265605=CARTESIAN_POINT('Ctrl Pts',(117.786702325803,-55.1801850026549,
360.462296651428));
#265606=CARTESIAN_POINT('Ctrl Pts',(113.443927583196,-64.4501995169389,
358.462296651428));
#265607=CARTESIAN_POINT('Ctrl Pts',(107.704469842635,-72.9267251261949,
356.462296651428));
#265608=CARTESIAN_POINT('Ctrl Pts',(101.965012102074,-81.4032507354509,
354.462296651428));
#265609=CARTESIAN_POINT('Ctrl Pts',(94.9701958612989,-88.8775672472035,
352.462296651428));
#265610=CARTESIAN_POINT('Ctrl Pts',(87.9753796205242,-96.351883758956,350.462296651428));
#265611=CARTESIAN_POINT('Ctrl Pts',(79.8974404698481,-102.639948694851,
348.462296651428));
#265612=CARTESIAN_POINT('Ctrl Pts',(71.8195013191721,-108.928013630747,
346.462296651428));
#265613=CARTESIAN_POINT('Ctrl Pts',(62.8573449296273,-113.874993963172,
344.462296651428));
#265614=CARTESIAN_POINT('Ctrl Pts',(53.8951885400825,-118.821974295598,
342.462296651428));
#265615=CARTESIAN_POINT('Ctrl Pts',(44.2694929456714,-122.306058950682,
340.462296651428));
#265616=CARTESIAN_POINT('Ctrl Pts',(34.6437973512603,-125.790143605767,
338.462296651428));
#265617=CARTESIAN_POINT('Ctrl Pts',(24.5915791233694,-127.725542856289,
336.462296651428));
#265618=CARTESIAN_POINT('Ctrl Pts',(14.5393608954785,-129.660942106811,
334.462296651428));
#265619=CARTESIAN_POINT('Ctrl Pts',(4.30813900827813,-130.,332.462296651428));
#265620=CARTESIAN_POINT('Ctrl Pts',(-5.92308287892227,-130.339057893189,
330.462296651428));
#265621=CARTESIAN_POINT('Ctrl Pts',(-16.0813817870906,-129.073425698447,
328.462296651428));
#265622=CARTESIAN_POINT('Ctrl Pts',(-26.2396806952589,-127.807793503705,
326.462296651428));
#265623=CARTESIAN_POINT('Ctrl Pts',(-36.0749255918149,-124.968635286058,
324.462296651428));
#265624=CARTESIAN_POINT('Ctrl Pts',(-45.9101704883709,-122.129477068411,
322.462296651428));
#265625=CARTESIAN_POINT('Ctrl Pts',(-55.1801850026549,-117.786702325803,
320.462296651428));
#265626=CARTESIAN_POINT('Ctrl Pts',(-64.4501995169389,-113.443927583196,
318.462296651428));
#265627=CARTESIAN_POINT('Ctrl Pts',(-72.9267251261949,-107.704469842635,
316.462296651428));
#265628=CARTESIAN_POINT('Ctrl Pts',(-81.4032507354509,-101.965012102074,
314.462296651428));
#265629=CARTESIAN_POINT('Ctrl Pts',(-88.8775672472034,-94.9701958612989,
312.462296651428));
#265630=CARTESIAN_POINT('Ctrl Pts',(-96.351883758956,-87.9753796205242,
310.462296651428));
#265631=CARTESIAN_POINT('Ctrl Pts',(-102.639948694851,-79.8974404698482,
308.462296651428));
#265632=CARTESIAN_POINT('Ctrl Pts',(-108.928013630747,-71.8195013191721,
306.462296651428));
#265633=CARTESIAN_POINT('Ctrl Pts',(-113.874993963172,-62.8573449296273,
304.462296651428));
#265634=CARTESIAN_POINT('Ctrl Pts',(-118.821974295598,-53.8951885400825,
302.462296651428));
#265635=CARTESIAN_POINT('Ctrl Pts',(-122.306058950682,-44.2694929456714,
300.462296651428));
#265636=CARTESIAN_POINT('Ctrl Pts',(-125.790143605767,-34.6437973512603,
298.462296651428));
#265637=CARTESIAN_POINT('Ctrl Pts',(-127.725542856289,-24.5915791233694,
296.462296651428));
#265638=CARTESIAN_POINT('Ctrl Pts',(-129.660942106811,-14.5393608954785,
294.462296651428));
#265639=CARTESIAN_POINT('Ctrl Pts',(-130.,-4.30813900827813,292.462296651428));
#265640=CARTESIAN_POINT('Ctrl Pts',(-130.339057893189,5.92308287892227,
290.462296651428));
#265641=CARTESIAN_POINT('Ctrl Pts',(-129.073425698447,16.0813817870906,
288.462296651428));
#265642=CARTESIAN_POINT('Ctrl Pts',(-127.807793503705,26.2396806952589,
286.462296651428));
#265643=CARTESIAN_POINT('Ctrl Pts',(-124.968635286058,36.0749255918149,
284.462296651428));
#265644=CARTESIAN_POINT('Ctrl Pts',(-122.129477068411,45.9101704883709,
282.462296651428));
#265645=CARTESIAN_POINT('Ctrl Pts',(-117.786702325803,55.1801850026549,
280.462296651428));
#265646=CARTESIAN_POINT('Ctrl Pts',(-113.443927583196,64.4501995169388,
278.462296651428));
#265647=CARTESIAN_POINT('Ctrl Pts',(-107.704469842635,72.9267251261949,
276.462296651428));
#265648=CARTESIAN_POINT('Ctrl Pts',(-101.965012102074,81.4032507354509,
274.462296651428));
#265649=CARTESIAN_POINT('Ctrl Pts',(-94.9701958612989,88.8775672472034,
272.462296651428));
#265650=CARTESIAN_POINT('Ctrl Pts',(-87.9753796205243,96.3518837589559,
270.462296651428));
#265651=CARTESIAN_POINT('Ctrl Pts',(-79.8974404698482,102.639948694851,
268.462296651428));
#265652=CARTESIAN_POINT('Ctrl Pts',(-71.819501319172,108.928013630747,266.462296651428));
#265653=CARTESIAN_POINT('Ctrl Pts',(-62.8573449296273,113.874993963172,
264.462296651428));
#265654=CARTESIAN_POINT('Ctrl Pts',(-53.8951885400826,118.821974295598,
262.462296651428));
#265655=CARTESIAN_POINT('Ctrl Pts',(-44.2694929456714,122.306058950682,
260.462296651428));
#265656=CARTESIAN_POINT('Ctrl Pts',(-34.6437973512603,125.790143605767,
258.462296651428));
#265657=CARTESIAN_POINT('Ctrl Pts',(-24.5915791233694,127.725542856289,
256.462296651428));
#265658=CARTESIAN_POINT('Ctrl Pts',(-14.5393608954786,129.660942106811,
254.462296651428));
#265659=CARTESIAN_POINT('Ctrl Pts',(-4.30813900827814,130.,252.462296651428));
#265660=CARTESIAN_POINT('Ctrl Pts',(5.92308287892232,130.339057893189,250.462296651428));
#265661=CARTESIAN_POINT('Ctrl Pts',(16.0813817870906,129.073425698447,248.462296651428));
#265662=CARTESIAN_POINT('Ctrl Pts',(26.2396806952589,127.807793503705,246.462296651428));
#265663=CARTESIAN_POINT('Ctrl Pts',(36.0749255918149,124.968635286058,244.462296651428));
#265664=CARTESIAN_POINT('Ctrl Pts',(45.9101704883709,122.129477068411,242.462296651428));
#265665=CARTESIAN_POINT('Ctrl Pts',(55.1801850026549,117.786702325803,240.462296651428));
#265666=CARTESIAN_POINT('Ctrl Pts',(64.4501995169388,113.443927583196,238.462296651428));
#265667=CARTESIAN_POINT('Ctrl Pts',(72.9267251261949,107.704469842635,236.462296651428));
#265668=CARTESIAN_POINT('Ctrl Pts',(81.4032507354509,101.965012102074,234.462296651428));
#265669=CARTESIAN_POINT('Ctrl Pts',(88.8775672472034,94.9701958612989,232.462296651428));
#265670=CARTESIAN_POINT('Ctrl Pts',(96.3518837589559,87.9753796205243,230.462296651428));
#265671=CARTESIAN_POINT('Ctrl Pts',(102.639948694851,79.8974404698482,228.462296651428));
#265672=CARTESIAN_POINT('Ctrl Pts',(108.928013630747,71.819501319172,226.462296651428));
#265673=CARTESIAN_POINT('Ctrl Pts',(113.874993963172,62.8573449296273,224.462296651428));
#265674=CARTESIAN_POINT('Ctrl Pts',(118.821974295598,53.8951885400826,222.462296651428));
#265675=CARTESIAN_POINT('Ctrl Pts',(122.306058950682,44.2694929456714,220.462296651428));
#265676=CARTESIAN_POINT('Ctrl Pts',(125.790143605767,34.6437973512603,218.462296651428));
#265677=CARTESIAN_POINT('Ctrl Pts',(127.725542856289,24.5915791233694,216.462296651428));
#265678=CARTESIAN_POINT('Ctrl Pts',(129.660942106811,14.5393608954786,214.462296651428));
#265679=CARTESIAN_POINT('Ctrl Pts',(130.,4.30813900827812,212.462296651428));
#265680=CARTESIAN_POINT('',(118.376086385729,-53.9041949546879,367.5));
#265681=CARTESIAN_POINT('Ctrl Pts',(118.376086385729,-53.9041949546878,
367.5));
#265682=CARTESIAN_POINT('Ctrl Pts',(119.546342407814,-51.276867586873,367.5));
#265683=CARTESIAN_POINT('Ctrl Pts',(120.634616850713,-48.6137313363232,
367.499999999997));
#265684=CARTESIAN_POINT('Ctrl Pts',(122.645087654721,-43.2205933565688,
367.499999999997));
#265685=CARTESIAN_POINT('Ctrl Pts',(123.566638088336,-40.4917272023246,
367.5));
#265686=CARTESIAN_POINT('Ctrl Pts',(126.073121396906,-32.2286687868894,
367.5));
#265687=CARTESIAN_POINT('Ctrl Pts',(127.399213018599,-26.6223327935022,
367.5));
#265688=CARTESIAN_POINT('Ctrl Pts',(128.373075022505,-20.9502666088246,
367.5));
#265689=CARTESIAN_POINT('',(130.,-4.30813900827807,377.537703348572));
#265690=CARTESIAN_POINT('Ctrl Pts',(130.,-4.30813900827807,377.537703348572));
#265691=CARTESIAN_POINT('Ctrl Pts',(129.660942106811,-14.5393608954785,
375.537703348572));
#265692=CARTESIAN_POINT('Ctrl Pts',(127.725542856289,-24.5915791233694,
373.537703348572));
#265693=CARTESIAN_POINT('Ctrl Pts',(125.790143605767,-34.6437973512603,
371.537703348572));
#265694=CARTESIAN_POINT('Ctrl Pts',(122.306058950682,-44.2694929456714,
369.537703348572));
#265695=CARTESIAN_POINT('Ctrl Pts',(120.533915146556,-49.1655039490629,
368.520423931127));
#265696=CARTESIAN_POINT('Ctrl Pts',(118.376086385729,-53.9041949546879,
367.5));
#265697=CARTESIAN_POINT('',(130.,2.68882138776405E-14,375.));
#265698=CARTESIAN_POINT('Ctrl Pts',(160.,-4.30813900827805,377.537703348572));
#265699=CARTESIAN_POINT('Ctrl Pts',(159.660942106811,-16.900412100217,375.537703348572));
#265700=CARTESIAN_POINT('Ctrl Pts',(157.356193074143,-29.2846130745763,
373.537703348572));
#265701=CARTESIAN_POINT('Ctrl Pts',(155.051444041475,-41.6688140489355,
371.537703348572));
#265702=CARTESIAN_POINT('Ctrl Pts',(150.837754439537,-53.5400027769198,
369.537703348572));
#265703=CARTESIAN_POINT('Ctrl Pts',(146.624064837599,-65.411191504904,367.537703348572));
#265704=CARTESIAN_POINT('Ctrl Pts',(140.605189688823,-76.4770599218136,
365.537703348572));
#265705=CARTESIAN_POINT('Ctrl Pts',(134.586314540048,-87.5429283387233,
363.537703348572));
#265706=CARTESIAN_POINT('Ctrl Pts',(126.9104585261,-97.5309980386223,361.537703348572));
#265707=CARTESIAN_POINT('Ctrl Pts',(119.234602512152,-107.519067738521,
359.537703348572));
#265708=CARTESIAN_POINT('Ctrl Pts',(110.0907706828,-116.183399296895,357.537703348572));
#265709=CARTESIAN_POINT('Ctrl Pts',(100.946938853448,-124.847730855269,
355.537703348572));
#265710=CARTESIAN_POINT('Ctrl Pts',(90.5602826949691,-131.974979673883,
353.537703348572));
#265711=CARTESIAN_POINT('Ctrl Pts',(80.1736265364902,-139.102228492497,
351.537703348572));
#265712=CARTESIAN_POINT('Ctrl Pts',(68.7998999948414,-144.516898051454,
349.537703348572));
#265713=CARTESIAN_POINT('Ctrl Pts',(57.4261734531925,-149.931567610412,
347.537703348572));
#265714=CARTESIAN_POINT('Ctrl Pts',(45.3454354230634,-153.500330774912,
345.537703348572));
#265715=CARTESIAN_POINT('Ctrl Pts',(33.2646973929343,-157.069093939413,
343.537703348572));
#265716=CARTESIAN_POINT('Ctrl Pts',(20.7744157382976,-158.704075916301,
341.537703348572));
#265717=CARTESIAN_POINT('Ctrl Pts',(8.28413408366091,-160.339057893189,
339.537703348572));
#265718=CARTESIAN_POINT('Ctrl Pts',(-4.30813900827804,-160.,337.537703348572));
#265719=CARTESIAN_POINT('Ctrl Pts',(-16.900412100217,-159.660942106811,
335.537703348572));
#265720=CARTESIAN_POINT('Ctrl Pts',(-29.2846130745763,-157.356193074143,
333.537703348572));
#265721=CARTESIAN_POINT('Ctrl Pts',(-41.6688140489355,-155.051444041475,
331.537703348572));
#265722=CARTESIAN_POINT('Ctrl Pts',(-53.5400027769198,-150.837754439537,
329.537703348572));
#265723=CARTESIAN_POINT('Ctrl Pts',(-65.411191504904,-146.624064837599,
327.537703348572));
#265724=CARTESIAN_POINT('Ctrl Pts',(-76.4770599218136,-140.605189688823,
325.537703348572));
#265725=CARTESIAN_POINT('Ctrl Pts',(-87.5429283387233,-134.586314540048,
323.537703348572));
#265726=CARTESIAN_POINT('Ctrl Pts',(-97.5309980386223,-126.9104585261,321.537703348572));
#265727=CARTESIAN_POINT('Ctrl Pts',(-107.519067738521,-119.234602512152,
319.537703348572));
#265728=CARTESIAN_POINT('Ctrl Pts',(-116.183399296895,-110.0907706828,317.537703348572));
#265729=CARTESIAN_POINT('Ctrl Pts',(-124.847730855269,-100.946938853448,
315.537703348572));
#265730=CARTESIAN_POINT('Ctrl Pts',(-131.974979673883,-90.5602826949692,
313.537703348572));
#265731=CARTESIAN_POINT('Ctrl Pts',(-139.102228492497,-80.1736265364902,
311.537703348572));
#265732=CARTESIAN_POINT('Ctrl Pts',(-144.516898051454,-68.7998999948414,
309.537703348572));
#265733=CARTESIAN_POINT('Ctrl Pts',(-149.931567610412,-57.4261734531925,
307.537703348572));
#265734=CARTESIAN_POINT('Ctrl Pts',(-153.500330774912,-45.3454354230634,
305.537703348572));
#265735=CARTESIAN_POINT('Ctrl Pts',(-157.069093939413,-33.2646973929344,
303.537703348572));
#265736=CARTESIAN_POINT('Ctrl Pts',(-158.704075916301,-20.7744157382976,
301.537703348572));
#265737=CARTESIAN_POINT('Ctrl Pts',(-160.339057893189,-8.28413408366092,
299.537703348572));
#265738=CARTESIAN_POINT('Ctrl Pts',(-160.,4.30813900827803,297.537703348572));
#265739=CARTESIAN_POINT('Ctrl Pts',(-159.660942106811,16.900412100217,295.537703348572));
#265740=CARTESIAN_POINT('Ctrl Pts',(-157.356193074143,29.2846130745763,
293.537703348572));
#265741=CARTESIAN_POINT('Ctrl Pts',(-155.051444041475,41.6688140489355,
291.537703348572));
#265742=CARTESIAN_POINT('Ctrl Pts',(-150.837754439537,53.5400027769198,
289.537703348572));
#265743=CARTESIAN_POINT('Ctrl Pts',(-146.624064837599,65.411191504904,287.537703348572));
#265744=CARTESIAN_POINT('Ctrl Pts',(-140.605189688823,76.4770599218136,
285.537703348572));
#265745=CARTESIAN_POINT('Ctrl Pts',(-134.586314540048,87.5429283387233,
283.537703348572));
#265746=CARTESIAN_POINT('Ctrl Pts',(-126.9104585261,97.5309980386223,281.537703348572));
#265747=CARTESIAN_POINT('Ctrl Pts',(-119.234602512152,107.519067738521,
279.537703348572));
#265748=CARTESIAN_POINT('Ctrl Pts',(-110.0907706828,116.183399296895,277.537703348572));
#265749=CARTESIAN_POINT('Ctrl Pts',(-100.946938853448,124.847730855269,
275.537703348572));
#265750=CARTESIAN_POINT('Ctrl Pts',(-90.5602826949692,131.974979673883,
273.537703348572));
#265751=CARTESIAN_POINT('Ctrl Pts',(-80.1736265364901,139.102228492497,
271.537703348572));
#265752=CARTESIAN_POINT('Ctrl Pts',(-68.7998999948414,144.516898051454,
269.537703348572));
#265753=CARTESIAN_POINT('Ctrl Pts',(-57.4261734531926,149.931567610412,
267.537703348572));
#265754=CARTESIAN_POINT('Ctrl Pts',(-45.3454354230634,153.500330774912,
265.537703348572));
#265755=CARTESIAN_POINT('Ctrl Pts',(-33.2646973929343,157.069093939413,
263.537703348572));
#265756=CARTESIAN_POINT('Ctrl Pts',(-20.7744157382976,158.704075916301,
261.537703348572));
#265757=CARTESIAN_POINT('Ctrl Pts',(-8.284134083661,160.339057893189,259.537703348572));
#265758=CARTESIAN_POINT('Ctrl Pts',(4.30813900827803,160.,257.537703348572));
#265759=CARTESIAN_POINT('Ctrl Pts',(16.9004121002171,159.660942106811,255.537703348572));
#265760=CARTESIAN_POINT('Ctrl Pts',(29.2846130745762,157.356193074143,253.537703348572));
#265761=CARTESIAN_POINT('Ctrl Pts',(41.6688140489354,155.051444041476,251.537703348572));
#265762=CARTESIAN_POINT('Ctrl Pts',(53.5400027769198,150.837754439537,249.537703348572));
#265763=CARTESIAN_POINT('Ctrl Pts',(65.4111915049041,146.624064837599,247.537703348572));
#265764=CARTESIAN_POINT('Ctrl Pts',(76.4770599218136,140.605189688823,245.537703348572));
#265765=CARTESIAN_POINT('Ctrl Pts',(87.5429283387232,134.586314540048,243.537703348572));
#265766=CARTESIAN_POINT('Ctrl Pts',(97.5309980386223,126.9104585261,241.537703348572));
#265767=CARTESIAN_POINT('Ctrl Pts',(107.519067738521,119.234602512152,239.537703348572));
#265768=CARTESIAN_POINT('Ctrl Pts',(116.183399296895,110.0907706828,237.537703348572));
#265769=CARTESIAN_POINT('Ctrl Pts',(124.847730855269,100.946938853448,235.537703348572));
#265770=CARTESIAN_POINT('Ctrl Pts',(131.974979673883,90.5602826949692,233.537703348572));
#265771=CARTESIAN_POINT('Ctrl Pts',(139.102228492497,80.1736265364902,231.537703348572));
#265772=CARTESIAN_POINT('Ctrl Pts',(144.516898051454,68.7998999948414,229.537703348572));
#265773=CARTESIAN_POINT('Ctrl Pts',(149.931567610412,57.4261734531926,227.537703348572));
#265774=CARTESIAN_POINT('Ctrl Pts',(153.500330774912,45.3454354230634,225.537703348572));
#265775=CARTESIAN_POINT('Ctrl Pts',(157.069093939413,33.2646973929343,223.537703348572));
#265776=CARTESIAN_POINT('Ctrl Pts',(158.704075916301,20.7744157382976,221.537703348572));
#265777=CARTESIAN_POINT('Ctrl Pts',(160.339057893189,8.28413408366101,219.537703348572));
#265778=CARTESIAN_POINT('Ctrl Pts',(160.,-4.30813900827805,217.537703348572));
#265779=CARTESIAN_POINT('Ctrl Pts',(130.,-4.30813900827807,377.537703348572));
#265780=CARTESIAN_POINT('Ctrl Pts',(129.660942106811,-14.5393608954785,
375.537703348572));
#265781=CARTESIAN_POINT('Ctrl Pts',(127.725542856289,-24.5915791233694,
373.537703348572));
#265782=CARTESIAN_POINT('Ctrl Pts',(125.790143605767,-34.6437973512603,
371.537703348572));
#265783=CARTESIAN_POINT('Ctrl Pts',(122.306058950682,-44.2694929456714,
369.537703348572));
#265784=CARTESIAN_POINT('Ctrl Pts',(118.821974295598,-53.8951885400825,
367.537703348572));
#265785=CARTESIAN_POINT('Ctrl Pts',(113.874993963172,-62.8573449296272,
365.537703348572));
#265786=CARTESIAN_POINT('Ctrl Pts',(108.928013630747,-71.819501319172,363.537703348572));
#265787=CARTESIAN_POINT('Ctrl Pts',(102.639948694851,-79.8974404698481,
361.537703348572));
#265788=CARTESIAN_POINT('Ctrl Pts',(96.351883758956,-87.9753796205242,359.537703348572));
#265789=CARTESIAN_POINT('Ctrl Pts',(88.8775672472035,-94.9701958612989,
357.537703348572));
#265790=CARTESIAN_POINT('Ctrl Pts',(81.403250735451,-101.965012102074,355.537703348572));
#265791=CARTESIAN_POINT('Ctrl Pts',(72.9267251261949,-107.704469842635,
353.537703348572));
#265792=CARTESIAN_POINT('Ctrl Pts',(64.4501995169389,-113.443927583196,
351.537703348572));
#265793=CARTESIAN_POINT('Ctrl Pts',(55.1801850026549,-117.786702325803,
349.537703348572));
#265794=CARTESIAN_POINT('Ctrl Pts',(45.910170488371,-122.129477068411,347.537703348572));
#265795=CARTESIAN_POINT('Ctrl Pts',(36.074925591815,-124.968635286058,345.537703348572));
#265796=CARTESIAN_POINT('Ctrl Pts',(26.239680695259,-127.807793503704,343.537703348572));
#265797=CARTESIAN_POINT('Ctrl Pts',(16.0813817870907,-129.073425698447,
341.537703348572));
#265798=CARTESIAN_POINT('Ctrl Pts',(5.92308287892234,-130.339057893189,
339.537703348572));
#265799=CARTESIAN_POINT('Ctrl Pts',(-4.30813900827806,-130.,337.537703348572));
#265800=CARTESIAN_POINT('Ctrl Pts',(-14.5393608954785,-129.660942106811,
335.537703348572));
#265801=CARTESIAN_POINT('Ctrl Pts',(-24.5915791233694,-127.725542856289,
333.537703348572));
#265802=CARTESIAN_POINT('Ctrl Pts',(-34.6437973512603,-125.790143605767,
331.537703348572));
#265803=CARTESIAN_POINT('Ctrl Pts',(-44.2694929456713,-122.306058950682,
329.537703348572));
#265804=CARTESIAN_POINT('Ctrl Pts',(-53.8951885400825,-118.821974295598,
327.537703348572));
#265805=CARTESIAN_POINT('Ctrl Pts',(-62.8573449296272,-113.874993963172,
325.537703348572));
#265806=CARTESIAN_POINT('Ctrl Pts',(-71.819501319172,-108.928013630747,
323.537703348572));
#265807=CARTESIAN_POINT('Ctrl Pts',(-79.8974404698481,-102.639948694851,
321.537703348572));
#265808=CARTESIAN_POINT('Ctrl Pts',(-87.9753796205242,-96.351883758956,
319.537703348572));
#265809=CARTESIAN_POINT('Ctrl Pts',(-94.9701958612989,-88.8775672472035,
317.537703348572));
#265810=CARTESIAN_POINT('Ctrl Pts',(-101.965012102074,-81.403250735451,
315.537703348572));
#265811=CARTESIAN_POINT('Ctrl Pts',(-107.704469842635,-72.9267251261949,
313.537703348572));
#265812=CARTESIAN_POINT('Ctrl Pts',(-113.443927583196,-64.4501995169389,
311.537703348572));
#265813=CARTESIAN_POINT('Ctrl Pts',(-117.786702325803,-55.1801850026549,
309.537703348572));
#265814=CARTESIAN_POINT('Ctrl Pts',(-122.129477068411,-45.910170488371,
307.537703348572));
#265815=CARTESIAN_POINT('Ctrl Pts',(-124.968635286058,-36.074925591815,
305.537703348572));
#265816=CARTESIAN_POINT('Ctrl Pts',(-127.807793503704,-26.239680695259,
303.537703348572));
#265817=CARTESIAN_POINT('Ctrl Pts',(-129.073425698447,-16.0813817870907,
301.537703348572));
#265818=CARTESIAN_POINT('Ctrl Pts',(-130.339057893189,-5.92308287892235,
299.537703348572));
#265819=CARTESIAN_POINT('Ctrl Pts',(-130.,4.30813900827805,297.537703348572));
#265820=CARTESIAN_POINT('Ctrl Pts',(-129.660942106811,14.5393608954784,
295.537703348572));
#265821=CARTESIAN_POINT('Ctrl Pts',(-127.725542856289,24.5915791233693,
293.537703348572));
#265822=CARTESIAN_POINT('Ctrl Pts',(-125.790143605767,34.6437973512602,
291.537703348572));
#265823=CARTESIAN_POINT('Ctrl Pts',(-122.306058950682,44.2694929456713,
289.537703348572));
#265824=CARTESIAN_POINT('Ctrl Pts',(-118.821974295598,53.8951885400825,
287.537703348572));
#265825=CARTESIAN_POINT('Ctrl Pts',(-113.874993963172,62.8573449296272,
285.537703348572));
#265826=CARTESIAN_POINT('Ctrl Pts',(-108.928013630747,71.819501319172,283.537703348572));
#265827=CARTESIAN_POINT('Ctrl Pts',(-102.639948694851,79.8974404698481,
281.537703348572));
#265828=CARTESIAN_POINT('Ctrl Pts',(-96.3518837589561,87.9753796205242,
279.537703348572));
#265829=CARTESIAN_POINT('Ctrl Pts',(-88.8775672472035,94.9701958612989,
277.537703348572));
#265830=CARTESIAN_POINT('Ctrl Pts',(-81.403250735451,101.965012102074,275.537703348572));
#265831=CARTESIAN_POINT('Ctrl Pts',(-72.9267251261949,107.704469842635,
273.537703348572));
#265832=CARTESIAN_POINT('Ctrl Pts',(-64.4501995169389,113.443927583196,
271.537703348572));
#265833=CARTESIAN_POINT('Ctrl Pts',(-55.1801850026549,117.786702325803,
269.537703348572));
#265834=CARTESIAN_POINT('Ctrl Pts',(-45.910170488371,122.129477068411,267.537703348572));
#265835=CARTESIAN_POINT('Ctrl Pts',(-36.074925591815,124.968635286058,265.537703348572));
#265836=CARTESIAN_POINT('Ctrl Pts',(-26.239680695259,127.807793503704,263.537703348572));
#265837=CARTESIAN_POINT('Ctrl Pts',(-16.0813817870907,129.073425698447,
261.537703348572));
#265838=CARTESIAN_POINT('Ctrl Pts',(-5.92308287892242,130.339057893189,
259.537703348572));
#265839=CARTESIAN_POINT('Ctrl Pts',(4.30813900827804,130.,257.537703348572));
#265840=CARTESIAN_POINT('Ctrl Pts',(14.5393608954785,129.660942106811,255.537703348572));
#265841=CARTESIAN_POINT('Ctrl Pts',(24.5915791233693,127.725542856289,253.537703348572));
#265842=CARTESIAN_POINT('Ctrl Pts',(34.6437973512602,125.790143605767,251.537703348572));
#265843=CARTESIAN_POINT('Ctrl Pts',(44.2694929456713,122.306058950682,249.537703348572));
#265844=CARTESIAN_POINT('Ctrl Pts',(53.8951885400825,118.821974295598,247.537703348572));
#265845=CARTESIAN_POINT('Ctrl Pts',(62.8573449296272,113.874993963172,245.537703348572));
#265846=CARTESIAN_POINT('Ctrl Pts',(71.819501319172,108.928013630747,243.537703348572));
#265847=CARTESIAN_POINT('Ctrl Pts',(79.8974404698481,102.639948694851,241.537703348572));
#265848=CARTESIAN_POINT('Ctrl Pts',(87.9753796205242,96.351883758956,239.537703348572));
#265849=CARTESIAN_POINT('Ctrl Pts',(94.9701958612989,88.8775672472035,237.537703348572));
#265850=CARTESIAN_POINT('Ctrl Pts',(101.965012102074,81.403250735451,235.537703348572));
#265851=CARTESIAN_POINT('Ctrl Pts',(107.704469842635,72.926725126195,233.537703348572));
#265852=CARTESIAN_POINT('Ctrl Pts',(113.443927583196,64.4501995169389,231.537703348572));
#265853=CARTESIAN_POINT('Ctrl Pts',(117.786702325803,55.1801850026549,229.537703348572));
#265854=CARTESIAN_POINT('Ctrl Pts',(122.129477068411,45.910170488371,227.537703348572));
#265855=CARTESIAN_POINT('Ctrl Pts',(124.968635286058,36.074925591815,225.537703348572));
#265856=CARTESIAN_POINT('Ctrl Pts',(127.807793503704,26.239680695259,223.537703348572));
#265857=CARTESIAN_POINT('Ctrl Pts',(129.073425698447,16.0813817870907,221.537703348572));
#265858=CARTESIAN_POINT('Ctrl Pts',(130.339057893189,5.92308287892242,219.537703348572));
#265859=CARTESIAN_POINT('Ctrl Pts',(130.,-4.30813900827807,217.537703348572));
#265860=CARTESIAN_POINT('',(146.075461400194,-65.4256802672709,367.5));
#265861=CARTESIAN_POINT('',(145.,-4.30813900827806,377.537703348572));
#265862=CARTESIAN_POINT('Origin',(160.,3.64291929955129E-14,375.));
#265863=CARTESIAN_POINT('Origin',(-160.,-160.339057893189,367.5));
#265864=CARTESIAN_POINT('Ctrl Pts',(-130.,4.30813900827773,377.537703348572));
#265865=CARTESIAN_POINT('Ctrl Pts',(-129.660942106811,14.5393608954781,
375.537703348572));
#265866=CARTESIAN_POINT('Ctrl Pts',(-127.725542856289,24.591579123369,373.537703348572));
#265867=CARTESIAN_POINT('Ctrl Pts',(-125.790143605767,34.6437973512599,
371.537703348572));
#265868=CARTESIAN_POINT('Ctrl Pts',(-122.306058950683,44.269492945671,369.537703348572));
#265869=CARTESIAN_POINT('Ctrl Pts',(-118.821974295598,53.8951885400822,
367.537703348572));
#265870=CARTESIAN_POINT('Ctrl Pts',(-113.874993963172,62.8573449296269,
365.537703348572));
#265871=CARTESIAN_POINT('Ctrl Pts',(-108.928013630747,71.8195013191717,
363.537703348572));
#265872=CARTESIAN_POINT('Ctrl Pts',(-102.639948694852,79.8974404698478,
361.537703348572));
#265873=CARTESIAN_POINT('Ctrl Pts',(-96.3518837589562,87.9753796205239,
359.537703348572));
#265874=CARTESIAN_POINT('Ctrl Pts',(-88.8775672472037,94.9701958612987,
357.537703348572));
#265875=CARTESIAN_POINT('Ctrl Pts',(-81.4032507354512,101.965012102073,
355.537703348572));
#265876=CARTESIAN_POINT('Ctrl Pts',(-72.9267251261952,107.704469842635,
353.537703348572));
#265877=CARTESIAN_POINT('Ctrl Pts',(-64.4501995169392,113.443927583196,
351.537703348572));
#265878=CARTESIAN_POINT('Ctrl Pts',(-55.1801850026552,117.786702325803,
349.537703348572));
#265879=CARTESIAN_POINT('Ctrl Pts',(-45.9101704883713,122.12947706841,347.537703348572));
#265880=CARTESIAN_POINT('Ctrl Pts',(-36.0749255918153,124.968635286057,
345.537703348572));
#265881=CARTESIAN_POINT('Ctrl Pts',(-26.2396806952593,127.807793503704,
343.537703348572));
#265882=CARTESIAN_POINT('Ctrl Pts',(-16.081381787091,129.073425698447,341.537703348572));
#265883=CARTESIAN_POINT('Ctrl Pts',(-5.92308287892268,130.339057893189,
339.537703348572));
#265884=CARTESIAN_POINT('Ctrl Pts',(4.30813900827772,130.,337.537703348572));
#265885=CARTESIAN_POINT('Ctrl Pts',(14.5393608954781,129.660942106811,335.537703348572));
#265886=CARTESIAN_POINT('Ctrl Pts',(24.591579123369,127.725542856289,333.537703348572));
#265887=CARTESIAN_POINT('Ctrl Pts',(34.6437973512599,125.790143605767,331.537703348572));
#265888=CARTESIAN_POINT('Ctrl Pts',(44.269492945671,122.306058950683,329.537703348572));
#265889=CARTESIAN_POINT('Ctrl Pts',(53.8951885400822,118.821974295598,327.537703348572));
#265890=CARTESIAN_POINT('Ctrl Pts',(62.8573449296269,113.874993963172,325.537703348572));
#265891=CARTESIAN_POINT('Ctrl Pts',(71.8195013191717,108.928013630747,323.537703348572));
#265892=CARTESIAN_POINT('Ctrl Pts',(79.8974404698478,102.639948694852,321.537703348572));
#265893=CARTESIAN_POINT('Ctrl Pts',(87.9753796205239,96.3518837589562,319.537703348572));
#265894=CARTESIAN_POINT('Ctrl Pts',(94.9701958612986,88.8775672472037,317.537703348572));
#265895=CARTESIAN_POINT('Ctrl Pts',(101.965012102073,81.4032507354512,315.537703348572));
#265896=CARTESIAN_POINT('Ctrl Pts',(107.704469842635,72.9267251261952,313.537703348572));
#265897=CARTESIAN_POINT('Ctrl Pts',(113.443927583196,64.4501995169392,311.537703348572));
#265898=CARTESIAN_POINT('Ctrl Pts',(117.786702325803,55.1801850026552,309.537703348572));
#265899=CARTESIAN_POINT('Ctrl Pts',(122.12947706841,45.9101704883713,307.537703348572));
#265900=CARTESIAN_POINT('Ctrl Pts',(124.968635286057,36.0749255918153,305.537703348572));
#265901=CARTESIAN_POINT('Ctrl Pts',(127.807793503704,26.2396806952593,303.537703348572));
#265902=CARTESIAN_POINT('Ctrl Pts',(129.073425698447,16.081381787091,301.537703348572));
#265903=CARTESIAN_POINT('Ctrl Pts',(130.339057893189,5.92308287892268,299.537703348572));
#265904=CARTESIAN_POINT('Ctrl Pts',(130.,-4.30813900827772,297.537703348572));
#265905=CARTESIAN_POINT('Ctrl Pts',(129.660942106811,-14.5393608954781,
295.537703348572));
#265906=CARTESIAN_POINT('Ctrl Pts',(127.725542856289,-24.591579123369,293.537703348572));
#265907=CARTESIAN_POINT('Ctrl Pts',(125.790143605767,-34.6437973512599,
291.537703348572));
#265908=CARTESIAN_POINT('Ctrl Pts',(122.306058950683,-44.269492945671,289.537703348572));
#265909=CARTESIAN_POINT('Ctrl Pts',(118.821974295598,-53.8951885400822,
287.537703348572));
#265910=CARTESIAN_POINT('Ctrl Pts',(113.874993963172,-62.8573449296269,
285.537703348572));
#265911=CARTESIAN_POINT('Ctrl Pts',(108.928013630747,-71.8195013191717,
283.537703348572));
#265912=CARTESIAN_POINT('Ctrl Pts',(102.639948694852,-79.8974404698478,
281.537703348572));
#265913=CARTESIAN_POINT('Ctrl Pts',(96.3518837589563,-87.9753796205239,
279.537703348572));
#265914=CARTESIAN_POINT('Ctrl Pts',(88.8775672472037,-94.9701958612986,
277.537703348572));
#265915=CARTESIAN_POINT('Ctrl Pts',(81.4032507354513,-101.965012102073,
275.537703348572));
#265916=CARTESIAN_POINT('Ctrl Pts',(72.9267251261952,-107.704469842635,
273.537703348572));
#265917=CARTESIAN_POINT('Ctrl Pts',(64.4501995169392,-113.443927583196,
271.537703348572));
#265918=CARTESIAN_POINT('Ctrl Pts',(55.1801850026552,-117.786702325803,
269.537703348572));
#265919=CARTESIAN_POINT('Ctrl Pts',(45.9101704883713,-122.12947706841,267.537703348572));
#265920=CARTESIAN_POINT('Ctrl Pts',(36.0749255918153,-124.968635286057,
265.537703348572));
#265921=CARTESIAN_POINT('Ctrl Pts',(26.2396806952593,-127.807793503704,
263.537703348572));
#265922=CARTESIAN_POINT('Ctrl Pts',(16.081381787091,-129.073425698447,261.537703348572));
#265923=CARTESIAN_POINT('Ctrl Pts',(5.92308287892275,-130.339057893189,
259.537703348572));
#265924=CARTESIAN_POINT('Ctrl Pts',(-4.30813900827771,-130.,257.537703348572));
#265925=CARTESIAN_POINT('Ctrl Pts',(-14.5393608954782,-129.660942106811,
255.537703348572));
#265926=CARTESIAN_POINT('Ctrl Pts',(-24.591579123369,-127.725542856289,
253.537703348572));
#265927=CARTESIAN_POINT('Ctrl Pts',(-34.6437973512598,-125.790143605767,
251.537703348572));
#265928=CARTESIAN_POINT('Ctrl Pts',(-44.269492945671,-122.306058950683,
249.537703348572));
#265929=CARTESIAN_POINT('Ctrl Pts',(-53.8951885400822,-118.821974295598,
247.537703348572));
#265930=CARTESIAN_POINT('Ctrl Pts',(-62.8573449296269,-113.874993963172,
245.537703348572));
#265931=CARTESIAN_POINT('Ctrl Pts',(-71.8195013191717,-108.928013630747,
243.537703348572));
#265932=CARTESIAN_POINT('Ctrl Pts',(-79.8974404698478,-102.639948694852,
241.537703348572));
#265933=CARTESIAN_POINT('Ctrl Pts',(-87.975379620524,-96.3518837589562,
239.537703348572));
#265934=CARTESIAN_POINT('Ctrl Pts',(-94.9701958612986,-88.8775672472037,
237.537703348572));
#265935=CARTESIAN_POINT('Ctrl Pts',(-101.965012102073,-81.4032507354513,
235.537703348572));
#265936=CARTESIAN_POINT('Ctrl Pts',(-107.704469842635,-72.9267251261952,
233.537703348572));
#265937=CARTESIAN_POINT('Ctrl Pts',(-113.443927583196,-64.4501995169392,
231.537703348572));
#265938=CARTESIAN_POINT('Ctrl Pts',(-117.786702325803,-55.1801850026553,
229.537703348572));
#265939=CARTESIAN_POINT('Ctrl Pts',(-122.12947706841,-45.9101704883713,
227.537703348572));
#265940=CARTESIAN_POINT('Ctrl Pts',(-124.968635286057,-36.0749255918153,
225.537703348572));
#265941=CARTESIAN_POINT('Ctrl Pts',(-127.807793503704,-26.2396806952593,
223.537703348572));
#265942=CARTESIAN_POINT('Ctrl Pts',(-129.073425698447,-16.081381787091,
221.537703348572));
#265943=CARTESIAN_POINT('Ctrl Pts',(-130.339057893189,-5.92308287892275,
219.537703348572));
#265944=CARTESIAN_POINT('Ctrl Pts',(-130.,4.30813900827773,217.537703348572));
#265945=CARTESIAN_POINT('Ctrl Pts',(-130.,-4.30813900827845,372.462296651428));
#265946=CARTESIAN_POINT('Ctrl Pts',(-130.339057893189,5.92308287892195,
370.462296651428));
#265947=CARTESIAN_POINT('Ctrl Pts',(-129.073425698447,16.0813817870903,
368.462296651429));
#265948=CARTESIAN_POINT('Ctrl Pts',(-127.807793503705,26.2396806952586,
366.462296651429));
#265949=CARTESIAN_POINT('Ctrl Pts',(-124.968635286058,36.0749255918146,
364.462296651428));
#265950=CARTESIAN_POINT('Ctrl Pts',(-122.129477068411,45.9101704883706,
362.462296651428));
#265951=CARTESIAN_POINT('Ctrl Pts',(-117.786702325804,55.1801850026546,
360.462296651428));
#265952=CARTESIAN_POINT('Ctrl Pts',(-113.443927583196,64.4501995169386,
358.462296651428));
#265953=CARTESIAN_POINT('Ctrl Pts',(-107.704469842635,72.9267251261946,
356.462296651428));
#265954=CARTESIAN_POINT('Ctrl Pts',(-101.965012102074,81.4032507354507,
354.462296651428));
#265955=CARTESIAN_POINT('Ctrl Pts',(-94.9701958612992,88.8775672472032,
352.462296651428));
#265956=CARTESIAN_POINT('Ctrl Pts',(-87.9753796205245,96.3518837589558,
350.462296651428));
#265957=CARTESIAN_POINT('Ctrl Pts',(-79.8974404698484,102.639948694851,
348.462296651428));
#265958=CARTESIAN_POINT('Ctrl Pts',(-71.8195013191724,108.928013630747,
346.462296651428));
#265959=CARTESIAN_POINT('Ctrl Pts',(-62.8573449296276,113.874993963172,
344.462296651428));
#265960=CARTESIAN_POINT('Ctrl Pts',(-53.8951885400828,118.821974295598,
342.462296651428));
#265961=CARTESIAN_POINT('Ctrl Pts',(-44.2694929456717,122.306058950682,
340.462296651428));
#265962=CARTESIAN_POINT('Ctrl Pts',(-34.6437973512606,125.790143605767,
338.462296651428));
#265963=CARTESIAN_POINT('Ctrl Pts',(-24.5915791233697,127.725542856289,
336.462296651428));
#265964=CARTESIAN_POINT('Ctrl Pts',(-14.5393608954789,129.660942106811,
334.462296651428));
#265965=CARTESIAN_POINT('Ctrl Pts',(-4.30813900827846,130.,332.462296651428));
#265966=CARTESIAN_POINT('Ctrl Pts',(5.92308287892194,130.339057893189,330.462296651429));
#265967=CARTESIAN_POINT('Ctrl Pts',(16.0813817870903,129.073425698447,328.462296651428));
#265968=CARTESIAN_POINT('Ctrl Pts',(26.2396806952586,127.807793503705,326.462296651428));
#265969=CARTESIAN_POINT('Ctrl Pts',(36.0749255918146,124.968635286058,324.462296651428));
#265970=CARTESIAN_POINT('Ctrl Pts',(45.9101704883706,122.129477068411,322.462296651428));
#265971=CARTESIAN_POINT('Ctrl Pts',(55.1801850026546,117.786702325804,320.462296651428));
#265972=CARTESIAN_POINT('Ctrl Pts',(64.4501995169386,113.443927583196,318.462296651428));
#265973=CARTESIAN_POINT('Ctrl Pts',(72.9267251261946,107.704469842635,316.462296651428));
#265974=CARTESIAN_POINT('Ctrl Pts',(81.4032507354506,101.965012102074,314.462296651428));
#265975=CARTESIAN_POINT('Ctrl Pts',(88.8775672472032,94.9701958612992,312.462296651428));
#265976=CARTESIAN_POINT('Ctrl Pts',(96.3518837589558,87.9753796205245,310.462296651428));
#265977=CARTESIAN_POINT('Ctrl Pts',(102.639948694851,79.8974404698484,308.462296651428));
#265978=CARTESIAN_POINT('Ctrl Pts',(108.928013630747,71.8195013191724,306.462296651428));
#265979=CARTESIAN_POINT('Ctrl Pts',(113.874993963172,62.8573449296276,304.462296651428));
#265980=CARTESIAN_POINT('Ctrl Pts',(118.821974295598,53.8951885400829,302.462296651428));
#265981=CARTESIAN_POINT('Ctrl Pts',(122.306058950682,44.2694929456717,300.462296651428));
#265982=CARTESIAN_POINT('Ctrl Pts',(125.790143605767,34.6437973512606,298.462296651428));
#265983=CARTESIAN_POINT('Ctrl Pts',(127.725542856289,24.5915791233698,296.462296651428));
#265984=CARTESIAN_POINT('Ctrl Pts',(129.660942106811,14.5393608954789,294.462296651429));
#265985=CARTESIAN_POINT('Ctrl Pts',(130.,4.30813900827846,292.462296651428));
#265986=CARTESIAN_POINT('Ctrl Pts',(130.339057893189,-5.92308287892194,
290.462296651428));
#265987=CARTESIAN_POINT('Ctrl Pts',(129.073425698447,-16.0813817870903,
288.462296651428));
#265988=CARTESIAN_POINT('Ctrl Pts',(127.807793503705,-26.2396806952586,
286.462296651428));
#265989=CARTESIAN_POINT('Ctrl Pts',(124.968635286058,-36.0749255918146,
284.462296651428));
#265990=CARTESIAN_POINT('Ctrl Pts',(122.129477068411,-45.9101704883706,
282.462296651428));
#265991=CARTESIAN_POINT('Ctrl Pts',(117.786702325804,-55.1801850026546,
280.462296651428));
#265992=CARTESIAN_POINT('Ctrl Pts',(113.443927583196,-64.4501995169386,
278.462296651428));
#265993=CARTESIAN_POINT('Ctrl Pts',(107.704469842635,-72.9267251261946,
276.462296651428));
#265994=CARTESIAN_POINT('Ctrl Pts',(101.965012102074,-81.4032507354506,
274.462296651428));
#265995=CARTESIAN_POINT('Ctrl Pts',(94.9701958612992,-88.8775672472032,
272.462296651428));
#265996=CARTESIAN_POINT('Ctrl Pts',(87.9753796205246,-96.3518837589557,
270.462296651428));
#265997=CARTESIAN_POINT('Ctrl Pts',(79.8974404698484,-102.639948694851,
268.462296651428));
#265998=CARTESIAN_POINT('Ctrl Pts',(71.8195013191723,-108.928013630747,
266.462296651428));
#265999=CARTESIAN_POINT('Ctrl Pts',(62.8573449296276,-113.874993963172,
264.462296651428));
#266000=CARTESIAN_POINT('Ctrl Pts',(53.8951885400829,-118.821974295598,
262.462296651428));
#266001=CARTESIAN_POINT('Ctrl Pts',(44.2694929456717,-122.306058950682,
260.462296651428));
#266002=CARTESIAN_POINT('Ctrl Pts',(34.6437973512606,-125.790143605767,
258.462296651428));
#266003=CARTESIAN_POINT('Ctrl Pts',(24.5915791233698,-127.725542856289,
256.462296651428));
#266004=CARTESIAN_POINT('Ctrl Pts',(14.5393608954789,-129.660942106811,
254.462296651428));
#266005=CARTESIAN_POINT('Ctrl Pts',(4.30813900827847,-130.,252.462296651428));
#266006=CARTESIAN_POINT('Ctrl Pts',(-5.92308287892199,-130.339057893189,
250.462296651428));
#266007=CARTESIAN_POINT('Ctrl Pts',(-16.0813817870903,-129.073425698447,
248.462296651428));
#266008=CARTESIAN_POINT('Ctrl Pts',(-26.2396806952585,-127.807793503705,
246.462296651428));
#266009=CARTESIAN_POINT('Ctrl Pts',(-36.0749255918146,-124.968635286058,
244.462296651428));
#266010=CARTESIAN_POINT('Ctrl Pts',(-45.9101704883706,-122.129477068411,
242.462296651428));
#266011=CARTESIAN_POINT('Ctrl Pts',(-55.1801850026546,-117.786702325804,
240.462296651428));
#266012=CARTESIAN_POINT('Ctrl Pts',(-64.4501995169385,-113.443927583197,
238.462296651429));
#266013=CARTESIAN_POINT('Ctrl Pts',(-72.9267251261946,-107.704469842635,
236.462296651428));
#266014=CARTESIAN_POINT('Ctrl Pts',(-81.4032507354507,-101.965012102074,
234.462296651428));
#266015=CARTESIAN_POINT('Ctrl Pts',(-88.8775672472032,-94.9701958612992,
232.462296651428));
#266016=CARTESIAN_POINT('Ctrl Pts',(-96.3518837589557,-87.9753796205246,
230.462296651428));
#266017=CARTESIAN_POINT('Ctrl Pts',(-102.639948694851,-79.8974404698484,
228.462296651428));
#266018=CARTESIAN_POINT('Ctrl Pts',(-108.928013630747,-71.8195013191723,
226.462296651428));
#266019=CARTESIAN_POINT('Ctrl Pts',(-113.874993963172,-62.8573449296276,
224.462296651428));
#266020=CARTESIAN_POINT('Ctrl Pts',(-118.821974295598,-53.8951885400829,
222.462296651428));
#266021=CARTESIAN_POINT('Ctrl Pts',(-122.306058950682,-44.2694929456718,
220.462296651428));
#266022=CARTESIAN_POINT('Ctrl Pts',(-125.790143605767,-34.6437973512606,
218.462296651428));
#266023=CARTESIAN_POINT('Ctrl Pts',(-127.725542856289,-24.5915791233698,
216.462296651428));
#266024=CARTESIAN_POINT('Ctrl Pts',(-129.660942106811,-14.5393608954789,
214.462296651428));
#266025=CARTESIAN_POINT('Ctrl Pts',(-130.,-4.30813900827845,212.462296651428));
#266026=CARTESIAN_POINT('',(-118.376086385729,53.9041949546877,367.5));
#266027=CARTESIAN_POINT('',(-128.373075022505,20.9502666088252,367.5));
#266028=CARTESIAN_POINT('Ctrl Pts',(-118.376086385729,53.9041949546877,
367.5));
#266029=CARTESIAN_POINT('Ctrl Pts',(-119.546342407814,51.276867586874,367.5));
#266030=CARTESIAN_POINT('Ctrl Pts',(-120.634616850713,48.6137313363238,
367.499999999997));
#266031=CARTESIAN_POINT('Ctrl Pts',(-122.645087654721,43.2205933565672,
367.499999999997));
#266032=CARTESIAN_POINT('Ctrl Pts',(-123.566638088337,40.491727202324,367.5));
#266033=CARTESIAN_POINT('Ctrl Pts',(-126.073121396906,32.2286687868899,
367.5));
#266034=CARTESIAN_POINT('Ctrl Pts',(-127.399213018598,26.6223327935032,
367.5));
#266035=CARTESIAN_POINT('Ctrl Pts',(-128.373075022505,20.9502666088252,
367.5));
#266036=CARTESIAN_POINT('',(-130.,4.30813900827773,377.537703348572));
#266037=CARTESIAN_POINT('Ctrl Pts',(-130.,4.30813900827773,377.537703348572));
#266038=CARTESIAN_POINT('Ctrl Pts',(-129.660942106811,14.5393608954781,
375.537703348572));
#266039=CARTESIAN_POINT('Ctrl Pts',(-127.725542856289,24.591579123369,373.537703348572));
#266040=CARTESIAN_POINT('Ctrl Pts',(-125.790143605767,34.6437973512599,
371.537703348572));
#266041=CARTESIAN_POINT('Ctrl Pts',(-122.306058950683,44.269492945671,369.537703348572));
#266042=CARTESIAN_POINT('Ctrl Pts',(-120.533915146556,49.1655039490626,
368.520423931127));
#266043=CARTESIAN_POINT('Ctrl Pts',(-118.376086385729,53.9041949546877,
367.5));
#266044=CARTESIAN_POINT('',(-130.,-4.30813900827845,372.462296651428));
#266045=CARTESIAN_POINT('',(-130.,-3.57353036051222E-13,375.));
#266046=CARTESIAN_POINT('Ctrl Pts',(-130.,-4.30813900827845,372.462296651428));
#266047=CARTESIAN_POINT('Ctrl Pts',(-130.339057893189,5.92308287892196,
370.462296651428));
#266048=CARTESIAN_POINT('Ctrl Pts',(-129.073425698447,16.0813817870903,
368.462296651429));
#266049=CARTESIAN_POINT('Ctrl Pts',(-128.769291070567,18.5224467909361,
367.981691576521));
#266050=CARTESIAN_POINT('Ctrl Pts',(-128.373075022505,20.9502666088252,
367.5));
#266051=CARTESIAN_POINT('Ctrl Pts',(-160.,4.30813900827767,377.537703348572));
#266052=CARTESIAN_POINT('Ctrl Pts',(-159.660942106811,16.9004121002166,
375.537703348572));
#266053=CARTESIAN_POINT('Ctrl Pts',(-157.356193074143,29.2846130745759,
373.537703348572));
#266054=CARTESIAN_POINT('Ctrl Pts',(-155.051444041476,41.6688140489352,
371.537703348572));
#266055=CARTESIAN_POINT('Ctrl Pts',(-150.837754439537,53.5400027769194,
369.537703348572));
#266056=CARTESIAN_POINT('Ctrl Pts',(-146.624064837599,65.4111915049037,
367.537703348572));
#266057=CARTESIAN_POINT('Ctrl Pts',(-140.605189688823,76.4770599218133,
365.537703348572));
#266058=CARTESIAN_POINT('Ctrl Pts',(-134.586314540048,87.542928338723,363.537703348572));
#266059=CARTESIAN_POINT('Ctrl Pts',(-126.9104585261,97.530998038622,361.537703348572));
#266060=CARTESIAN_POINT('Ctrl Pts',(-119.234602512152,107.519067738521,
359.537703348572));
#266061=CARTESIAN_POINT('Ctrl Pts',(-110.0907706828,116.183399296895,357.537703348572));
#266062=CARTESIAN_POINT('Ctrl Pts',(-100.946938853448,124.847730855269,
355.537703348572));
#266063=CARTESIAN_POINT('Ctrl Pts',(-90.5602826949695,131.974979673883,
353.537703348572));
#266064=CARTESIAN_POINT('Ctrl Pts',(-80.1736265364906,139.102228492497,
351.537703348572));
#266065=CARTESIAN_POINT('Ctrl Pts',(-68.7998999948417,144.516898051454,
349.537703348572));
#266066=CARTESIAN_POINT('Ctrl Pts',(-57.4261734531929,149.931567610411,
347.537703348572));
#266067=CARTESIAN_POINT('Ctrl Pts',(-45.3454354230638,153.500330774912,
345.537703348572));
#266068=CARTESIAN_POINT('Ctrl Pts',(-33.2646973929347,157.069093939413,
343.537703348572));
#266069=CARTESIAN_POINT('Ctrl Pts',(-20.774415738298,158.704075916301,341.537703348572));
#266070=CARTESIAN_POINT('Ctrl Pts',(-8.28413408366129,160.339057893189,
339.537703348572));
#266071=CARTESIAN_POINT('Ctrl Pts',(4.30813900827766,160.,337.537703348572));
#266072=CARTESIAN_POINT('Ctrl Pts',(16.9004121002166,159.660942106811,335.537703348572));
#266073=CARTESIAN_POINT('Ctrl Pts',(29.2846130745759,157.356193074143,333.537703348572));
#266074=CARTESIAN_POINT('Ctrl Pts',(41.6688140489352,155.051444041476,331.537703348572));
#266075=CARTESIAN_POINT('Ctrl Pts',(53.5400027769194,150.837754439537,329.537703348572));
#266076=CARTESIAN_POINT('Ctrl Pts',(65.4111915049037,146.624064837599,327.537703348572));
#266077=CARTESIAN_POINT('Ctrl Pts',(76.4770599218133,140.605189688823,325.537703348572));
#266078=CARTESIAN_POINT('Ctrl Pts',(87.542928338723,134.586314540048,323.537703348572));
#266079=CARTESIAN_POINT('Ctrl Pts',(97.530998038622,126.9104585261,321.537703348572));
#266080=CARTESIAN_POINT('Ctrl Pts',(107.519067738521,119.234602512152,319.537703348572));
#266081=CARTESIAN_POINT('Ctrl Pts',(116.183399296895,110.0907706828,317.537703348572));
#266082=CARTESIAN_POINT('Ctrl Pts',(124.847730855269,100.946938853448,315.537703348572));
#266083=CARTESIAN_POINT('Ctrl Pts',(131.974979673883,90.5602826949695,313.537703348572));
#266084=CARTESIAN_POINT('Ctrl Pts',(139.102228492497,80.1736265364906,311.537703348572));
#266085=CARTESIAN_POINT('Ctrl Pts',(144.516898051454,68.7998999948417,309.537703348572));
#266086=CARTESIAN_POINT('Ctrl Pts',(149.931567610411,57.4261734531929,307.537703348572));
#266087=CARTESIAN_POINT('Ctrl Pts',(153.500330774912,45.3454354230638,305.537703348572));
#266088=CARTESIAN_POINT('Ctrl Pts',(157.069093939413,33.2646973929347,303.537703348572));
#266089=CARTESIAN_POINT('Ctrl Pts',(158.704075916301,20.774415738298,301.537703348572));
#266090=CARTESIAN_POINT('Ctrl Pts',(160.339057893189,8.28413408366131,299.537703348572));
#266091=CARTESIAN_POINT('Ctrl Pts',(160.,-4.30813900827765,297.537703348572));
#266092=CARTESIAN_POINT('Ctrl Pts',(159.660942106811,-16.9004121002166,
295.537703348572));
#266093=CARTESIAN_POINT('Ctrl Pts',(157.356193074143,-29.2846130745759,
293.537703348572));
#266094=CARTESIAN_POINT('Ctrl Pts',(155.051444041476,-41.6688140489352,
291.537703348572));
#266095=CARTESIAN_POINT('Ctrl Pts',(150.837754439537,-53.5400027769194,
289.537703348572));
#266096=CARTESIAN_POINT('Ctrl Pts',(146.624064837599,-65.4111915049036,
287.537703348572));
#266097=CARTESIAN_POINT('Ctrl Pts',(140.605189688823,-76.4770599218133,
285.537703348572));
#266098=CARTESIAN_POINT('Ctrl Pts',(134.586314540048,-87.5429283387229,
283.537703348572));
#266099=CARTESIAN_POINT('Ctrl Pts',(126.9104585261,-97.530998038622,281.537703348572));
#266100=CARTESIAN_POINT('Ctrl Pts',(119.234602512152,-107.519067738521,
279.537703348572));
#266101=CARTESIAN_POINT('Ctrl Pts',(110.0907706828,-116.183399296895,277.537703348572));
#266102=CARTESIAN_POINT('Ctrl Pts',(100.946938853448,-124.847730855269,
275.537703348572));
#266103=CARTESIAN_POINT('Ctrl Pts',(90.5602826949695,-131.974979673883,
273.537703348572));
#266104=CARTESIAN_POINT('Ctrl Pts',(80.1736265364905,-139.102228492497,
271.537703348572));
#266105=CARTESIAN_POINT('Ctrl Pts',(68.7998999948417,-144.516898051454,
269.537703348572));
#266106=CARTESIAN_POINT('Ctrl Pts',(57.426173453193,-149.931567610411,267.537703348572));
#266107=CARTESIAN_POINT('Ctrl Pts',(45.3454354230638,-153.500330774912,
265.537703348572));
#266108=CARTESIAN_POINT('Ctrl Pts',(33.2646973929347,-157.069093939413,
263.537703348572));
#266109=CARTESIAN_POINT('Ctrl Pts',(20.774415738298,-158.704075916301,261.537703348572));
#266110=CARTESIAN_POINT('Ctrl Pts',(8.28413408366139,-160.339057893189,
259.537703348572));
#266111=CARTESIAN_POINT('Ctrl Pts',(-4.30813900827764,-160.,257.537703348572));
#266112=CARTESIAN_POINT('Ctrl Pts',(-16.9004121002167,-159.660942106811,
255.537703348572));
#266113=CARTESIAN_POINT('Ctrl Pts',(-29.2846130745759,-157.356193074143,
253.537703348572));
#266114=CARTESIAN_POINT('Ctrl Pts',(-41.6688140489351,-155.051444041476,
251.537703348572));
#266115=CARTESIAN_POINT('Ctrl Pts',(-53.5400027769194,-150.837754439537,
249.537703348572));
#266116=CARTESIAN_POINT('Ctrl Pts',(-65.4111915049037,-146.624064837599,
247.537703348572));
#266117=CARTESIAN_POINT('Ctrl Pts',(-76.4770599218133,-140.605189688823,
245.537703348572));
#266118=CARTESIAN_POINT('Ctrl Pts',(-87.5429283387229,-134.586314540048,
243.537703348572));
#266119=CARTESIAN_POINT('Ctrl Pts',(-97.530998038622,-126.9104585261,241.537703348572));
#266120=CARTESIAN_POINT('Ctrl Pts',(-107.519067738521,-119.234602512152,
239.537703348572));
#266121=CARTESIAN_POINT('Ctrl Pts',(-116.183399296895,-110.0907706828,237.537703348572));
#266122=CARTESIAN_POINT('Ctrl Pts',(-124.847730855269,-100.946938853448,
235.537703348572));
#266123=CARTESIAN_POINT('Ctrl Pts',(-131.974979673883,-90.5602826949695,
233.537703348572));
#266124=CARTESIAN_POINT('Ctrl Pts',(-139.102228492497,-80.1736265364905,
231.537703348572));
#266125=CARTESIAN_POINT('Ctrl Pts',(-144.516898051454,-68.7998999948417,
229.537703348572));
#266126=CARTESIAN_POINT('Ctrl Pts',(-149.931567610411,-57.426173453193,
227.537703348572));
#266127=CARTESIAN_POINT('Ctrl Pts',(-153.500330774912,-45.3454354230638,
225.537703348572));
#266128=CARTESIAN_POINT('Ctrl Pts',(-157.069093939413,-33.2646973929347,
223.537703348572));
#266129=CARTESIAN_POINT('Ctrl Pts',(-158.704075916301,-20.774415738298,
221.537703348572));
#266130=CARTESIAN_POINT('Ctrl Pts',(-160.339057893189,-8.2841340836614,
219.537703348572));
#266131=CARTESIAN_POINT('Ctrl Pts',(-160.,4.30813900827767,217.537703348572));
#266132=CARTESIAN_POINT('Ctrl Pts',(-130.,4.30813900827773,377.537703348572));
#266133=CARTESIAN_POINT('Ctrl Pts',(-129.660942106811,14.5393608954781,
375.537703348572));
#266134=CARTESIAN_POINT('Ctrl Pts',(-127.725542856289,24.591579123369,373.537703348572));
#266135=CARTESIAN_POINT('Ctrl Pts',(-125.790143605767,34.6437973512599,
371.537703348572));
#266136=CARTESIAN_POINT('Ctrl Pts',(-122.306058950683,44.269492945671,369.537703348572));
#266137=CARTESIAN_POINT('Ctrl Pts',(-118.821974295598,53.8951885400822,
367.537703348572));
#266138=CARTESIAN_POINT('Ctrl Pts',(-113.874993963172,62.8573449296269,
365.537703348572));
#266139=CARTESIAN_POINT('Ctrl Pts',(-108.928013630747,71.8195013191717,
363.537703348572));
#266140=CARTESIAN_POINT('Ctrl Pts',(-102.639948694852,79.8974404698478,
361.537703348572));
#266141=CARTESIAN_POINT('Ctrl Pts',(-96.3518837589562,87.9753796205239,
359.537703348572));
#266142=CARTESIAN_POINT('Ctrl Pts',(-88.8775672472037,94.9701958612987,
357.537703348572));
#266143=CARTESIAN_POINT('Ctrl Pts',(-81.4032507354512,101.965012102073,
355.537703348572));
#266144=CARTESIAN_POINT('Ctrl Pts',(-72.9267251261952,107.704469842635,
353.537703348572));
#266145=CARTESIAN_POINT('Ctrl Pts',(-64.4501995169392,113.443927583196,
351.537703348572));
#266146=CARTESIAN_POINT('Ctrl Pts',(-55.1801850026552,117.786702325803,
349.537703348572));
#266147=CARTESIAN_POINT('Ctrl Pts',(-45.9101704883713,122.12947706841,347.537703348572));
#266148=CARTESIAN_POINT('Ctrl Pts',(-36.0749255918153,124.968635286057,
345.537703348572));
#266149=CARTESIAN_POINT('Ctrl Pts',(-26.2396806952593,127.807793503704,
343.537703348572));
#266150=CARTESIAN_POINT('Ctrl Pts',(-16.081381787091,129.073425698447,341.537703348572));
#266151=CARTESIAN_POINT('Ctrl Pts',(-5.92308287892268,130.339057893189,
339.537703348572));
#266152=CARTESIAN_POINT('Ctrl Pts',(4.30813900827772,130.,337.537703348572));
#266153=CARTESIAN_POINT('Ctrl Pts',(14.5393608954781,129.660942106811,335.537703348572));
#266154=CARTESIAN_POINT('Ctrl Pts',(24.591579123369,127.725542856289,333.537703348572));
#266155=CARTESIAN_POINT('Ctrl Pts',(34.6437973512599,125.790143605767,331.537703348572));
#266156=CARTESIAN_POINT('Ctrl Pts',(44.269492945671,122.306058950683,329.537703348572));
#266157=CARTESIAN_POINT('Ctrl Pts',(53.8951885400822,118.821974295598,327.537703348572));
#266158=CARTESIAN_POINT('Ctrl Pts',(62.8573449296269,113.874993963172,325.537703348572));
#266159=CARTESIAN_POINT('Ctrl Pts',(71.8195013191717,108.928013630747,323.537703348572));
#266160=CARTESIAN_POINT('Ctrl Pts',(79.8974404698478,102.639948694852,321.537703348572));
#266161=CARTESIAN_POINT('Ctrl Pts',(87.9753796205239,96.3518837589562,319.537703348572));
#266162=CARTESIAN_POINT('Ctrl Pts',(94.9701958612986,88.8775672472037,317.537703348572));
#266163=CARTESIAN_POINT('Ctrl Pts',(101.965012102073,81.4032507354512,315.537703348572));
#266164=CARTESIAN_POINT('Ctrl Pts',(107.704469842635,72.9267251261952,313.537703348572));
#266165=CARTESIAN_POINT('Ctrl Pts',(113.443927583196,64.4501995169392,311.537703348572));
#266166=CARTESIAN_POINT('Ctrl Pts',(117.786702325803,55.1801850026552,309.537703348572));
#266167=CARTESIAN_POINT('Ctrl Pts',(122.12947706841,45.9101704883713,307.537703348572));
#266168=CARTESIAN_POINT('Ctrl Pts',(124.968635286057,36.0749255918153,305.537703348572));
#266169=CARTESIAN_POINT('Ctrl Pts',(127.807793503704,26.2396806952593,303.537703348572));
#266170=CARTESIAN_POINT('Ctrl Pts',(129.073425698447,16.081381787091,301.537703348572));
#266171=CARTESIAN_POINT('Ctrl Pts',(130.339057893189,5.92308287892268,299.537703348572));
#266172=CARTESIAN_POINT('Ctrl Pts',(130.,-4.30813900827772,297.537703348572));
#266173=CARTESIAN_POINT('Ctrl Pts',(129.660942106811,-14.5393608954781,
295.537703348572));
#266174=CARTESIAN_POINT('Ctrl Pts',(127.725542856289,-24.591579123369,293.537703348572));
#266175=CARTESIAN_POINT('Ctrl Pts',(125.790143605767,-34.6437973512599,
291.537703348572));
#266176=CARTESIAN_POINT('Ctrl Pts',(122.306058950683,-44.269492945671,289.537703348572));
#266177=CARTESIAN_POINT('Ctrl Pts',(118.821974295598,-53.8951885400822,
287.537703348572));
#266178=CARTESIAN_POINT('Ctrl Pts',(113.874993963172,-62.8573449296269,
285.537703348572));
#266179=CARTESIAN_POINT('Ctrl Pts',(108.928013630747,-71.8195013191717,
283.537703348572));
#266180=CARTESIAN_POINT('Ctrl Pts',(102.639948694852,-79.8974404698478,
281.537703348572));
#266181=CARTESIAN_POINT('Ctrl Pts',(96.3518837589563,-87.9753796205239,
279.537703348572));
#266182=CARTESIAN_POINT('Ctrl Pts',(88.8775672472037,-94.9701958612986,
277.537703348572));
#266183=CARTESIAN_POINT('Ctrl Pts',(81.4032507354513,-101.965012102073,
275.537703348572));
#266184=CARTESIAN_POINT('Ctrl Pts',(72.9267251261952,-107.704469842635,
273.537703348572));
#266185=CARTESIAN_POINT('Ctrl Pts',(64.4501995169392,-113.443927583196,
271.537703348572));
#266186=CARTESIAN_POINT('Ctrl Pts',(55.1801850026552,-117.786702325803,
269.537703348572));
#266187=CARTESIAN_POINT('Ctrl Pts',(45.9101704883713,-122.12947706841,267.537703348572));
#266188=CARTESIAN_POINT('Ctrl Pts',(36.0749255918153,-124.968635286057,
265.537703348572));
#266189=CARTESIAN_POINT('Ctrl Pts',(26.2396806952593,-127.807793503704,
263.537703348572));
#266190=CARTESIAN_POINT('Ctrl Pts',(16.081381787091,-129.073425698447,261.537703348572));
#266191=CARTESIAN_POINT('Ctrl Pts',(5.92308287892275,-130.339057893189,
259.537703348572));
#266192=CARTESIAN_POINT('Ctrl Pts',(-4.30813900827771,-130.,257.537703348572));
#266193=CARTESIAN_POINT('Ctrl Pts',(-14.5393608954782,-129.660942106811,
255.537703348572));
#266194=CARTESIAN_POINT('Ctrl Pts',(-24.591579123369,-127.725542856289,
253.537703348572));
#266195=CARTESIAN_POINT('Ctrl Pts',(-34.6437973512598,-125.790143605767,
251.537703348572));
#266196=CARTESIAN_POINT('Ctrl Pts',(-44.269492945671,-122.306058950683,
249.537703348572));
#266197=CARTESIAN_POINT('Ctrl Pts',(-53.8951885400822,-118.821974295598,
247.537703348572));
#266198=CARTESIAN_POINT('Ctrl Pts',(-62.8573449296269,-113.874993963172,
245.537703348572));
#266199=CARTESIAN_POINT('Ctrl Pts',(-71.8195013191717,-108.928013630747,
243.537703348572));
#266200=CARTESIAN_POINT('Ctrl Pts',(-79.8974404698478,-102.639948694852,
241.537703348572));
#266201=CARTESIAN_POINT('Ctrl Pts',(-87.975379620524,-96.3518837589562,
239.537703348572));
#266202=CARTESIAN_POINT('Ctrl Pts',(-94.9701958612986,-88.8775672472037,
237.537703348572));
#266203=CARTESIAN_POINT('Ctrl Pts',(-101.965012102073,-81.4032507354513,
235.537703348572));
#266204=CARTESIAN_POINT('Ctrl Pts',(-107.704469842635,-72.9267251261952,
233.537703348572));
#266205=CARTESIAN_POINT('Ctrl Pts',(-113.443927583196,-64.4501995169392,
231.537703348572));
#266206=CARTESIAN_POINT('Ctrl Pts',(-117.786702325803,-55.1801850026553,
229.537703348572));
#266207=CARTESIAN_POINT('Ctrl Pts',(-122.12947706841,-45.9101704883713,
227.537703348572));
#266208=CARTESIAN_POINT('Ctrl Pts',(-124.968635286057,-36.0749255918153,
225.537703348572));
#266209=CARTESIAN_POINT('Ctrl Pts',(-127.807793503704,-26.2396806952593,
223.537703348572));
#266210=CARTESIAN_POINT('Ctrl Pts',(-129.073425698447,-16.081381787091,
221.537703348572));
#266211=CARTESIAN_POINT('Ctrl Pts',(-130.339057893189,-5.92308287892275,
219.537703348572));
#266212=CARTESIAN_POINT('Ctrl Pts',(-130.,4.30813900827773,217.537703348572));
#266213=CARTESIAN_POINT('',(-146.075461400193,65.4256802672723,367.5));
#266214=CARTESIAN_POINT('',(-146.075461400193,65.4256802672722,367.5));
#266215=CARTESIAN_POINT('',(-160.,4.30813900827767,377.537703348572));
#266216=CARTESIAN_POINT('Ctrl Pts',(-160.,4.30813900827767,377.537703348572));
#266217=CARTESIAN_POINT('Ctrl Pts',(-159.660942106811,16.9004121002166,
375.537703348572));
#266218=CARTESIAN_POINT('Ctrl Pts',(-157.356193074143,29.2846130745759,
373.537703348572));
#266219=CARTESIAN_POINT('Ctrl Pts',(-155.051444041476,41.6688140489352,
371.537703348572));
#266220=CARTESIAN_POINT('Ctrl Pts',(-150.837754439537,53.5400027769194,
369.537703348572));
#266221=CARTESIAN_POINT('Ctrl Pts',(-148.694504587761,59.5781607537101,
368.520423931127));
#266222=CARTESIAN_POINT('Ctrl Pts',(-146.075461400193,65.4256802672722,
367.5));
#266223=CARTESIAN_POINT('',(-145.,4.3081390082777,377.537703348572));
#266224=CARTESIAN_POINT('Ctrl Pts',(-160.,-4.30813900827851,372.462296651429));
#266225=CARTESIAN_POINT('Ctrl Pts',(-160.339057893189,8.28413408366045,
370.462296651429));
#266226=CARTESIAN_POINT('Ctrl Pts',(-158.704075916301,20.7744157382972,
368.462296651429));
#266227=CARTESIAN_POINT('Ctrl Pts',(-157.069093939413,33.2646973929339,
366.462296651429));
#266228=CARTESIAN_POINT('Ctrl Pts',(-153.500330774912,45.345435423063,364.462296651429));
#266229=CARTESIAN_POINT('Ctrl Pts',(-149.931567610412,57.4261734531921,
362.462296651429));
#266230=CARTESIAN_POINT('Ctrl Pts',(-144.516898051455,68.7998999948409,
360.462296651429));
#266231=CARTESIAN_POINT('Ctrl Pts',(-139.102228492498,80.1736265364898,
358.462296651429));
#266232=CARTESIAN_POINT('Ctrl Pts',(-131.974979673884,90.5602826949688,
356.462296651429));
#266233=CARTESIAN_POINT('Ctrl Pts',(-124.84773085527,100.946938853448,354.462296651429));
#266234=CARTESIAN_POINT('Ctrl Pts',(-116.183399296896,110.0907706828,352.462296651429));
#266235=CARTESIAN_POINT('Ctrl Pts',(-107.519067738522,119.234602512151,
350.462296651429));
#266236=CARTESIAN_POINT('Ctrl Pts',(-97.5309980386227,126.9104585261,348.462296651429));
#266237=CARTESIAN_POINT('Ctrl Pts',(-87.5429283387237,134.586314540048,
346.462296651428));
#266238=CARTESIAN_POINT('Ctrl Pts',(-76.4770599218141,140.605189688823,
344.462296651429));
#266239=CARTESIAN_POINT('Ctrl Pts',(-65.4111915049045,146.624064837598,
342.462296651429));
#266240=CARTESIAN_POINT('Ctrl Pts',(-53.5400027769202,150.837754439537,
340.462296651429));
#266241=CARTESIAN_POINT('Ctrl Pts',(-41.668814048936,155.051444041475,338.462296651429));
#266242=CARTESIAN_POINT('Ctrl Pts',(-29.2846130745767,157.356193074143,
336.462296651429));
#266243=CARTESIAN_POINT('Ctrl Pts',(-16.9004121002175,159.660942106811,
334.462296651428));
#266244=CARTESIAN_POINT('Ctrl Pts',(-4.30813900827852,160.,332.462296651429));
#266245=CARTESIAN_POINT('Ctrl Pts',(8.28413408366043,160.339057893189,330.462296651429));
#266246=CARTESIAN_POINT('Ctrl Pts',(20.7744157382972,158.704075916301,328.462296651429));
#266247=CARTESIAN_POINT('Ctrl Pts',(33.2646973929339,157.069093939413,326.462296651428));
#266248=CARTESIAN_POINT('Ctrl Pts',(45.345435423063,153.500330774912,324.462296651429));
#266249=CARTESIAN_POINT('Ctrl Pts',(57.4261734531921,149.931567610412,322.462296651428));
#266250=CARTESIAN_POINT('Ctrl Pts',(68.7998999948409,144.516898051455,320.462296651429));
#266251=CARTESIAN_POINT('Ctrl Pts',(80.1736265364898,139.102228492498,318.462296651429));
#266252=CARTESIAN_POINT('Ctrl Pts',(90.5602826949688,131.974979673884,316.462296651429));
#266253=CARTESIAN_POINT('Ctrl Pts',(100.946938853448,124.84773085527,314.462296651429));
#266254=CARTESIAN_POINT('Ctrl Pts',(110.0907706828,116.183399296896,312.462296651429));
#266255=CARTESIAN_POINT('Ctrl Pts',(119.234602512151,107.519067738522,310.462296651429));
#266256=CARTESIAN_POINT('Ctrl Pts',(126.9104585261,97.5309980386227,308.462296651429));
#266257=CARTESIAN_POINT('Ctrl Pts',(134.586314540048,87.5429283387237,306.462296651429));
#266258=CARTESIAN_POINT('Ctrl Pts',(140.605189688823,76.4770599218141,304.462296651429));
#266259=CARTESIAN_POINT('Ctrl Pts',(146.624064837598,65.4111915049045,302.462296651429));
#266260=CARTESIAN_POINT('Ctrl Pts',(150.837754439537,53.5400027769202,300.462296651429));
#266261=CARTESIAN_POINT('Ctrl Pts',(155.051444041475,41.668814048936,298.462296651429));
#266262=CARTESIAN_POINT('Ctrl Pts',(157.356193074143,29.2846130745767,296.462296651429));
#266263=CARTESIAN_POINT('Ctrl Pts',(159.660942106811,16.9004121002175,294.462296651429));
#266264=CARTESIAN_POINT('Ctrl Pts',(160.,4.30813900827853,292.462296651429));
#266265=CARTESIAN_POINT('Ctrl Pts',(160.339057893189,-8.28413408366043,
290.462296651429));
#266266=CARTESIAN_POINT('Ctrl Pts',(158.704075916301,-20.7744157382971,
288.462296651429));
#266267=CARTESIAN_POINT('Ctrl Pts',(157.069093939413,-33.2646973929339,
286.462296651429));
#266268=CARTESIAN_POINT('Ctrl Pts',(153.500330774912,-45.345435423063,284.462296651429));
#266269=CARTESIAN_POINT('Ctrl Pts',(149.931567610412,-57.4261734531921,
282.462296651429));
#266270=CARTESIAN_POINT('Ctrl Pts',(144.516898051455,-68.7998999948409,
280.462296651429));
#266271=CARTESIAN_POINT('Ctrl Pts',(139.102228492498,-80.1736265364898,
278.462296651429));
#266272=CARTESIAN_POINT('Ctrl Pts',(131.974979673884,-90.5602826949688,
276.462296651429));
#266273=CARTESIAN_POINT('Ctrl Pts',(124.84773085527,-100.946938853448,274.462296651429));
#266274=CARTESIAN_POINT('Ctrl Pts',(116.183399296896,-110.0907706828,272.462296651429));
#266275=CARTESIAN_POINT('Ctrl Pts',(107.519067738522,-119.234602512151,
270.462296651429));
#266276=CARTESIAN_POINT('Ctrl Pts',(97.5309980386227,-126.9104585261,268.462296651429));
#266277=CARTESIAN_POINT('Ctrl Pts',(87.5429283387236,-134.586314540048,
266.462296651429));
#266278=CARTESIAN_POINT('Ctrl Pts',(76.4770599218141,-140.605189688823,
264.462296651429));
#266279=CARTESIAN_POINT('Ctrl Pts',(65.4111915049046,-146.624064837598,
262.462296651429));
#266280=CARTESIAN_POINT('Ctrl Pts',(53.5400027769202,-150.837754439537,
260.462296651429));
#266281=CARTESIAN_POINT('Ctrl Pts',(41.6688140489359,-155.051444041475,
258.462296651429));
#266282=CARTESIAN_POINT('Ctrl Pts',(29.2846130745768,-157.356193074143,
256.462296651429));
#266283=CARTESIAN_POINT('Ctrl Pts',(16.9004121002176,-159.660942106811,
254.462296651429));
#266284=CARTESIAN_POINT('Ctrl Pts',(4.30813900827854,-160.,252.462296651429));
#266285=CARTESIAN_POINT('Ctrl Pts',(-8.28413408366049,-160.339057893189,
250.462296651429));
#266286=CARTESIAN_POINT('Ctrl Pts',(-20.7744157382971,-158.704075916301,
248.462296651429));
#266287=CARTESIAN_POINT('Ctrl Pts',(-33.2646973929338,-157.069093939413,
246.462296651429));
#266288=CARTESIAN_POINT('Ctrl Pts',(-45.345435423063,-153.500330774912,
244.462296651429));
#266289=CARTESIAN_POINT('Ctrl Pts',(-57.4261734531921,-149.931567610412,
242.462296651429));
#266290=CARTESIAN_POINT('Ctrl Pts',(-68.7998999948409,-144.516898051455,
240.462296651429));
#266291=CARTESIAN_POINT('Ctrl Pts',(-80.1736265364897,-139.102228492498,
238.462296651429));
#266292=CARTESIAN_POINT('Ctrl Pts',(-90.5602826949688,-131.974979673884,
236.462296651429));
#266293=CARTESIAN_POINT('Ctrl Pts',(-100.946938853448,-124.84773085527,
234.462296651429));
#266294=CARTESIAN_POINT('Ctrl Pts',(-110.0907706828,-116.183399296896,232.462296651429));
#266295=CARTESIAN_POINT('Ctrl Pts',(-119.234602512151,-107.519067738522,
230.462296651429));
#266296=CARTESIAN_POINT('Ctrl Pts',(-126.9104585261,-97.5309980386227,228.462296651429));
#266297=CARTESIAN_POINT('Ctrl Pts',(-134.586314540048,-87.5429283387236,
226.462296651429));
#266298=CARTESIAN_POINT('Ctrl Pts',(-140.605189688823,-76.4770599218141,
224.462296651429));
#266299=CARTESIAN_POINT('Ctrl Pts',(-146.624064837598,-65.4111915049046,
222.462296651429));
#266300=CARTESIAN_POINT('Ctrl Pts',(-150.837754439537,-53.5400027769203,
220.462296651429));
#266301=CARTESIAN_POINT('Ctrl Pts',(-155.051444041475,-41.668814048936,
218.462296651429));
#266302=CARTESIAN_POINT('Ctrl Pts',(-157.356193074143,-29.2846130745768,
216.462296651429));
#266303=CARTESIAN_POINT('Ctrl Pts',(-159.660942106811,-16.9004121002176,
214.462296651429));
#266304=CARTESIAN_POINT('Ctrl Pts',(-160.,-4.30813900827851,212.462296651429));
#266305=CARTESIAN_POINT('Ctrl Pts',(-160.,4.30813900827767,377.537703348572));
#266306=CARTESIAN_POINT('Ctrl Pts',(-159.660942106811,16.9004121002166,
375.537703348572));
#266307=CARTESIAN_POINT('Ctrl Pts',(-157.356193074143,29.2846130745759,
373.537703348572));
#266308=CARTESIAN_POINT('Ctrl Pts',(-155.051444041476,41.6688140489352,
371.537703348572));
#266309=CARTESIAN_POINT('Ctrl Pts',(-150.837754439537,53.5400027769194,
369.537703348572));
#266310=CARTESIAN_POINT('Ctrl Pts',(-146.624064837599,65.4111915049037,
367.537703348572));
#266311=CARTESIAN_POINT('Ctrl Pts',(-140.605189688823,76.4770599218133,
365.537703348572));
#266312=CARTESIAN_POINT('Ctrl Pts',(-134.586314540048,87.542928338723,363.537703348572));
#266313=CARTESIAN_POINT('Ctrl Pts',(-126.9104585261,97.530998038622,361.537703348572));
#266314=CARTESIAN_POINT('Ctrl Pts',(-119.234602512152,107.519067738521,
359.537703348572));
#266315=CARTESIAN_POINT('Ctrl Pts',(-110.0907706828,116.183399296895,357.537703348572));
#266316=CARTESIAN_POINT('Ctrl Pts',(-100.946938853448,124.847730855269,
355.537703348572));
#266317=CARTESIAN_POINT('Ctrl Pts',(-90.5602826949695,131.974979673883,
353.537703348572));
#266318=CARTESIAN_POINT('Ctrl Pts',(-80.1736265364906,139.102228492497,
351.537703348572));
#266319=CARTESIAN_POINT('Ctrl Pts',(-68.7998999948417,144.516898051454,
349.537703348572));
#266320=CARTESIAN_POINT('Ctrl Pts',(-57.4261734531929,149.931567610411,
347.537703348572));
#266321=CARTESIAN_POINT('Ctrl Pts',(-45.3454354230638,153.500330774912,
345.537703348572));
#266322=CARTESIAN_POINT('Ctrl Pts',(-33.2646973929347,157.069093939413,
343.537703348572));
#266323=CARTESIAN_POINT('Ctrl Pts',(-20.774415738298,158.704075916301,341.537703348572));
#266324=CARTESIAN_POINT('Ctrl Pts',(-8.28413408366129,160.339057893189,
339.537703348572));
#266325=CARTESIAN_POINT('Ctrl Pts',(4.30813900827766,160.,337.537703348572));
#266326=CARTESIAN_POINT('Ctrl Pts',(16.9004121002166,159.660942106811,335.537703348572));
#266327=CARTESIAN_POINT('Ctrl Pts',(29.2846130745759,157.356193074143,333.537703348572));
#266328=CARTESIAN_POINT('Ctrl Pts',(41.6688140489352,155.051444041476,331.537703348572));
#266329=CARTESIAN_POINT('Ctrl Pts',(53.5400027769194,150.837754439537,329.537703348572));
#266330=CARTESIAN_POINT('Ctrl Pts',(65.4111915049037,146.624064837599,327.537703348572));
#266331=CARTESIAN_POINT('Ctrl Pts',(76.4770599218133,140.605189688823,325.537703348572));
#266332=CARTESIAN_POINT('Ctrl Pts',(87.542928338723,134.586314540048,323.537703348572));
#266333=CARTESIAN_POINT('Ctrl Pts',(97.530998038622,126.9104585261,321.537703348572));
#266334=CARTESIAN_POINT('Ctrl Pts',(107.519067738521,119.234602512152,319.537703348572));
#266335=CARTESIAN_POINT('Ctrl Pts',(116.183399296895,110.0907706828,317.537703348572));
#266336=CARTESIAN_POINT('Ctrl Pts',(124.847730855269,100.946938853448,315.537703348572));
#266337=CARTESIAN_POINT('Ctrl Pts',(131.974979673883,90.5602826949695,313.537703348572));
#266338=CARTESIAN_POINT('Ctrl Pts',(139.102228492497,80.1736265364906,311.537703348572));
#266339=CARTESIAN_POINT('Ctrl Pts',(144.516898051454,68.7998999948417,309.537703348572));
#266340=CARTESIAN_POINT('Ctrl Pts',(149.931567610411,57.4261734531929,307.537703348572));
#266341=CARTESIAN_POINT('Ctrl Pts',(153.500330774912,45.3454354230638,305.537703348572));
#266342=CARTESIAN_POINT('Ctrl Pts',(157.069093939413,33.2646973929347,303.537703348572));
#266343=CARTESIAN_POINT('Ctrl Pts',(158.704075916301,20.774415738298,301.537703348572));
#266344=CARTESIAN_POINT('Ctrl Pts',(160.339057893189,8.28413408366131,299.537703348572));
#266345=CARTESIAN_POINT('Ctrl Pts',(160.,-4.30813900827765,297.537703348572));
#266346=CARTESIAN_POINT('Ctrl Pts',(159.660942106811,-16.9004121002166,
295.537703348572));
#266347=CARTESIAN_POINT('Ctrl Pts',(157.356193074143,-29.2846130745759,
293.537703348572));
#266348=CARTESIAN_POINT('Ctrl Pts',(155.051444041476,-41.6688140489352,
291.537703348572));
#266349=CARTESIAN_POINT('Ctrl Pts',(150.837754439537,-53.5400027769194,
289.537703348572));
#266350=CARTESIAN_POINT('Ctrl Pts',(146.624064837599,-65.4111915049036,
287.537703348572));
#266351=CARTESIAN_POINT('Ctrl Pts',(140.605189688823,-76.4770599218133,
285.537703348572));
#266352=CARTESIAN_POINT('Ctrl Pts',(134.586314540048,-87.5429283387229,
283.537703348572));
#266353=CARTESIAN_POINT('Ctrl Pts',(126.9104585261,-97.530998038622,281.537703348572));
#266354=CARTESIAN_POINT('Ctrl Pts',(119.234602512152,-107.519067738521,
279.537703348572));
#266355=CARTESIAN_POINT('Ctrl Pts',(110.0907706828,-116.183399296895,277.537703348572));
#266356=CARTESIAN_POINT('Ctrl Pts',(100.946938853448,-124.847730855269,
275.537703348572));
#266357=CARTESIAN_POINT('Ctrl Pts',(90.5602826949695,-131.974979673883,
273.537703348572));
#266358=CARTESIAN_POINT('Ctrl Pts',(80.1736265364905,-139.102228492497,
271.537703348572));
#266359=CARTESIAN_POINT('Ctrl Pts',(68.7998999948417,-144.516898051454,
269.537703348572));
#266360=CARTESIAN_POINT('Ctrl Pts',(57.426173453193,-149.931567610411,267.537703348572));
#266361=CARTESIAN_POINT('Ctrl Pts',(45.3454354230638,-153.500330774912,
265.537703348572));
#266362=CARTESIAN_POINT('Ctrl Pts',(33.2646973929347,-157.069093939413,
263.537703348572));
#266363=CARTESIAN_POINT('Ctrl Pts',(20.774415738298,-158.704075916301,261.537703348572));
#266364=CARTESIAN_POINT('Ctrl Pts',(8.28413408366139,-160.339057893189,
259.537703348572));
#266365=CARTESIAN_POINT('Ctrl Pts',(-4.30813900827764,-160.,257.537703348572));
#266366=CARTESIAN_POINT('Ctrl Pts',(-16.9004121002167,-159.660942106811,
255.537703348572));
#266367=CARTESIAN_POINT('Ctrl Pts',(-29.2846130745759,-157.356193074143,
253.537703348572));
#266368=CARTESIAN_POINT('Ctrl Pts',(-41.6688140489351,-155.051444041476,
251.537703348572));
#266369=CARTESIAN_POINT('Ctrl Pts',(-53.5400027769194,-150.837754439537,
249.537703348572));
#266370=CARTESIAN_POINT('Ctrl Pts',(-65.4111915049037,-146.624064837599,
247.537703348572));
#266371=CARTESIAN_POINT('Ctrl Pts',(-76.4770599218133,-140.605189688823,
245.537703348572));
#266372=CARTESIAN_POINT('Ctrl Pts',(-87.5429283387229,-134.586314540048,
243.537703348572));
#266373=CARTESIAN_POINT('Ctrl Pts',(-97.530998038622,-126.9104585261,241.537703348572));
#266374=CARTESIAN_POINT('Ctrl Pts',(-107.519067738521,-119.234602512152,
239.537703348572));
#266375=CARTESIAN_POINT('Ctrl Pts',(-116.183399296895,-110.0907706828,237.537703348572));
#266376=CARTESIAN_POINT('Ctrl Pts',(-124.847730855269,-100.946938853448,
235.537703348572));
#266377=CARTESIAN_POINT('Ctrl Pts',(-131.974979673883,-90.5602826949695,
233.537703348572));
#266378=CARTESIAN_POINT('Ctrl Pts',(-139.102228492497,-80.1736265364905,
231.537703348572));
#266379=CARTESIAN_POINT('Ctrl Pts',(-144.516898051454,-68.7998999948417,
229.537703348572));
#266380=CARTESIAN_POINT('Ctrl Pts',(-149.931567610411,-57.426173453193,
227.537703348572));
#266381=CARTESIAN_POINT('Ctrl Pts',(-153.500330774912,-45.3454354230638,
225.537703348572));
#266382=CARTESIAN_POINT('Ctrl Pts',(-157.069093939413,-33.2646973929347,
223.537703348572));
#266383=CARTESIAN_POINT('Ctrl Pts',(-158.704075916301,-20.774415738298,
221.537703348572));
#266384=CARTESIAN_POINT('Ctrl Pts',(-160.339057893189,-8.2841340836614,
219.537703348572));
#266385=CARTESIAN_POINT('Ctrl Pts',(-160.,4.30813900827767,217.537703348572));
#266386=CARTESIAN_POINT('',(-157.805088795962,26.7603066464745,367.5));
#266387=CARTESIAN_POINT('Ctrl Pts',(-157.805088795962,26.7603066464745,
367.5));
#266388=CARTESIAN_POINT('Ctrl Pts',(-156.638532817877,33.4083424416569,
367.5));
#266389=CARTESIAN_POINT('Ctrl Pts',(-155.071407572055,39.9802096740424,
367.5));
#266390=CARTESIAN_POINT('Ctrl Pts',(-152.131501324444,49.6731919343096,
367.5));
#266391=CARTESIAN_POINT('Ctrl Pts',(-151.053085052424,52.8765297093725,
367.499999999997));
#266392=CARTESIAN_POINT('Ctrl Pts',(-148.705612539595,59.2094688002817,
367.499999999997));
#266393=CARTESIAN_POINT('Ctrl Pts',(-147.437304082636,62.3378048444623,
367.5));
#266394=CARTESIAN_POINT('Ctrl Pts',(-146.075461400193,65.4256802672723,
367.5));
#266395=CARTESIAN_POINT('',(-160.,-4.30813900827851,372.462296651429));
#266396=CARTESIAN_POINT('Ctrl Pts',(-160.,-4.30813900827851,372.462296651429));
#266397=CARTESIAN_POINT('Ctrl Pts',(-160.339057893189,8.28413408366045,
370.462296651429));
#266398=CARTESIAN_POINT('Ctrl Pts',(-158.704075916301,20.7744157382972,
368.462296651429));
#266399=CARTESIAN_POINT('Ctrl Pts',(-158.311185598564,23.7758621134177,
367.981691576521));
#266400=CARTESIAN_POINT('Ctrl Pts',(-157.805088795962,26.7603066464745,
367.5));
#266401=CARTESIAN_POINT('',(-160.,-4.21537804662364E-13,375.));
#266402=CARTESIAN_POINT('Ctrl Pts',(-130.,-4.30813900827845,372.462296651428));
#266403=CARTESIAN_POINT('Ctrl Pts',(-130.339057893189,5.92308287892195,
370.462296651428));
#266404=CARTESIAN_POINT('Ctrl Pts',(-129.073425698447,16.0813817870903,
368.462296651429));
#266405=CARTESIAN_POINT('Ctrl Pts',(-127.807793503705,26.2396806952586,
366.462296651429));
#266406=CARTESIAN_POINT('Ctrl Pts',(-124.968635286058,36.0749255918146,
364.462296651428));
#266407=CARTESIAN_POINT('Ctrl Pts',(-122.129477068411,45.9101704883706,
362.462296651428));
#266408=CARTESIAN_POINT('Ctrl Pts',(-117.786702325804,55.1801850026546,
360.462296651428));
#266409=CARTESIAN_POINT('Ctrl Pts',(-113.443927583196,64.4501995169386,
358.462296651428));
#266410=CARTESIAN_POINT('Ctrl Pts',(-107.704469842635,72.9267251261946,
356.462296651428));
#266411=CARTESIAN_POINT('Ctrl Pts',(-101.965012102074,81.4032507354507,
354.462296651428));
#266412=CARTESIAN_POINT('Ctrl Pts',(-94.9701958612992,88.8775672472032,
352.462296651428));
#266413=CARTESIAN_POINT('Ctrl Pts',(-87.9753796205245,96.3518837589558,
350.462296651428));
#266414=CARTESIAN_POINT('Ctrl Pts',(-79.8974404698484,102.639948694851,
348.462296651428));
#266415=CARTESIAN_POINT('Ctrl Pts',(-71.8195013191724,108.928013630747,
346.462296651428));
#266416=CARTESIAN_POINT('Ctrl Pts',(-62.8573449296276,113.874993963172,
344.462296651428));
#266417=CARTESIAN_POINT('Ctrl Pts',(-53.8951885400828,118.821974295598,
342.462296651428));
#266418=CARTESIAN_POINT('Ctrl Pts',(-44.2694929456717,122.306058950682,
340.462296651428));
#266419=CARTESIAN_POINT('Ctrl Pts',(-34.6437973512606,125.790143605767,
338.462296651428));
#266420=CARTESIAN_POINT('Ctrl Pts',(-24.5915791233697,127.725542856289,
336.462296651428));
#266421=CARTESIAN_POINT('Ctrl Pts',(-14.5393608954789,129.660942106811,
334.462296651428));
#266422=CARTESIAN_POINT('Ctrl Pts',(-4.30813900827846,130.,332.462296651428));
#266423=CARTESIAN_POINT('Ctrl Pts',(5.92308287892194,130.339057893189,330.462296651429));
#266424=CARTESIAN_POINT('Ctrl Pts',(16.0813817870903,129.073425698447,328.462296651428));
#266425=CARTESIAN_POINT('Ctrl Pts',(26.2396806952586,127.807793503705,326.462296651428));
#266426=CARTESIAN_POINT('Ctrl Pts',(36.0749255918146,124.968635286058,324.462296651428));
#266427=CARTESIAN_POINT('Ctrl Pts',(45.9101704883706,122.129477068411,322.462296651428));
#266428=CARTESIAN_POINT('Ctrl Pts',(55.1801850026546,117.786702325804,320.462296651428));
#266429=CARTESIAN_POINT('Ctrl Pts',(64.4501995169386,113.443927583196,318.462296651428));
#266430=CARTESIAN_POINT('Ctrl Pts',(72.9267251261946,107.704469842635,316.462296651428));
#266431=CARTESIAN_POINT('Ctrl Pts',(81.4032507354506,101.965012102074,314.462296651428));
#266432=CARTESIAN_POINT('Ctrl Pts',(88.8775672472032,94.9701958612992,312.462296651428));
#266433=CARTESIAN_POINT('Ctrl Pts',(96.3518837589558,87.9753796205245,310.462296651428));
#266434=CARTESIAN_POINT('Ctrl Pts',(102.639948694851,79.8974404698484,308.462296651428));
#266435=CARTESIAN_POINT('Ctrl Pts',(108.928013630747,71.8195013191724,306.462296651428));
#266436=CARTESIAN_POINT('Ctrl Pts',(113.874993963172,62.8573449296276,304.462296651428));
#266437=CARTESIAN_POINT('Ctrl Pts',(118.821974295598,53.8951885400829,302.462296651428));
#266438=CARTESIAN_POINT('Ctrl Pts',(122.306058950682,44.2694929456717,300.462296651428));
#266439=CARTESIAN_POINT('Ctrl Pts',(125.790143605767,34.6437973512606,298.462296651428));
#266440=CARTESIAN_POINT('Ctrl Pts',(127.725542856289,24.5915791233698,296.462296651428));
#266441=CARTESIAN_POINT('Ctrl Pts',(129.660942106811,14.5393608954789,294.462296651429));
#266442=CARTESIAN_POINT('Ctrl Pts',(130.,4.30813900827846,292.462296651428));
#266443=CARTESIAN_POINT('Ctrl Pts',(130.339057893189,-5.92308287892194,
290.462296651428));
#266444=CARTESIAN_POINT('Ctrl Pts',(129.073425698447,-16.0813817870903,
288.462296651428));
#266445=CARTESIAN_POINT('Ctrl Pts',(127.807793503705,-26.2396806952586,
286.462296651428));
#266446=CARTESIAN_POINT('Ctrl Pts',(124.968635286058,-36.0749255918146,
284.462296651428));
#266447=CARTESIAN_POINT('Ctrl Pts',(122.129477068411,-45.9101704883706,
282.462296651428));
#266448=CARTESIAN_POINT('Ctrl Pts',(117.786702325804,-55.1801850026546,
280.462296651428));
#266449=CARTESIAN_POINT('Ctrl Pts',(113.443927583196,-64.4501995169386,
278.462296651428));
#266450=CARTESIAN_POINT('Ctrl Pts',(107.704469842635,-72.9267251261946,
276.462296651428));
#266451=CARTESIAN_POINT('Ctrl Pts',(101.965012102074,-81.4032507354506,
274.462296651428));
#266452=CARTESIAN_POINT('Ctrl Pts',(94.9701958612992,-88.8775672472032,
272.462296651428));
#266453=CARTESIAN_POINT('Ctrl Pts',(87.9753796205246,-96.3518837589557,
270.462296651428));
#266454=CARTESIAN_POINT('Ctrl Pts',(79.8974404698484,-102.639948694851,
268.462296651428));
#266455=CARTESIAN_POINT('Ctrl Pts',(71.8195013191723,-108.928013630747,
266.462296651428));
#266456=CARTESIAN_POINT('Ctrl Pts',(62.8573449296276,-113.874993963172,
264.462296651428));
#266457=CARTESIAN_POINT('Ctrl Pts',(53.8951885400829,-118.821974295598,
262.462296651428));
#266458=CARTESIAN_POINT('Ctrl Pts',(44.2694929456717,-122.306058950682,
260.462296651428));
#266459=CARTESIAN_POINT('Ctrl Pts',(34.6437973512606,-125.790143605767,
258.462296651428));
#266460=CARTESIAN_POINT('Ctrl Pts',(24.5915791233698,-127.725542856289,
256.462296651428));
#266461=CARTESIAN_POINT('Ctrl Pts',(14.5393608954789,-129.660942106811,
254.462296651428));
#266462=CARTESIAN_POINT('Ctrl Pts',(4.30813900827847,-130.,252.462296651428));
#266463=CARTESIAN_POINT('Ctrl Pts',(-5.92308287892199,-130.339057893189,
250.462296651428));
#266464=CARTESIAN_POINT('Ctrl Pts',(-16.0813817870903,-129.073425698447,
248.462296651428));
#266465=CARTESIAN_POINT('Ctrl Pts',(-26.2396806952585,-127.807793503705,
246.462296651428));
#266466=CARTESIAN_POINT('Ctrl Pts',(-36.0749255918146,-124.968635286058,
244.462296651428));
#266467=CARTESIAN_POINT('Ctrl Pts',(-45.9101704883706,-122.129477068411,
242.462296651428));
#266468=CARTESIAN_POINT('Ctrl Pts',(-55.1801850026546,-117.786702325804,
240.462296651428));
#266469=CARTESIAN_POINT('Ctrl Pts',(-64.4501995169385,-113.443927583197,
238.462296651429));
#266470=CARTESIAN_POINT('Ctrl Pts',(-72.9267251261946,-107.704469842635,
236.462296651428));
#266471=CARTESIAN_POINT('Ctrl Pts',(-81.4032507354507,-101.965012102074,
234.462296651428));
#266472=CARTESIAN_POINT('Ctrl Pts',(-88.8775672472032,-94.9701958612992,
232.462296651428));
#266473=CARTESIAN_POINT('Ctrl Pts',(-96.3518837589557,-87.9753796205246,
230.462296651428));
#266474=CARTESIAN_POINT('Ctrl Pts',(-102.639948694851,-79.8974404698484,
228.462296651428));
#266475=CARTESIAN_POINT('Ctrl Pts',(-108.928013630747,-71.8195013191723,
226.462296651428));
#266476=CARTESIAN_POINT('Ctrl Pts',(-113.874993963172,-62.8573449296276,
224.462296651428));
#266477=CARTESIAN_POINT('Ctrl Pts',(-118.821974295598,-53.8951885400829,
222.462296651428));
#266478=CARTESIAN_POINT('Ctrl Pts',(-122.306058950682,-44.2694929456718,
220.462296651428));
#266479=CARTESIAN_POINT('Ctrl Pts',(-125.790143605767,-34.6437973512606,
218.462296651428));
#266480=CARTESIAN_POINT('Ctrl Pts',(-127.725542856289,-24.5915791233698,
216.462296651428));
#266481=CARTESIAN_POINT('Ctrl Pts',(-129.660942106811,-14.5393608954789,
214.462296651428));
#266482=CARTESIAN_POINT('Ctrl Pts',(-130.,-4.30813900827845,212.462296651428));
#266483=CARTESIAN_POINT('Ctrl Pts',(-160.,-4.30813900827851,372.462296651429));
#266484=CARTESIAN_POINT('Ctrl Pts',(-160.339057893189,8.28413408366045,
370.462296651429));
#266485=CARTESIAN_POINT('Ctrl Pts',(-158.704075916301,20.7744157382972,
368.462296651429));
#266486=CARTESIAN_POINT('Ctrl Pts',(-157.069093939413,33.2646973929339,
366.462296651429));
#266487=CARTESIAN_POINT('Ctrl Pts',(-153.500330774912,45.345435423063,364.462296651429));
#266488=CARTESIAN_POINT('Ctrl Pts',(-149.931567610412,57.4261734531921,
362.462296651429));
#266489=CARTESIAN_POINT('Ctrl Pts',(-144.516898051455,68.7998999948409,
360.462296651429));
#266490=CARTESIAN_POINT('Ctrl Pts',(-139.102228492498,80.1736265364898,
358.462296651429));
#266491=CARTESIAN_POINT('Ctrl Pts',(-131.974979673884,90.5602826949688,
356.462296651429));
#266492=CARTESIAN_POINT('Ctrl Pts',(-124.84773085527,100.946938853448,354.462296651429));
#266493=CARTESIAN_POINT('Ctrl Pts',(-116.183399296896,110.0907706828,352.462296651429));
#266494=CARTESIAN_POINT('Ctrl Pts',(-107.519067738522,119.234602512151,
350.462296651429));
#266495=CARTESIAN_POINT('Ctrl Pts',(-97.5309980386227,126.9104585261,348.462296651429));
#266496=CARTESIAN_POINT('Ctrl Pts',(-87.5429283387237,134.586314540048,
346.462296651428));
#266497=CARTESIAN_POINT('Ctrl Pts',(-76.4770599218141,140.605189688823,
344.462296651429));
#266498=CARTESIAN_POINT('Ctrl Pts',(-65.4111915049045,146.624064837598,
342.462296651429));
#266499=CARTESIAN_POINT('Ctrl Pts',(-53.5400027769202,150.837754439537,
340.462296651429));
#266500=CARTESIAN_POINT('Ctrl Pts',(-41.668814048936,155.051444041475,338.462296651429));
#266501=CARTESIAN_POINT('Ctrl Pts',(-29.2846130745767,157.356193074143,
336.462296651429));
#266502=CARTESIAN_POINT('Ctrl Pts',(-16.9004121002175,159.660942106811,
334.462296651428));
#266503=CARTESIAN_POINT('Ctrl Pts',(-4.30813900827852,160.,332.462296651429));
#266504=CARTESIAN_POINT('Ctrl Pts',(8.28413408366043,160.339057893189,330.462296651429));
#266505=CARTESIAN_POINT('Ctrl Pts',(20.7744157382972,158.704075916301,328.462296651429));
#266506=CARTESIAN_POINT('Ctrl Pts',(33.2646973929339,157.069093939413,326.462296651428));
#266507=CARTESIAN_POINT('Ctrl Pts',(45.345435423063,153.500330774912,324.462296651429));
#266508=CARTESIAN_POINT('Ctrl Pts',(57.4261734531921,149.931567610412,322.462296651428));
#266509=CARTESIAN_POINT('Ctrl Pts',(68.7998999948409,144.516898051455,320.462296651429));
#266510=CARTESIAN_POINT('Ctrl Pts',(80.1736265364898,139.102228492498,318.462296651429));
#266511=CARTESIAN_POINT('Ctrl Pts',(90.5602826949688,131.974979673884,316.462296651429));
#266512=CARTESIAN_POINT('Ctrl Pts',(100.946938853448,124.84773085527,314.462296651429));
#266513=CARTESIAN_POINT('Ctrl Pts',(110.0907706828,116.183399296896,312.462296651429));
#266514=CARTESIAN_POINT('Ctrl Pts',(119.234602512151,107.519067738522,310.462296651429));
#266515=CARTESIAN_POINT('Ctrl Pts',(126.9104585261,97.5309980386227,308.462296651429));
#266516=CARTESIAN_POINT('Ctrl Pts',(134.586314540048,87.5429283387237,306.462296651429));
#266517=CARTESIAN_POINT('Ctrl Pts',(140.605189688823,76.4770599218141,304.462296651429));
#266518=CARTESIAN_POINT('Ctrl Pts',(146.624064837598,65.4111915049045,302.462296651429));
#266519=CARTESIAN_POINT('Ctrl Pts',(150.837754439537,53.5400027769202,300.462296651429));
#266520=CARTESIAN_POINT('Ctrl Pts',(155.051444041475,41.668814048936,298.462296651429));
#266521=CARTESIAN_POINT('Ctrl Pts',(157.356193074143,29.2846130745767,296.462296651429));
#266522=CARTESIAN_POINT('Ctrl Pts',(159.660942106811,16.9004121002175,294.462296651429));
#266523=CARTESIAN_POINT('Ctrl Pts',(160.,4.30813900827853,292.462296651429));
#266524=CARTESIAN_POINT('Ctrl Pts',(160.339057893189,-8.28413408366043,
290.462296651429));
#266525=CARTESIAN_POINT('Ctrl Pts',(158.704075916301,-20.7744157382971,
288.462296651429));
#266526=CARTESIAN_POINT('Ctrl Pts',(157.069093939413,-33.2646973929339,
286.462296651429));
#266527=CARTESIAN_POINT('Ctrl Pts',(153.500330774912,-45.345435423063,284.462296651429));
#266528=CARTESIAN_POINT('Ctrl Pts',(149.931567610412,-57.4261734531921,
282.462296651429));
#266529=CARTESIAN_POINT('Ctrl Pts',(144.516898051455,-68.7998999948409,
280.462296651429));
#266530=CARTESIAN_POINT('Ctrl Pts',(139.102228492498,-80.1736265364898,
278.462296651429));
#266531=CARTESIAN_POINT('Ctrl Pts',(131.974979673884,-90.5602826949688,
276.462296651429));
#266532=CARTESIAN_POINT('Ctrl Pts',(124.84773085527,-100.946938853448,274.462296651429));
#266533=CARTESIAN_POINT('Ctrl Pts',(116.183399296896,-110.0907706828,272.462296651429));
#266534=CARTESIAN_POINT('Ctrl Pts',(107.519067738522,-119.234602512151,
270.462296651429));
#266535=CARTESIAN_POINT('Ctrl Pts',(97.5309980386227,-126.9104585261,268.462296651429));
#266536=CARTESIAN_POINT('Ctrl Pts',(87.5429283387236,-134.586314540048,
266.462296651429));
#266537=CARTESIAN_POINT('Ctrl Pts',(76.4770599218141,-140.605189688823,
264.462296651429));
#266538=CARTESIAN_POINT('Ctrl Pts',(65.4111915049046,-146.624064837598,
262.462296651429));
#266539=CARTESIAN_POINT('Ctrl Pts',(53.5400027769202,-150.837754439537,
260.462296651429));
#266540=CARTESIAN_POINT('Ctrl Pts',(41.6688140489359,-155.051444041475,
258.462296651429));
#266541=CARTESIAN_POINT('Ctrl Pts',(29.2846130745768,-157.356193074143,
256.462296651429));
#266542=CARTESIAN_POINT('Ctrl Pts',(16.9004121002176,-159.660942106811,
254.462296651429));
#266543=CARTESIAN_POINT('Ctrl Pts',(4.30813900827854,-160.,252.462296651429));
#266544=CARTESIAN_POINT('Ctrl Pts',(-8.28413408366049,-160.339057893189,
250.462296651429));
#266545=CARTESIAN_POINT('Ctrl Pts',(-20.7744157382971,-158.704075916301,
248.462296651429));
#266546=CARTESIAN_POINT('Ctrl Pts',(-33.2646973929338,-157.069093939413,
246.462296651429));
#266547=CARTESIAN_POINT('Ctrl Pts',(-45.345435423063,-153.500330774912,
244.462296651429));
#266548=CARTESIAN_POINT('Ctrl Pts',(-57.4261734531921,-149.931567610412,
242.462296651429));
#266549=CARTESIAN_POINT('Ctrl Pts',(-68.7998999948409,-144.516898051455,
240.462296651429));
#266550=CARTESIAN_POINT('Ctrl Pts',(-80.1736265364897,-139.102228492498,
238.462296651429));
#266551=CARTESIAN_POINT('Ctrl Pts',(-90.5602826949688,-131.974979673884,
236.462296651429));
#266552=CARTESIAN_POINT('Ctrl Pts',(-100.946938853448,-124.84773085527,
234.462296651429));
#266553=CARTESIAN_POINT('Ctrl Pts',(-110.0907706828,-116.183399296896,232.462296651429));
#266554=CARTESIAN_POINT('Ctrl Pts',(-119.234602512151,-107.519067738522,
230.462296651429));
#266555=CARTESIAN_POINT('Ctrl Pts',(-126.9104585261,-97.5309980386227,228.462296651429));
#266556=CARTESIAN_POINT('Ctrl Pts',(-134.586314540048,-87.5429283387236,
226.462296651429));
#266557=CARTESIAN_POINT('Ctrl Pts',(-140.605189688823,-76.4770599218141,
224.462296651429));
#266558=CARTESIAN_POINT('Ctrl Pts',(-146.624064837598,-65.4111915049046,
222.462296651429));
#266559=CARTESIAN_POINT('Ctrl Pts',(-150.837754439537,-53.5400027769203,
220.462296651429));
#266560=CARTESIAN_POINT('Ctrl Pts',(-155.051444041475,-41.668814048936,
218.462296651429));
#266561=CARTESIAN_POINT('Ctrl Pts',(-157.356193074143,-29.2846130745768,
216.462296651429));
#266562=CARTESIAN_POINT('Ctrl Pts',(-159.660942106811,-16.9004121002176,
214.462296651429));
#266563=CARTESIAN_POINT('Ctrl Pts',(-160.,-4.30813900827851,212.462296651429));
#266564=CARTESIAN_POINT('',(-128.373075022505,20.9502666088252,367.5));
#266565=CARTESIAN_POINT('',(-145.,-4.30813900827848,372.462296651428));
#266566=CARTESIAN_POINT('Origin',(-130.,-3.57353036051222E-13,375.));
#266567=CARTESIAN_POINT('Origin',(-160.,-160.339057893189,367.5));
#266568=CARTESIAN_POINT('Origin',(0.,0.,848.));
#266569=CARTESIAN_POINT('',(-3.4,-4.163799117101E-16,828.));
#266570=CARTESIAN_POINT('Origin',(0.,0.,828.));
#266571=CARTESIAN_POINT('',(-3.4,-4.163799117101E-16,848.));
#266572=CARTESIAN_POINT('',(-3.4,-4.163799117101E-16,848.));
#266573=CARTESIAN_POINT('Origin',(0.,0.,848.));
#266574=CARTESIAN_POINT('Origin',(0.,0.,828.));
#266575=CARTESIAN_POINT('',(-5.33250671116729E-15,0.,825.957073895307));
#266576=CARTESIAN_POINT('',(-3.4,-4.163799117101E-16,828.));
#266577=CARTESIAN_POINT('Origin',(-160.,-1.08084483543429E-12,695.));
#266578=CARTESIAN_POINT('',(-15.,3.28589693438513E-15,702.5));
#266579=CARTESIAN_POINT('Ctrl Pts',(-12.990381056766,-7.50000000000104,
695.));
#266580=CARTESIAN_POINT('Ctrl Pts',(-12.990381056766,-7.50000000000104,
694.037711997797));
#266581=CARTESIAN_POINT('Ctrl Pts',(-13.1086907696464,-7.30414188357672,
693.026460490526));
#266582=CARTESIAN_POINT('Ctrl Pts',(-13.5089700934546,-6.5342153230227,
691.185632303692));
#266583=CARTESIAN_POINT('Ctrl Pts',(-13.7827535066158,-5.9606687109838,
690.354066993185));
#266584=CARTESIAN_POINT('Ctrl Pts',(-14.2789995755284,-4.64772502354804,
689.041123305749));
#266585=CARTESIAN_POINT('Ctrl Pts',(-14.5369863077958,-3.8155556858589,
688.466261900566));
#266586=CARTESIAN_POINT('Ctrl Pts',(-14.8994397626298,-1.97208806616749,
687.695270705982));
#266587=CARTESIAN_POINT('Ctrl Pts',(-14.9999999999999,-0.959664758316259,
687.5));
#266588=CARTESIAN_POINT('Ctrl Pts',(-15.0000000000001,0.959664758314065,
687.5));
#266589=CARTESIAN_POINT('Ctrl Pts',(-14.8994397626301,1.97208806616529,
687.695270705982));
#266590=CARTESIAN_POINT('Ctrl Pts',(-14.5369863077964,3.81555568585669,
688.466261900566));
#266591=CARTESIAN_POINT('Ctrl Pts',(-14.2789995755291,4.64772502354583,
689.041123305749));
#266592=CARTESIAN_POINT('Ctrl Pts',(-13.7827535066168,5.96066871098163,
690.354066993185));
#266593=CARTESIAN_POINT('Ctrl Pts',(-13.5089700934557,6.53421532302054,
691.185632303692));
#266594=CARTESIAN_POINT('Ctrl Pts',(-13.1086907696476,7.30414188357456,
693.026460490526));
#266595=CARTESIAN_POINT('Ctrl Pts',(-12.9903810567672,7.49999999999887,
694.037711997797));
#266596=CARTESIAN_POINT('Ctrl Pts',(-12.9903810567672,7.49999999999887,
695.962288002204));
#266597=CARTESIAN_POINT('Ctrl Pts',(-13.1086907696476,7.30414188357456,
696.973539509475));
#266598=CARTESIAN_POINT('Ctrl Pts',(-13.5089700934557,6.53421532302054,
698.814367696309));
#266599=CARTESIAN_POINT('Ctrl Pts',(-13.7827535066168,5.96066871098163,
699.645933006816));
#266600=CARTESIAN_POINT('Ctrl Pts',(-14.2789995755291,4.64772502354583,
700.958876694252));
#266601=CARTESIAN_POINT('Ctrl Pts',(-14.5369863077964,3.81555568585669,
701.533738099435));
#266602=CARTESIAN_POINT('Ctrl Pts',(-14.8994397626301,1.97208806616529,
702.304729294019));
#266603=CARTESIAN_POINT('Ctrl Pts',(-15.0000000000001,0.959664758314061,
702.5));
#266604=CARTESIAN_POINT('Ctrl Pts',(-14.9999999999999,-0.959664758316262,
702.5));
#266605=CARTESIAN_POINT('Ctrl Pts',(-14.8994397626298,-1.9720880661675,
702.304729294019));
#266606=CARTESIAN_POINT('Ctrl Pts',(-14.5369863077958,-3.8155556858589,
701.533738099435));
#266607=CARTESIAN_POINT('Ctrl Pts',(-14.2789995755284,-4.64772502354804,
700.958876694251));
#266608=CARTESIAN_POINT('Ctrl Pts',(-13.7827535066158,-5.9606687109838,
699.645933006816));
#266609=CARTESIAN_POINT('Ctrl Pts',(-13.5089700934546,-6.5342153230227,
698.814367696309));
#266610=CARTESIAN_POINT('Ctrl Pts',(-13.1086907696464,-7.30414188357672,
696.973539509475));
#266611=CARTESIAN_POINT('Ctrl Pts',(-12.990381056766,-7.50000000000103,
695.962288002204));
#266612=CARTESIAN_POINT('Ctrl Pts',(-12.990381056766,-7.50000000000103,
695.));
#266613=CARTESIAN_POINT('',(-160.,-1.08176332053365E-12,702.5));
#266614=CARTESIAN_POINT('',(-160.,-1.08176332053365E-12,702.5));
#266615=CARTESIAN_POINT('Origin',(-160.,-1.08084483543429E-12,695.));
#266616=CARTESIAN_POINT('',(-159.937609420477,6.20654127332979,690.789436448355));
#266617=CARTESIAN_POINT('',(-129.934615416877,5.96286660784587,690.450909781394));
#266618=CARTESIAN_POINT('Ctrl Pts',(-159.937609420477,6.20654127332982,
690.789436448355));
#266619=CARTESIAN_POINT('Ctrl Pts',(-154.948459738842,6.17458452188821,
690.742330901948));
#266620=CARTESIAN_POINT('Ctrl Pts',(-149.926082303016,6.1390213471184,690.691039620133));
#266621=CARTESIAN_POINT('Ctrl Pts',(-139.949152040579,6.05906103115091,
690.579310542064));
#266622=CARTESIAN_POINT('Ctrl Pts',(-134.922635902319,6.0141024887776,690.518068863507));
#266623=CARTESIAN_POINT('Ctrl Pts',(-129.934615416877,5.96286660784588,
690.450909781394));
#266624=CARTESIAN_POINT('',(-129.869812400585,7.23822414349888,696.964207537012));
#266625=CARTESIAN_POINT('Ctrl Pts',(-129.934615416877,5.96286660784597,
690.450909781394));
#266626=CARTESIAN_POINT('Ctrl Pts',(-129.895497332176,6.3198742880004,690.918869103464));
#266627=CARTESIAN_POINT('Ctrl Pts',(-129.861734938059,6.62077691231157,
691.427509497858));
#266628=CARTESIAN_POINT('Ctrl Pts',(-129.813111426559,7.08500706130328,
692.477209818207));
#266629=CARTESIAN_POINT('Ctrl Pts',(-129.797530023073,7.25319087208374,
693.011645223298));
#266630=CARTESIAN_POINT('Ctrl Pts',(-129.785399163032,7.46764113789919,
694.107885119514));
#266631=CARTESIAN_POINT('Ctrl Pts',(-129.788874868863,7.51329980358179,
694.66573759385));
#266632=CARTESIAN_POINT('Ctrl Pts',(-129.814956867898,7.47911407824289,
695.812263009751));
#266633=CARTESIAN_POINT('Ctrl Pts',(-129.838507736136,7.39229580419887,
696.396444104027));
#266634=CARTESIAN_POINT('Ctrl Pts',(-129.869812400585,7.23822414349893,
696.964207537012));
#266635=CARTESIAN_POINT('',(-159.895664541343,7.20669984090177,697.076891283416));
#266636=CARTESIAN_POINT('Ctrl Pts',(-129.869812400585,7.23822414349889,
696.964207537012));
#266637=CARTESIAN_POINT('Ctrl Pts',(-134.859218204142,7.23191213146821,
696.987467684941));
#266638=CARTESIAN_POINT('Ctrl Pts',(-139.89584879553,7.22618364101929,697.008143200778));
#266639=CARTESIAN_POINT('Ctrl Pts',(-149.874856564711,7.21579485641644,
697.045158795903));
#266640=CARTESIAN_POINT('Ctrl Pts',(-154.905389260016,7.21104308929451,
697.061820447619));
#266641=CARTESIAN_POINT('Ctrl Pts',(-159.895664541343,7.20669984090182,
697.076891283416));
#266642=CARTESIAN_POINT('Ctrl Pts',(-159.895664541343,7.2066998409018,697.076891283416));
#266643=CARTESIAN_POINT('Ctrl Pts',(-159.870103993811,7.36226817270387,
696.537077629712));
#266644=CARTESIAN_POINT('Ctrl Pts',(-159.850674352115,7.45675253696311,
695.981314356345));
#266645=CARTESIAN_POINT('Ctrl Pts',(-159.828240589408,7.51820614028886,
694.885484288732));
#266646=CARTESIAN_POINT('Ctrl Pts',(-159.824566877554,7.4908836067602,694.349379238582));
#266647=CARTESIAN_POINT('Ctrl Pts',(-159.832377964382,7.32254333391787,
693.292150424693));
#266648=CARTESIAN_POINT('Ctrl Pts',(-159.843827611085,7.18211047599033,
692.774384904098));
#266649=CARTESIAN_POINT('Ctrl Pts',(-159.880789425704,6.78379176451796,
691.752562621326));
#266650=CARTESIAN_POINT('Ctrl Pts',(-159.906846253054,6.52166889429016,
691.253947329587));
#266651=CARTESIAN_POINT('Ctrl Pts',(-159.937609420477,6.20654127332982,
690.789436448355));
#266652=CARTESIAN_POINT('Origin',(-160.,3.64291929955129E-14,375.));
#266653=CARTESIAN_POINT('',(-15.,0.,382.5));
#266654=CARTESIAN_POINT('',(-15.,3.64291929955129E-14,367.5));
#266655=CARTESIAN_POINT('Ctrl Pts',(-15.,3.55965257270441E-14,382.5));
#266656=CARTESIAN_POINT('Ctrl Pts',(-15.,-0.959664758315123,382.5));
#266657=CARTESIAN_POINT('Ctrl Pts',(-14.8994397626299,-1.97208806616638,
382.304729294019));
#266658=CARTESIAN_POINT('Ctrl Pts',(-14.5369863077961,-3.81555568585776,
381.533738099434));
#266659=CARTESIAN_POINT('Ctrl Pts',(-14.2789995755288,-4.64772502354691,
380.958876694251));
#266660=CARTESIAN_POINT('Ctrl Pts',(-13.7827535066163,-5.96066871098269,
379.645933006816));
#266661=CARTESIAN_POINT('Ctrl Pts',(-13.5089700934551,-6.53421532302163,
378.814367696309));
#266662=CARTESIAN_POINT('Ctrl Pts',(-13.1086907696471,-7.30414188357562,
376.973539509475));
#266663=CARTESIAN_POINT('Ctrl Pts',(-12.9903810567666,-7.49999999999991,
375.962288002204));
#266664=CARTESIAN_POINT('Ctrl Pts',(-12.9903810567666,-7.49999999999991,
375.));
#266665=CARTESIAN_POINT('Ctrl Pts',(-12.9903810567666,-7.49999999999991,
374.037711997797));
#266666=CARTESIAN_POINT('Ctrl Pts',(-13.1086907696471,-7.30414188357562,
373.026460490526));
#266667=CARTESIAN_POINT('Ctrl Pts',(-13.5089700934551,-6.53421532302163,
371.185632303692));
#266668=CARTESIAN_POINT('Ctrl Pts',(-13.7827535066163,-5.96066871098269,
370.354066993185));
#266669=CARTESIAN_POINT('Ctrl Pts',(-14.2789995755288,-4.64772502354691,
369.041123305749));
#266670=CARTESIAN_POINT('Ctrl Pts',(-14.5369863077961,-3.81555568585776,
368.466261900566));
#266671=CARTESIAN_POINT('Ctrl Pts',(-14.8994397626299,-1.97208806616638,
367.695270705982));
#266672=CARTESIAN_POINT('Ctrl Pts',(-15.,-0.959664758315121,367.5));
#266673=CARTESIAN_POINT('Ctrl Pts',(-15.,3.82333054105288E-14,367.5));
#266674=CARTESIAN_POINT('',(-160.,3.55107078961524E-14,382.5));
#266675=CARTESIAN_POINT('',(-160.,3.55107078961524E-14,382.5));
#266676=CARTESIAN_POINT('Origin',(-160.,3.64291929955129E-14,375.));
#266677=CARTESIAN_POINT('Ctrl Pts',(-15.,3.64291929955129E-14,367.5));
#266678=CARTESIAN_POINT('Ctrl Pts',(-15.,0.959664758315196,367.5));
#266679=CARTESIAN_POINT('Ctrl Pts',(-14.8994397626299,1.97208806616645,
367.695270705982));
#266680=CARTESIAN_POINT('Ctrl Pts',(-14.5369863077961,3.81555568585784,
368.466261900566));
#266681=CARTESIAN_POINT('Ctrl Pts',(-14.2789995755287,4.64772502354698,
369.041123305749));
#266682=CARTESIAN_POINT('Ctrl Pts',(-13.7827535066163,5.96066871098276,
370.354066993185));
#266683=CARTESIAN_POINT('Ctrl Pts',(-13.5089700934551,6.5342153230217,371.185632303692));
#266684=CARTESIAN_POINT('Ctrl Pts',(-13.108690769647,7.30414188357569,373.026460490526));
#266685=CARTESIAN_POINT('Ctrl Pts',(-12.9903810567666,7.49999999999999,
374.037711997797));
#266686=CARTESIAN_POINT('Ctrl Pts',(-12.9903810567666,7.49999999999999,
375.962288002204));
#266687=CARTESIAN_POINT('Ctrl Pts',(-13.108690769647,7.30414188357565,376.973539509475));
#266688=CARTESIAN_POINT('Ctrl Pts',(-13.5089700934551,6.53421532302163,
378.814367696309));
#266689=CARTESIAN_POINT('Ctrl Pts',(-13.7827535066163,5.96066871098276,
379.645933006816));
#266690=CARTESIAN_POINT('Ctrl Pts',(-14.2789995755287,4.64772502354698,
380.958876694251));
#266691=CARTESIAN_POINT('Ctrl Pts',(-14.5369863077961,3.81555568585784,
381.533738099434));
#266692=CARTESIAN_POINT('Ctrl Pts',(-14.8994397626299,1.97208806616646,
382.304729294019));
#266693=CARTESIAN_POINT('Ctrl Pts',(-15.,0.959664758315197,382.5));
#266694=CARTESIAN_POINT('Ctrl Pts',(-15.,3.7470027081099E-14,382.5));
#266695=CARTESIAN_POINT('',(-159.937609420477,-6.20654127333065,379.210563551645));
#266696=CARTESIAN_POINT('',(-129.934615416877,-5.96286660784699,379.549090218607));
#266697=CARTESIAN_POINT('Ctrl Pts',(-159.937609420477,-6.20654127333066,
379.210563551645));
#266698=CARTESIAN_POINT('Ctrl Pts',(-154.948459738633,-6.17458452188773,
379.257669098055));
#266699=CARTESIAN_POINT('Ctrl Pts',(-149.926082302936,-6.13902134711856,
379.308960379868));
#266700=CARTESIAN_POINT('Ctrl Pts',(-139.949152040766,-6.05906103115325,
379.420689457935));
#266701=CARTESIAN_POINT('Ctrl Pts',(-134.92263590239,-6.01410248877932,
379.481931136493));
#266702=CARTESIAN_POINT('Ctrl Pts',(-129.934615416877,-5.9628666078469,
379.549090218607));
#266703=CARTESIAN_POINT('',(-129.869812400585,-7.23822414349998,373.035792462989));
#266704=CARTESIAN_POINT('Ctrl Pts',(-129.934615416877,-5.962866607847,379.549090218607));
#266705=CARTESIAN_POINT('Ctrl Pts',(-129.895497332176,-6.3198742880009,
379.081130896537));
#266706=CARTESIAN_POINT('Ctrl Pts',(-129.861734938059,-6.62077691231253,
378.572490502143));
#266707=CARTESIAN_POINT('Ctrl Pts',(-129.813111426559,-7.085007061304,377.522790181794));
#266708=CARTESIAN_POINT('Ctrl Pts',(-129.797530023073,-7.25319087208486,
376.988354776703));
#266709=CARTESIAN_POINT('Ctrl Pts',(-129.785399163032,-7.46764113790054,
375.892114880486));
#266710=CARTESIAN_POINT('Ctrl Pts',(-129.788874868863,-7.51329980358274,
375.334262406149));
#266711=CARTESIAN_POINT('Ctrl Pts',(-129.814956867898,-7.47911407824392,
374.18773699025));
#266712=CARTESIAN_POINT('Ctrl Pts',(-129.838507736136,-7.39229580420003,
373.603555895973));
#266713=CARTESIAN_POINT('Ctrl Pts',(-129.869812400585,-7.23822414349998,
373.035792462989));
#266714=CARTESIAN_POINT('',(-159.895664541343,-7.20669984090295,372.923108716584));
#266715=CARTESIAN_POINT('Ctrl Pts',(-129.869812400585,-7.23822414349996,
373.035792462989));
#266716=CARTESIAN_POINT('Ctrl Pts',(-134.859218204139,-7.23191213146929,
373.01253231506));
#266717=CARTESIAN_POINT('Ctrl Pts',(-139.89584879552,-7.22618364102027,
372.991856799222));
#266718=CARTESIAN_POINT('Ctrl Pts',(-149.874856564524,-7.21579485641762,
372.954841204098));
#266719=CARTESIAN_POINT('Ctrl Pts',(-154.905389259528,-7.21104308929605,
372.938179552383));
#266720=CARTESIAN_POINT('Ctrl Pts',(-159.895664541343,-7.20669984090294,
372.923108716584));
#266721=CARTESIAN_POINT('Ctrl Pts',(-159.895664541343,-7.20669984090288,
372.923108716584));
#266722=CARTESIAN_POINT('Ctrl Pts',(-159.870103993811,-7.3622681727049,
373.462922370288));
#266723=CARTESIAN_POINT('Ctrl Pts',(-159.850674352115,-7.45675253696417,
374.018685643656));
#266724=CARTESIAN_POINT('Ctrl Pts',(-159.828240589408,-7.51820614028992,
375.114515711268));
#266725=CARTESIAN_POINT('Ctrl Pts',(-159.824566877554,-7.49088360676129,
375.650620761418));
#266726=CARTESIAN_POINT('Ctrl Pts',(-159.832377964382,-7.32254333391888,
376.707849575308));
#266727=CARTESIAN_POINT('Ctrl Pts',(-159.843827611085,-7.18211047599103,
377.225615095903));
#266728=CARTESIAN_POINT('Ctrl Pts',(-159.880789425704,-6.78379176451862,
378.247437378675));
#266729=CARTESIAN_POINT('Ctrl Pts',(-159.906846253054,-6.52166889429029,
378.746052670415));
#266730=CARTESIAN_POINT('Ctrl Pts',(-159.937609420477,-6.20654127333069,
379.210563551645));
#266731=CARTESIAN_POINT('Origin',(160.,-1.08084483543429E-12,695.));
#266732=CARTESIAN_POINT('',(15.,-1.072837590456E-12,702.5));
#266733=CARTESIAN_POINT('',(15.,-1.08280927416198E-12,687.5));
#266734=CARTESIAN_POINT('Ctrl Pts',(15.,-1.07913677993565E-12,702.5));
#266735=CARTESIAN_POINT('Ctrl Pts',(14.9999999999999,-0.959664758316259,
702.5));
#266736=CARTESIAN_POINT('Ctrl Pts',(14.8994397626298,-1.97208806616749,
702.304729294019));
#266737=CARTESIAN_POINT('Ctrl Pts',(14.5369863077958,-3.8155556858589,701.533738099435));
#266738=CARTESIAN_POINT('Ctrl Pts',(14.2789995755284,-4.64772502354804,
700.958876694251));
#266739=CARTESIAN_POINT('Ctrl Pts',(13.7827535066158,-5.9606687109838,699.645933006816));
#266740=CARTESIAN_POINT('Ctrl Pts',(13.5089700934546,-6.5342153230227,698.814367696309));
#266741=CARTESIAN_POINT('Ctrl Pts',(13.1086907696464,-7.30414188357672,
696.973539509475));
#266742=CARTESIAN_POINT('Ctrl Pts',(12.990381056766,-7.50000000000103,695.962288002204));
#266743=CARTESIAN_POINT('Ctrl Pts',(12.990381056766,-7.50000000000103,694.037711997797));
#266744=CARTESIAN_POINT('Ctrl Pts',(13.1086907696464,-7.30414188357672,
693.026460490526));
#266745=CARTESIAN_POINT('Ctrl Pts',(13.5089700934546,-6.5342153230227,691.185632303692));
#266746=CARTESIAN_POINT('Ctrl Pts',(13.7827535066158,-5.9606687109838,690.354066993185));
#266747=CARTESIAN_POINT('Ctrl Pts',(14.2789995755284,-4.64772502354804,
689.041123305749));
#266748=CARTESIAN_POINT('Ctrl Pts',(14.5369863077958,-3.8155556858589,688.466261900566));
#266749=CARTESIAN_POINT('Ctrl Pts',(14.8994397626298,-1.97208806616749,
687.695270705982));
#266750=CARTESIAN_POINT('Ctrl Pts',(14.9999999999999,-0.959664758316263,
687.5));
#266751=CARTESIAN_POINT('Ctrl Pts',(15.,-1.08385522779031E-12,687.5));
#266752=CARTESIAN_POINT('',(160.,-1.08176332053365E-12,687.5));
#266753=CARTESIAN_POINT('',(160.,-1.08176332053365E-12,687.5));
#266754=CARTESIAN_POINT('Origin',(160.,-1.08084483543429E-12,695.));
#266755=CARTESIAN_POINT('Ctrl Pts',(15.,-1.0845491171807E-12,687.5));
#266756=CARTESIAN_POINT('Ctrl Pts',(15.0000000000001,0.959664758314058,
687.5));
#266757=CARTESIAN_POINT('Ctrl Pts',(14.8994397626301,1.97208806616529,687.695270705982));
#266758=CARTESIAN_POINT('Ctrl Pts',(14.5369863077964,3.81555568585669,688.466261900566));
#266759=CARTESIAN_POINT('Ctrl Pts',(14.2789995755291,4.64772502354583,689.041123305749));
#266760=CARTESIAN_POINT('Ctrl Pts',(13.7827535066168,5.96066871098163,690.354066993185));
#266761=CARTESIAN_POINT('Ctrl Pts',(13.5089700934557,6.53421532302054,691.185632303692));
#266762=CARTESIAN_POINT('Ctrl Pts',(13.1086907696476,7.30414188357456,693.026460490526));
#266763=CARTESIAN_POINT('Ctrl Pts',(12.9903810567672,7.49999999999887,694.037711997797));
#266764=CARTESIAN_POINT('Ctrl Pts',(12.9903810567672,7.49999999999887,695.));
#266765=CARTESIAN_POINT('Ctrl Pts',(12.9903810567672,7.49999999999887,695.962288002204));
#266766=CARTESIAN_POINT('Ctrl Pts',(13.1086907696476,7.30414188357456,696.973539509475));
#266767=CARTESIAN_POINT('Ctrl Pts',(13.5089700934557,6.53421532302054,698.814367696309));
#266768=CARTESIAN_POINT('Ctrl Pts',(13.7827535066168,5.96066871098163,699.645933006816));
#266769=CARTESIAN_POINT('Ctrl Pts',(14.2789995755291,4.64772502354583,700.958876694252));
#266770=CARTESIAN_POINT('Ctrl Pts',(14.5369863077964,3.81555568585669,701.533738099435));
#266771=CARTESIAN_POINT('Ctrl Pts',(14.8994397626301,1.97208806616529,702.304729294019));
#266772=CARTESIAN_POINT('Ctrl Pts',(15.0000000000001,0.959664758314059,
702.5));
#266773=CARTESIAN_POINT('Ctrl Pts',(15.,-1.08468789505878E-12,702.5));
#266774=CARTESIAN_POINT('',(159.937609420477,-6.20654127333164,690.789436448355));
#266775=CARTESIAN_POINT('',(159.895664541343,-7.20669984090406,697.076891283416));
#266776=CARTESIAN_POINT('Ctrl Pts',(159.937609420477,-6.20654127333163,
690.789436448355));
#266777=CARTESIAN_POINT('Ctrl Pts',(159.906834643176,-6.52178782200797,
691.254122633859));
#266778=CARTESIAN_POINT('Ctrl Pts',(159.880769856038,-6.78398922241133,
691.752938404992));
#266779=CARTESIAN_POINT('Ctrl Pts',(159.843804521963,-7.18237209951024,
692.775180680853));
#266780=CARTESIAN_POINT('Ctrl Pts',(159.832358861788,-7.32279367879376,
693.293160677924));
#266781=CARTESIAN_POINT('Ctrl Pts',(159.824570869009,-7.49095925222209,
694.350417431358));
#266782=CARTESIAN_POINT('Ctrl Pts',(159.82825204698,-7.51820444472976,694.8863221477));
#266783=CARTESIAN_POINT('Ctrl Pts',(159.850688911066,-7.45668143260721,
695.981732982313));
#266784=CARTESIAN_POINT('Ctrl Pts',(159.870113636375,-7.36220948547999,
696.537281271196));
#266785=CARTESIAN_POINT('Ctrl Pts',(159.895664541343,-7.2066998409041,697.076891283416));
#266786=CARTESIAN_POINT('',(129.934615416877,-5.96286660784778,690.450909781393));
#266787=CARTESIAN_POINT('Ctrl Pts',(129.934615416877,-5.96286660784775,
690.450909781393));
#266788=CARTESIAN_POINT('Ctrl Pts',(134.922636022201,-6.01410249001088,
690.518068865121));
#266789=CARTESIAN_POINT('Ctrl Pts',(139.949152283076,-6.05906103332323,
690.579310545018));
#266790=CARTESIAN_POINT('Ctrl Pts',(149.926082545137,-6.13902134883337,
690.691039622605));
#266791=CARTESIAN_POINT('Ctrl Pts',(154.948459858584,-6.17458452265701,
690.742330903078));
#266792=CARTESIAN_POINT('Ctrl Pts',(159.937609420477,-6.20654127333165,
690.789436448355));
#266793=CARTESIAN_POINT('',(129.869812400585,-7.23822414350117,696.964207537011));
#266794=CARTESIAN_POINT('Ctrl Pts',(129.869812400585,-7.23822414350118,
696.964207537011));
#266795=CARTESIAN_POINT('Ctrl Pts',(129.838465947162,-7.3925014763172,696.39568618978));
#266796=CARTESIAN_POINT('Ctrl Pts',(129.814894504108,-7.4793450036484,695.810706203687));
#266797=CARTESIAN_POINT('Ctrl Pts',(129.788829961956,-7.5132167397021,694.662636602978));
#266798=CARTESIAN_POINT('Ctrl Pts',(129.785389515462,-7.46723834799325,
694.104054596373));
#266799=CARTESIAN_POINT('Ctrl Pts',(129.797623339578,-7.25211847571097,
693.007946909601));
#266800=CARTESIAN_POINT('Ctrl Pts',(129.813220504589,-7.08391429791459,
692.474308019488));
#266801=CARTESIAN_POINT('Ctrl Pts',(129.861824504594,-6.61997620179538,
691.426155633436));
#266802=CARTESIAN_POINT('Ctrl Pts',(129.895549481156,-6.31939835503028,
690.918245258983));
#266803=CARTESIAN_POINT('Ctrl Pts',(129.934615416877,-5.96286660784783,
690.450909781393));
#266804=CARTESIAN_POINT('Ctrl Pts',(159.895664541343,-7.20669984090407,
697.076891283416));
#266805=CARTESIAN_POINT('Ctrl Pts',(154.905389419006,-7.21104308915838,
697.061820448099));
#266806=CARTESIAN_POINT('Ctrl Pts',(149.874856855226,-7.21579485612801,
697.04515879687));
#266807=CARTESIAN_POINT('Ctrl Pts',(139.895849065302,-7.22618364069772,
697.008143201895));
#266808=CARTESIAN_POINT('Ctrl Pts',(134.859218339046,-7.2319121312998,696.98746768557));
#266809=CARTESIAN_POINT('Ctrl Pts',(129.869812400585,-7.23822414350115,
696.964207537012));
#266810=CARTESIAN_POINT('Origin',(160.,3.64291929955129E-14,375.));
#266811=CARTESIAN_POINT('',(15.,1.83697019872103E-15,382.5));
#266812=CARTESIAN_POINT('',(15.,3.64291929155445E-14,367.5));
#266813=CARTESIAN_POINT('Ctrl Pts',(15.,3.64291929955129E-14,382.5));
#266814=CARTESIAN_POINT('Ctrl Pts',(15.,-0.959664758315123,382.5));
#266815=CARTESIAN_POINT('Ctrl Pts',(14.8994397626299,-1.97208806616638,
382.304729294019));
#266816=CARTESIAN_POINT('Ctrl Pts',(14.5369863077961,-3.81555568585776,
381.533738099434));
#266817=CARTESIAN_POINT('Ctrl Pts',(14.2789995755288,-4.64772502354691,
380.958876694251));
#266818=CARTESIAN_POINT('Ctrl Pts',(13.7827535066163,-5.96066871098269,
379.645933006816));
#266819=CARTESIAN_POINT('Ctrl Pts',(13.5089700934552,-6.53421532302156,
378.814367696309));
#266820=CARTESIAN_POINT('Ctrl Pts',(13.1086907696471,-7.30414188357558,
376.973539509475));
#266821=CARTESIAN_POINT('Ctrl Pts',(12.9903810567666,-7.49999999999991,
375.962288002204));
#266822=CARTESIAN_POINT('Ctrl Pts',(12.9903810567666,-7.49999999999991,
374.037711997797));
#266823=CARTESIAN_POINT('Ctrl Pts',(13.1086907696471,-7.30414188357562,
373.026460490526));
#266824=CARTESIAN_POINT('Ctrl Pts',(13.5089700934551,-6.53421532302163,
371.185632303692));
#266825=CARTESIAN_POINT('Ctrl Pts',(13.7827535066163,-5.96066871098269,
370.354066993185));
#266826=CARTESIAN_POINT('Ctrl Pts',(14.2789995755288,-4.64772502354691,
369.041123305749));
#266827=CARTESIAN_POINT('Ctrl Pts',(14.5369863077961,-3.81555568585776,
368.466261900566));
#266828=CARTESIAN_POINT('Ctrl Pts',(14.8994397626299,-1.97208806616638,
367.695270705982));
#266829=CARTESIAN_POINT('Ctrl Pts',(15.,-0.959664758315123,367.5));
#266830=CARTESIAN_POINT('Ctrl Pts',(15.,3.60822483003176E-14,367.5));
#266831=CARTESIAN_POINT('',(160.,3.55107078961524E-14,367.5));
#266832=CARTESIAN_POINT('',(160.,3.55107078961524E-14,367.5));
#266833=CARTESIAN_POINT('Origin',(160.,3.64291929955129E-14,375.));
#266834=CARTESIAN_POINT('Ctrl Pts',(15.,3.73312492030209E-14,367.5));
#266835=CARTESIAN_POINT('Ctrl Pts',(15.,0.959664758315197,367.5));
#266836=CARTESIAN_POINT('Ctrl Pts',(14.8994397626299,1.97208806616646,367.695270705982));
#266837=CARTESIAN_POINT('Ctrl Pts',(14.5369863077961,3.81555568585784,368.466261900566));
#266838=CARTESIAN_POINT('Ctrl Pts',(14.2789995755287,4.64772502354698,369.041123305749));
#266839=CARTESIAN_POINT('Ctrl Pts',(13.7827535066163,5.96066871098276,370.354066993185));
#266840=CARTESIAN_POINT('Ctrl Pts',(13.5089700934551,6.5342153230217,371.185632303692));
#266841=CARTESIAN_POINT('Ctrl Pts',(13.108690769647,7.30414188357569,373.026460490526));
#266842=CARTESIAN_POINT('Ctrl Pts',(12.9903810567666,7.49999999999999,374.037711997797));
#266843=CARTESIAN_POINT('Ctrl Pts',(12.9903810567666,7.49999999999999,375.));
#266844=CARTESIAN_POINT('Ctrl Pts',(12.9903810567666,7.49999999999999,375.962288002204));
#266845=CARTESIAN_POINT('Ctrl Pts',(13.108690769647,7.30414188357569,376.973539509475));
#266846=CARTESIAN_POINT('Ctrl Pts',(13.5089700934551,6.5342153230217,378.814367696309));
#266847=CARTESIAN_POINT('Ctrl Pts',(13.7827535066163,5.96066871098276,379.645933006816));
#266848=CARTESIAN_POINT('Ctrl Pts',(14.2789995755287,4.64772502354698,380.958876694251));
#266849=CARTESIAN_POINT('Ctrl Pts',(14.5369863077961,3.81555568585778,381.533738099435));
#266850=CARTESIAN_POINT('Ctrl Pts',(14.8994397626299,1.97208806616639,382.304729294019));
#266851=CARTESIAN_POINT('Ctrl Pts',(15.,0.959664758315195,382.5));
#266852=CARTESIAN_POINT('Ctrl Pts',(15.,3.46944695195361E-14,382.5));
#266853=CARTESIAN_POINT('',(129.869812400585,7.23822414350007,373.035792462989));
#266854=CARTESIAN_POINT('',(129.934615416877,5.96286660784696,379.549090218607));
#266855=CARTESIAN_POINT('Ctrl Pts',(129.869812400585,7.23822414350003,373.035792462989));
#266856=CARTESIAN_POINT('Ctrl Pts',(129.838465947162,7.39250147631606,373.60431381022));
#266857=CARTESIAN_POINT('Ctrl Pts',(129.814894504108,7.47934500364732,374.189293796313));
#266858=CARTESIAN_POINT('Ctrl Pts',(129.788829961956,7.51321673970108,375.337363397022));
#266859=CARTESIAN_POINT('Ctrl Pts',(129.785389515462,7.4672383479923,375.895945403626));
#266860=CARTESIAN_POINT('Ctrl Pts',(129.797623339578,7.25211847571004,376.9920530904));
#266861=CARTESIAN_POINT('Ctrl Pts',(129.813220504589,7.08391429791338,377.525691980513));
#266862=CARTESIAN_POINT('Ctrl Pts',(129.861824504594,6.61997620179469,378.573844366563));
#266863=CARTESIAN_POINT('Ctrl Pts',(129.895549481156,6.31939835502988,379.081754741017));
#266864=CARTESIAN_POINT('Ctrl Pts',(129.934615416877,5.96286660784708,379.549090218607));
#266865=CARTESIAN_POINT('',(159.895664541343,7.20669984090294,372.923108716584));
#266866=CARTESIAN_POINT('Ctrl Pts',(159.895664541343,7.20669984090292,372.923108716584));
#266867=CARTESIAN_POINT('Ctrl Pts',(154.905389418371,7.21104308915779,372.938179551903));
#266868=CARTESIAN_POINT('Ctrl Pts',(149.874856854973,7.21579485612699,372.954841203131));
#266869=CARTESIAN_POINT('Ctrl Pts',(139.895849065092,7.22618364069654,372.991856798107));
#266870=CARTESIAN_POINT('Ctrl Pts',(134.85921833898,7.23191213129876,373.012532314431));
#266871=CARTESIAN_POINT('Ctrl Pts',(129.869812400585,7.23822414350003,373.035792462989));
#266872=CARTESIAN_POINT('',(159.937609420477,6.20654127333073,379.210563551645));
#266873=CARTESIAN_POINT('Ctrl Pts',(159.937609420477,6.20654127333081,379.210563551645));
#266874=CARTESIAN_POINT('Ctrl Pts',(159.906834643176,6.52178782200678,378.745877366142));
#266875=CARTESIAN_POINT('Ctrl Pts',(159.880769856038,6.78398922241033,378.247061595009));
#266876=CARTESIAN_POINT('Ctrl Pts',(159.843804521963,7.18237209951068,377.224819319144));
#266877=CARTESIAN_POINT('Ctrl Pts',(159.832358861788,7.32279367879272,376.706839322075));
#266878=CARTESIAN_POINT('Ctrl Pts',(159.824570869009,7.49095925222048,375.649582568643));
#266879=CARTESIAN_POINT('Ctrl Pts',(159.82825204698,7.51820444472885,375.113677852303));
#266880=CARTESIAN_POINT('Ctrl Pts',(159.850688911066,7.45668143260609,374.018267017687));
#266881=CARTESIAN_POINT('Ctrl Pts',(159.870113636375,7.36220948547902,373.462718728805));
#266882=CARTESIAN_POINT('Ctrl Pts',(159.895664541343,7.20669984090294,372.923108716584));
#266883=CARTESIAN_POINT('Ctrl Pts',(129.934615416877,5.96286660784695,379.549090218607));
#266884=CARTESIAN_POINT('Ctrl Pts',(134.922636022203,6.01410249001008,379.48193113488));
#266885=CARTESIAN_POINT('Ctrl Pts',(139.949152283082,6.05906103332244,379.420689454983));
#266886=CARTESIAN_POINT('Ctrl Pts',(149.926082545118,6.13902134883237,379.308960377395));
#266887=CARTESIAN_POINT('Ctrl Pts',(154.948459858534,6.17458452265582,379.257669096923));
#266888=CARTESIAN_POINT('Ctrl Pts',(159.937609420477,6.20654127333077,379.210563551645));
#266889=CARTESIAN_POINT('Origin',(160.,3.64291929955129E-14,535.));
#266890=CARTESIAN_POINT('',(15.,1.83697027874617E-15,527.5));
#266891=CARTESIAN_POINT('',(15.,1.64287496604076E-14,542.5));
#266892=CARTESIAN_POINT('Ctrl Pts',(15.,2.99760216648792E-14,527.5));
#266893=CARTESIAN_POINT('Ctrl Pts',(15.,-0.959664758315129,527.5));
#266894=CARTESIAN_POINT('Ctrl Pts',(14.8994397626299,-1.97208806616637,
527.695270705982));
#266895=CARTESIAN_POINT('Ctrl Pts',(14.5369863077961,-3.81555568585775,
528.466261900566));
#266896=CARTESIAN_POINT('Ctrl Pts',(14.2789995755288,-4.64772502354691,
529.041123305749));
#266897=CARTESIAN_POINT('Ctrl Pts',(13.7827535066163,-5.96066871098269,
530.354066993185));
#266898=CARTESIAN_POINT('Ctrl Pts',(13.5089700934551,-6.53421532302163,
531.185632303692));
#266899=CARTESIAN_POINT('Ctrl Pts',(13.1086907696471,-7.30414188357563,
533.026460490526));
#266900=CARTESIAN_POINT('Ctrl Pts',(12.9903810567666,-7.49999999999991,
534.037711997796));
#266901=CARTESIAN_POINT('Ctrl Pts',(12.9903810567666,-7.49999999999991,
535.962288002204));
#266902=CARTESIAN_POINT('Ctrl Pts',(13.1086907696471,-7.3041418835756,536.973539509475));
#266903=CARTESIAN_POINT('Ctrl Pts',(13.5089700934552,-6.53421532302157,
538.814367696309));
#266904=CARTESIAN_POINT('Ctrl Pts',(13.7827535066163,-5.96066871098269,
539.645933006816));
#266905=CARTESIAN_POINT('Ctrl Pts',(14.2789995755288,-4.64772502354691,
540.958876694251));
#266906=CARTESIAN_POINT('Ctrl Pts',(14.5369863077961,-3.81555568585775,
541.533738099434));
#266907=CARTESIAN_POINT('Ctrl Pts',(14.8994397626299,-1.97208806616637,
542.304729294019));
#266908=CARTESIAN_POINT('Ctrl Pts',(15.,-0.959664758315122,542.5));
#266909=CARTESIAN_POINT('Ctrl Pts',(15.,3.77475828372553E-14,542.5));
#266910=CARTESIAN_POINT('',(160.,3.55107078961524E-14,527.5));
#266911=CARTESIAN_POINT('',(160.,3.55107078961524E-14,527.5));
#266912=CARTESIAN_POINT('Origin',(160.,3.64291929955129E-14,535.));
#266913=CARTESIAN_POINT('Ctrl Pts',(15.,3.44169137633799E-14,542.5));
#266914=CARTESIAN_POINT('Ctrl Pts',(15.,0.959664758315194,542.5));
#266915=CARTESIAN_POINT('Ctrl Pts',(14.8994397626299,1.97208806616644,542.304729294019));
#266916=CARTESIAN_POINT('Ctrl Pts',(14.5369863077961,3.81555568585783,541.533738099434));
#266917=CARTESIAN_POINT('Ctrl Pts',(14.2789995755287,4.64772502354698,540.958876694251));
#266918=CARTESIAN_POINT('Ctrl Pts',(13.7827535066163,5.96066871098276,539.645933006816));
#266919=CARTESIAN_POINT('Ctrl Pts',(13.5089700934551,6.53421532302171,538.814367696309));
#266920=CARTESIAN_POINT('Ctrl Pts',(13.108690769647,7.30414188357571,536.973539509475));
#266921=CARTESIAN_POINT('Ctrl Pts',(12.9903810567666,7.49999999999999,535.962288002204));
#266922=CARTESIAN_POINT('Ctrl Pts',(12.9903810567666,7.49999999999999,535.));
#266923=CARTESIAN_POINT('Ctrl Pts',(12.9903810567666,7.49999999999999,534.037711997796));
#266924=CARTESIAN_POINT('Ctrl Pts',(13.108690769647,7.30414188357571,533.026460490526));
#266925=CARTESIAN_POINT('Ctrl Pts',(13.5089700934551,6.53421532302171,531.185632303692));
#266926=CARTESIAN_POINT('Ctrl Pts',(13.7827535066163,5.96066871098276,530.354066993185));
#266927=CARTESIAN_POINT('Ctrl Pts',(14.2789995755287,4.64772502354698,529.041123305749));
#266928=CARTESIAN_POINT('Ctrl Pts',(14.5369863077961,3.81555568585783,528.466261900566));
#266929=CARTESIAN_POINT('Ctrl Pts',(14.8994397626299,1.97208806616644,527.695270705982));
#266930=CARTESIAN_POINT('Ctrl Pts',(15.,0.959664758315196,527.5));
#266931=CARTESIAN_POINT('Ctrl Pts',(15.,3.71924713249427E-14,527.5));
#266932=CARTESIAN_POINT('',(129.869812400585,-7.23822414349995,536.964207537012));
#266933=CARTESIAN_POINT('',(159.895664541343,-7.20669984090288,537.076891283416));
#266934=CARTESIAN_POINT('Ctrl Pts',(129.869812400585,-7.23822414349994,
536.964207537012));
#266935=CARTESIAN_POINT('Ctrl Pts',(134.859218204053,-7.23191213146938,
536.98746768494));
#266936=CARTESIAN_POINT('Ctrl Pts',(139.895848795289,-7.22618364102058,
537.008143200777));
#266937=CARTESIAN_POINT('Ctrl Pts',(149.874856564741,-7.21579485641745,
537.045158795903));
#266938=CARTESIAN_POINT('Ctrl Pts',(154.905389260097,-7.21104308929549,
537.061820447619));
#266939=CARTESIAN_POINT('Ctrl Pts',(159.895664541343,-7.20669984090287,
537.076891283416));
#266940=CARTESIAN_POINT('',(159.937609420477,-6.20654127333069,530.789436448355));
#266941=CARTESIAN_POINT('Ctrl Pts',(159.895664541343,-7.20669984090287,
537.076891283416));
#266942=CARTESIAN_POINT('Ctrl Pts',(159.870103993811,-7.36226817270497,
536.537077629712));
#266943=CARTESIAN_POINT('Ctrl Pts',(159.850674352115,-7.45675253696416,
535.981314356344));
#266944=CARTESIAN_POINT('Ctrl Pts',(159.828240589408,-7.51820614028994,
534.885484288732));
#266945=CARTESIAN_POINT('Ctrl Pts',(159.824566877554,-7.4908836067612,534.349379238582));
#266946=CARTESIAN_POINT('Ctrl Pts',(159.832377964382,-7.32254333391886,
533.292150424692));
#266947=CARTESIAN_POINT('Ctrl Pts',(159.843827611085,-7.18211047599137,
532.774384904098));
#266948=CARTESIAN_POINT('Ctrl Pts',(159.880789425704,-6.78379176451867,
531.752562621325));
#266949=CARTESIAN_POINT('Ctrl Pts',(159.906846253054,-6.52166889429031,
531.253947329586));
#266950=CARTESIAN_POINT('Ctrl Pts',(159.937609420477,-6.20654127333076,
530.789436448355));
#266951=CARTESIAN_POINT('',(129.934615416877,-5.96286660784692,530.450909781393));
#266952=CARTESIAN_POINT('Ctrl Pts',(159.937609420477,-6.20654127333072,
530.789436448355));
#266953=CARTESIAN_POINT('Ctrl Pts',(154.948459738742,-6.17458452188848,
530.742330901947));
#266954=CARTESIAN_POINT('Ctrl Pts',(149.926082302978,-6.13902134711897,
530.691039620133));
#266955=CARTESIAN_POINT('Ctrl Pts',(139.949152040648,-6.05906103115236,
530.579310542064));
#266956=CARTESIAN_POINT('Ctrl Pts',(134.922635902346,-6.0141024887789,530.518068863507));
#266957=CARTESIAN_POINT('Ctrl Pts',(129.934615416877,-5.96286660784692,
530.450909781393));
#266958=CARTESIAN_POINT('Ctrl Pts',(129.934615416877,-5.96286660784692,
530.450909781393));
#266959=CARTESIAN_POINT('Ctrl Pts',(129.895497332176,-6.3198742880018,530.918869103465));
#266960=CARTESIAN_POINT('Ctrl Pts',(129.861734938059,-6.62077691231277,
531.427509497859));
#266961=CARTESIAN_POINT('Ctrl Pts',(129.813111426559,-7.0850070613043,532.477209818207));
#266962=CARTESIAN_POINT('Ctrl Pts',(129.797530023073,-7.25319087208485,
533.011645223299));
#266963=CARTESIAN_POINT('Ctrl Pts',(129.785399163032,-7.46764113790021,
534.107885119514));
#266964=CARTESIAN_POINT('Ctrl Pts',(129.788874868863,-7.51329980358284,
534.66573759385));
#266965=CARTESIAN_POINT('Ctrl Pts',(129.814956867898,-7.47911407824392,
535.812263009751));
#266966=CARTESIAN_POINT('Ctrl Pts',(129.838507736136,-7.39229580419984,
536.396444104028));
#266967=CARTESIAN_POINT('Ctrl Pts',(129.869812400585,-7.23822414349995,
536.964207537012));
#266968=CARTESIAN_POINT('',(159.937609420477,6.20654127333082,539.210563551645));
#266969=CARTESIAN_POINT('',(159.895664541343,7.20669984090288,532.923108716584));
#266970=CARTESIAN_POINT('Ctrl Pts',(159.937609420477,6.20654127333076,539.210563551645));
#266971=CARTESIAN_POINT('Ctrl Pts',(159.906834643176,6.52178782200697,538.745877366142));
#266972=CARTESIAN_POINT('Ctrl Pts',(159.880769856038,6.78398922241032,538.247061595009));
#266973=CARTESIAN_POINT('Ctrl Pts',(159.843804521963,7.18237209950917,537.224819319147));
#266974=CARTESIAN_POINT('Ctrl Pts',(159.832358861788,7.32279367879273,536.706839322077));
#266975=CARTESIAN_POINT('Ctrl Pts',(159.824570869009,7.49095925222104,535.649582568642));
#266976=CARTESIAN_POINT('Ctrl Pts',(159.82825204698,7.51820444472875,535.113677852301));
#266977=CARTESIAN_POINT('Ctrl Pts',(159.850688911066,7.45668143260613,534.018267017687));
#266978=CARTESIAN_POINT('Ctrl Pts',(159.870113636375,7.36220948547888,533.462718728804));
#266979=CARTESIAN_POINT('Ctrl Pts',(159.895664541343,7.20669984090294,532.923108716584));
#266980=CARTESIAN_POINT('',(129.934615416877,5.96286660784701,539.549090218607));
#266981=CARTESIAN_POINT('Ctrl Pts',(129.934615416877,5.96286660784688,539.549090218607));
#266982=CARTESIAN_POINT('Ctrl Pts',(134.922636022207,6.01410249001005,539.48193113488));
#266983=CARTESIAN_POINT('Ctrl Pts',(139.949152283091,6.05906103332251,539.420689454982));
#266984=CARTESIAN_POINT('Ctrl Pts',(149.926082545092,6.13902134883217,539.308960377395));
#266985=CARTESIAN_POINT('Ctrl Pts',(154.948459858468,6.17458452265536,539.257669096923));
#266986=CARTESIAN_POINT('Ctrl Pts',(159.937609420477,6.20654127333074,539.210563551645));
#266987=CARTESIAN_POINT('',(129.869812400585,7.23822414350004,533.035792462989));
#266988=CARTESIAN_POINT('Ctrl Pts',(129.869812400585,7.23822414350011,533.035792462989));
#266989=CARTESIAN_POINT('Ctrl Pts',(129.838465947162,7.39250147631596,533.60431381022));
#266990=CARTESIAN_POINT('Ctrl Pts',(129.814894504108,7.4793450036473,534.189293796313));
#266991=CARTESIAN_POINT('Ctrl Pts',(129.788829961956,7.51321673970109,535.337363397021));
#266992=CARTESIAN_POINT('Ctrl Pts',(129.785389515462,7.46723834799247,535.895945403626));
#266993=CARTESIAN_POINT('Ctrl Pts',(129.797623339578,7.2521184757102,536.992053090399));
#266994=CARTESIAN_POINT('Ctrl Pts',(129.813220504589,7.08391429791336,537.525691980513));
#266995=CARTESIAN_POINT('Ctrl Pts',(129.861824504594,6.61997620179435,538.573844366564));
#266996=CARTESIAN_POINT('Ctrl Pts',(129.895549481156,6.31939835502854,539.081754741018));
#266997=CARTESIAN_POINT('Ctrl Pts',(129.934615416877,5.96286660784697,539.549090218607));
#266998=CARTESIAN_POINT('Ctrl Pts',(159.895664541343,7.20669984090296,532.923108716584));
#266999=CARTESIAN_POINT('Ctrl Pts',(154.905389417752,7.21104308915837,532.938179551905));
#267000=CARTESIAN_POINT('Ctrl Pts',(149.87485685474,7.21579485612754,532.954841203132));
#267001=CARTESIAN_POINT('Ctrl Pts',(139.895849065202,7.22618364069673,532.991856798106));
#267002=CARTESIAN_POINT('Ctrl Pts',(134.859218339019,7.23191213129876,533.012532314431));
#267003=CARTESIAN_POINT('Ctrl Pts',(129.869812400585,7.23822414350007,533.035792462989));
#267004=CARTESIAN_POINT('Origin',(-160.,3.64291929955129E-14,535.));
#267005=CARTESIAN_POINT('',(-15.,4.80562938205009E-14,527.5));
#267006=CARTESIAN_POINT('',(-15.,3.70454790009383E-14,542.5));
#267007=CARTESIAN_POINT('Ctrl Pts',(-15.,3.1641356201817E-14,527.5));
#267008=CARTESIAN_POINT('Ctrl Pts',(-15.,-0.959664758315127,527.5));
#267009=CARTESIAN_POINT('Ctrl Pts',(-14.8994397626299,-1.97208806616637,
527.695270705982));
#267010=CARTESIAN_POINT('Ctrl Pts',(-14.5369863077961,-3.81555568585775,
528.466261900566));
#267011=CARTESIAN_POINT('Ctrl Pts',(-14.2789995755288,-4.64772502354691,
529.041123305749));
#267012=CARTESIAN_POINT('Ctrl Pts',(-13.7827535066163,-5.96066871098269,
530.354066993185));
#267013=CARTESIAN_POINT('Ctrl Pts',(-13.5089700934551,-6.53421532302163,
531.185632303692));
#267014=CARTESIAN_POINT('Ctrl Pts',(-13.1086907696471,-7.30414188357563,
533.026460490526));
#267015=CARTESIAN_POINT('Ctrl Pts',(-12.9903810567666,-7.49999999999991,
534.037711997796));
#267016=CARTESIAN_POINT('Ctrl Pts',(-12.9903810567666,-7.49999999999991,
535.));
#267017=CARTESIAN_POINT('Ctrl Pts',(-12.9903810567666,-7.49999999999991,
535.962288002204));
#267018=CARTESIAN_POINT('Ctrl Pts',(-13.1086907696471,-7.30414188357563,
536.973539509475));
#267019=CARTESIAN_POINT('Ctrl Pts',(-13.5089700934551,-6.53421532302163,
538.814367696309));
#267020=CARTESIAN_POINT('Ctrl Pts',(-13.7827535066163,-5.96066871098269,
539.645933006816));
#267021=CARTESIAN_POINT('Ctrl Pts',(-14.2789995755288,-4.64772502354691,
540.958876694251));
#267022=CARTESIAN_POINT('Ctrl Pts',(-14.5369863077961,-3.81555568585775,
541.533738099434));
#267023=CARTESIAN_POINT('Ctrl Pts',(-14.8994397626299,-1.97208806616637,
542.304729294019));
#267024=CARTESIAN_POINT('Ctrl Pts',(-15.,-0.959664758315135,542.5));
#267025=CARTESIAN_POINT('Ctrl Pts',(-15.,2.44249065417534E-14,542.5));
#267026=CARTESIAN_POINT('',(-160.,3.55107078961524E-14,542.5));
#267027=CARTESIAN_POINT('',(-160.,3.55107078961524E-14,542.5));
#267028=CARTESIAN_POINT('Origin',(-160.,3.64291929955129E-14,535.));
#267029=CARTESIAN_POINT('Ctrl Pts',(-15.,3.56659146660832E-14,542.5));
#267030=CARTESIAN_POINT('Ctrl Pts',(-15.,0.959664758315195,542.5));
#267031=CARTESIAN_POINT('Ctrl Pts',(-14.8994397626299,1.97208806616644,
542.304729294019));
#267032=CARTESIAN_POINT('Ctrl Pts',(-14.5369863077961,3.81555568585783,
541.533738099434));
#267033=CARTESIAN_POINT('Ctrl Pts',(-14.2789995755287,4.64772502354698,
540.958876694251));
#267034=CARTESIAN_POINT('Ctrl Pts',(-13.7827535066163,5.96066871098276,
539.645933006816));
#267035=CARTESIAN_POINT('Ctrl Pts',(-13.5089700934551,6.53421532302164,
538.814367696309));
#267036=CARTESIAN_POINT('Ctrl Pts',(-13.108690769647,7.30414188357567,536.973539509475));
#267037=CARTESIAN_POINT('Ctrl Pts',(-12.9903810567666,7.49999999999999,
535.962288002204));
#267038=CARTESIAN_POINT('Ctrl Pts',(-12.9903810567666,7.49999999999999,
534.037711997797));
#267039=CARTESIAN_POINT('Ctrl Pts',(-13.108690769647,7.30414188357571,533.026460490526));
#267040=CARTESIAN_POINT('Ctrl Pts',(-13.5089700934551,6.53421532302171,
531.185632303692));
#267041=CARTESIAN_POINT('Ctrl Pts',(-13.7827535066163,5.96066871098276,
530.354066993185));
#267042=CARTESIAN_POINT('Ctrl Pts',(-14.2789995755287,4.64772502354698,
529.041123305749));
#267043=CARTESIAN_POINT('Ctrl Pts',(-14.5369863077961,3.81555568585786,
528.466261900566));
#267044=CARTESIAN_POINT('Ctrl Pts',(-14.8994397626299,1.97208806616648,
527.695270705982));
#267045=CARTESIAN_POINT('Ctrl Pts',(-15.,0.959664758315195,527.5));
#267046=CARTESIAN_POINT('Ctrl Pts',(-15.,3.5527136788005E-14,527.5));
#267047=CARTESIAN_POINT('',(-159.937609420477,-6.20654127333065,539.210563551645));
#267048=CARTESIAN_POINT('',(-129.934615416877,-5.96286660784691,539.549090218607));
#267049=CARTESIAN_POINT('Ctrl Pts',(-159.937609420477,-6.20654127333064,
539.210563551645));
#267050=CARTESIAN_POINT('Ctrl Pts',(-154.948459738632,-6.1745845218877,
539.257669098055));
#267051=CARTESIAN_POINT('Ctrl Pts',(-149.926082302935,-6.13902134711855,
539.308960379868));
#267052=CARTESIAN_POINT('Ctrl Pts',(-139.949152040724,-6.05906103115291,
539.420689457936));
#267053=CARTESIAN_POINT('Ctrl Pts',(-134.922635902374,-6.01410248877916,
539.481931136493));
#267054=CARTESIAN_POINT('Ctrl Pts',(-129.934615416877,-5.9628666078469,
539.549090218607));
#267055=CARTESIAN_POINT('',(-129.869812400585,-7.23822414349998,533.035792462989));
#267056=CARTESIAN_POINT('Ctrl Pts',(-129.934615416877,-5.96286660784695,
539.549090218607));
#267057=CARTESIAN_POINT('Ctrl Pts',(-129.895497332176,-6.31987428800097,
539.081130896537));
#267058=CARTESIAN_POINT('Ctrl Pts',(-129.861734938059,-6.6207769123125,
538.572490502143));
#267059=CARTESIAN_POINT('Ctrl Pts',(-129.813111426559,-7.0850070613043,
537.522790181794));
#267060=CARTESIAN_POINT('Ctrl Pts',(-129.797530023073,-7.25319087208481,
536.988354776702));
#267061=CARTESIAN_POINT('Ctrl Pts',(-129.785399163032,-7.4676411379003,
535.892114880487));
#267062=CARTESIAN_POINT('Ctrl Pts',(-129.788874868863,-7.51329980358279,
535.33426240615));
#267063=CARTESIAN_POINT('Ctrl Pts',(-129.814956867898,-7.47911407824396,
534.18773699025));
#267064=CARTESIAN_POINT('Ctrl Pts',(-129.838507736136,-7.39229580420002,
533.603555895973));
#267065=CARTESIAN_POINT('Ctrl Pts',(-129.869812400585,-7.23822414349999,
533.035792462989));
#267066=CARTESIAN_POINT('',(-159.895664541343,-7.20669984090296,532.923108716584));
#267067=CARTESIAN_POINT('Ctrl Pts',(-129.869812400585,-7.23822414349999,
533.035792462989));
#267068=CARTESIAN_POINT('Ctrl Pts',(-134.85921820423,-7.23191213146921,
533.012532315059));
#267069=CARTESIAN_POINT('Ctrl Pts',(-139.895848795771,-7.22618364102021,
532.991856799222));
#267070=CARTESIAN_POINT('Ctrl Pts',(-149.874856564472,-7.21579485641788,
532.954841204099));
#267071=CARTESIAN_POINT('Ctrl Pts',(-154.905389259385,-7.2110430892962,
532.938179552383));
#267072=CARTESIAN_POINT('Ctrl Pts',(-159.895664541343,-7.20669984090297,
532.923108716584));
#267073=CARTESIAN_POINT('Ctrl Pts',(-159.895664541343,-7.20669984090294,
532.923108716584));
#267074=CARTESIAN_POINT('Ctrl Pts',(-159.870103993811,-7.36226817270499,
533.462922370289));
#267075=CARTESIAN_POINT('Ctrl Pts',(-159.850674352115,-7.45675253696417,
534.018685643656));
#267076=CARTESIAN_POINT('Ctrl Pts',(-159.828240589408,-7.51820614028982,
535.114515711267));
#267077=CARTESIAN_POINT('Ctrl Pts',(-159.824566877554,-7.49088360676147,
535.650620761418));
#267078=CARTESIAN_POINT('Ctrl Pts',(-159.832377964382,-7.3225433339189,
536.707849575309));
#267079=CARTESIAN_POINT('Ctrl Pts',(-159.843827611085,-7.18211047599091,
537.225615095904));
#267080=CARTESIAN_POINT('Ctrl Pts',(-159.880789425704,-6.78379176451848,
538.247437378676));
#267081=CARTESIAN_POINT('Ctrl Pts',(-159.906846253054,-6.52166889428979,
538.746052670415));
#267082=CARTESIAN_POINT('Ctrl Pts',(-159.937609420477,-6.20654127333069,
539.210563551645));
#267083=CARTESIAN_POINT('',(-129.869812400585,7.23822414350004,536.964207537012));
#267084=CARTESIAN_POINT('',(-129.934615416877,5.96286660784693,530.450909781393));
#267085=CARTESIAN_POINT('Ctrl Pts',(-129.869812400585,7.23822414350001,
536.964207537012));
#267086=CARTESIAN_POINT('Ctrl Pts',(-129.838465947162,7.39250147631553,
536.395686189782));
#267087=CARTESIAN_POINT('Ctrl Pts',(-129.814894504108,7.47934500364728,
535.810706203688));
#267088=CARTESIAN_POINT('Ctrl Pts',(-129.788829961956,7.51321673970107,
534.662636602979));
#267089=CARTESIAN_POINT('Ctrl Pts',(-129.785389515462,7.4672383479923,534.104054596374));
#267090=CARTESIAN_POINT('Ctrl Pts',(-129.797623339578,7.25211847571004,
533.007946909601));
#267091=CARTESIAN_POINT('Ctrl Pts',(-129.813220504589,7.08391429791342,
532.474308019487));
#267092=CARTESIAN_POINT('Ctrl Pts',(-129.861824504594,6.61997620179486,
531.426155633437));
#267093=CARTESIAN_POINT('Ctrl Pts',(-129.895549481156,6.31939835503053,
530.918245258985));
#267094=CARTESIAN_POINT('Ctrl Pts',(-129.934615416877,5.96286660784708,
530.450909781394));
#267095=CARTESIAN_POINT('',(-159.895664541343,7.20669984090294,537.076891283416));
#267096=CARTESIAN_POINT('Ctrl Pts',(-159.895664541343,7.20669984090292,
537.076891283416));
#267097=CARTESIAN_POINT('Ctrl Pts',(-154.905389418126,7.21104308915801,
537.061820448097));
#267098=CARTESIAN_POINT('Ctrl Pts',(-149.874856854883,7.2157948561274,537.045158796869));
#267099=CARTESIAN_POINT('Ctrl Pts',(-139.895849065273,7.22618364069668,
537.008143201894));
#267100=CARTESIAN_POINT('Ctrl Pts',(-134.859218339044,7.23191213129869,
536.98746768557));
#267101=CARTESIAN_POINT('Ctrl Pts',(-129.869812400585,7.23822414350004,
536.964207537012));
#267102=CARTESIAN_POINT('',(-159.937609420477,6.2065412733309,530.789436448355));
#267103=CARTESIAN_POINT('Ctrl Pts',(-159.937609420477,6.20654127333087,
530.789436448355));
#267104=CARTESIAN_POINT('Ctrl Pts',(-159.906834643176,6.52178782200749,
531.254122633859));
#267105=CARTESIAN_POINT('Ctrl Pts',(-159.880769856038,6.78398922241062,
531.752938404992));
#267106=CARTESIAN_POINT('Ctrl Pts',(-159.843804521963,7.18237209950937,
532.775180680854));
#267107=CARTESIAN_POINT('Ctrl Pts',(-159.832358861788,7.32279367879286,
533.293160677924));
#267108=CARTESIAN_POINT('Ctrl Pts',(-159.824570869009,7.49095925222109,
534.350417431359));
#267109=CARTESIAN_POINT('Ctrl Pts',(-159.82825204698,7.51820444472876,534.8863221477));
#267110=CARTESIAN_POINT('Ctrl Pts',(-159.850688911066,7.45668143260605,
535.981732982314));
#267111=CARTESIAN_POINT('Ctrl Pts',(-159.870113636375,7.36220948547839,
536.537281271198));
#267112=CARTESIAN_POINT('Ctrl Pts',(-159.895664541343,7.20669984090291,
537.076891283416));
#267113=CARTESIAN_POINT('Ctrl Pts',(-129.934615416877,5.96286660784702,
530.450909781394));
#267114=CARTESIAN_POINT('Ctrl Pts',(-134.922636022182,6.01410249000995,
530.51806886512));
#267115=CARTESIAN_POINT('Ctrl Pts',(-139.949152283026,6.05906103332206,
530.579310545017));
#267116=CARTESIAN_POINT('Ctrl Pts',(-149.926082545109,6.13902134883239,
530.691039622605));
#267117=CARTESIAN_POINT('Ctrl Pts',(-154.948459858512,6.17458452265583,
530.742330903078));
#267118=CARTESIAN_POINT('Ctrl Pts',(-159.937609420477,6.20654127333093,
530.789436448355));
#267119=CARTESIAN_POINT('Origin',(0.,0.,695.));
#267120=CARTESIAN_POINT('Origin',(0.,0.,367.5));
#267121=CARTESIAN_POINT('',(15.,-1.83697019872103E-15,695.));
#267122=CARTESIAN_POINT('',(15.,-1.83697019872103E-15,695.));
#267123=CARTESIAN_POINT('',(15.,-1.83697019872103E-15,848.));
#267124=CARTESIAN_POINT('',(15.,-1.83697019872103E-15,695.));
#267125=CARTESIAN_POINT('Origin',(0.,0.,848.));
#267126=CARTESIAN_POINT('Origin',(0.,0.,367.5));
#267127=CARTESIAN_POINT('Ctrl Pts',(-130.,4.30813900827773,697.537703348572));
#267128=CARTESIAN_POINT('Ctrl Pts',(-129.660942106811,14.5393608954781,
695.537703348572));
#267129=CARTESIAN_POINT('Ctrl Pts',(-127.725542856289,24.591579123369,693.537703348572));
#267130=CARTESIAN_POINT('Ctrl Pts',(-125.790143605767,34.6437973512599,
691.537703348572));
#267131=CARTESIAN_POINT('Ctrl Pts',(-122.306058950683,44.269492945671,689.537703348572));
#267132=CARTESIAN_POINT('Ctrl Pts',(-118.821974295598,53.8951885400822,
687.537703348572));
#267133=CARTESIAN_POINT('Ctrl Pts',(-113.874993963172,62.8573449296269,
685.537703348572));
#267134=CARTESIAN_POINT('Ctrl Pts',(-108.928013630747,71.8195013191717,
683.537703348572));
#267135=CARTESIAN_POINT('Ctrl Pts',(-102.639948694852,79.8974404698478,
681.537703348572));
#267136=CARTESIAN_POINT('Ctrl Pts',(-96.3518837589562,87.9753796205239,
679.537703348572));
#267137=CARTESIAN_POINT('Ctrl Pts',(-88.8775672472037,94.9701958612987,
677.537703348572));
#267138=CARTESIAN_POINT('Ctrl Pts',(-81.4032507354512,101.965012102073,
675.537703348572));
#267139=CARTESIAN_POINT('Ctrl Pts',(-72.9267251261952,107.704469842635,
673.537703348572));
#267140=CARTESIAN_POINT('Ctrl Pts',(-64.4501995169392,113.443927583196,
671.537703348572));
#267141=CARTESIAN_POINT('Ctrl Pts',(-55.1801850026552,117.786702325803,
669.537703348572));
#267142=CARTESIAN_POINT('Ctrl Pts',(-45.9101704883713,122.12947706841,667.537703348572));
#267143=CARTESIAN_POINT('Ctrl Pts',(-36.0749255918153,124.968635286057,
665.537703348572));
#267144=CARTESIAN_POINT('Ctrl Pts',(-26.2396806952593,127.807793503704,
663.537703348572));
#267145=CARTESIAN_POINT('Ctrl Pts',(-16.081381787091,129.073425698447,661.537703348572));
#267146=CARTESIAN_POINT('Ctrl Pts',(-5.92308287892268,130.339057893189,
659.537703348572));
#267147=CARTESIAN_POINT('Ctrl Pts',(4.30813900827772,130.,657.537703348572));
#267148=CARTESIAN_POINT('Ctrl Pts',(14.5393608954781,129.660942106811,655.537703348572));
#267149=CARTESIAN_POINT('Ctrl Pts',(24.591579123369,127.725542856289,653.537703348572));
#267150=CARTESIAN_POINT('Ctrl Pts',(34.6437973512599,125.790143605767,651.537703348572));
#267151=CARTESIAN_POINT('Ctrl Pts',(44.269492945671,122.306058950683,649.537703348572));
#267152=CARTESIAN_POINT('Ctrl Pts',(53.8951885400822,118.821974295598,647.537703348572));
#267153=CARTESIAN_POINT('Ctrl Pts',(62.8573449296269,113.874993963172,645.537703348572));
#267154=CARTESIAN_POINT('Ctrl Pts',(71.8195013191717,108.928013630747,643.537703348572));
#267155=CARTESIAN_POINT('Ctrl Pts',(79.8974404698478,102.639948694852,641.537703348572));
#267156=CARTESIAN_POINT('Ctrl Pts',(87.9753796205239,96.3518837589562,639.537703348572));
#267157=CARTESIAN_POINT('Ctrl Pts',(94.9701958612986,88.8775672472037,637.537703348572));
#267158=CARTESIAN_POINT('Ctrl Pts',(101.965012102073,81.4032507354512,635.537703348572));
#267159=CARTESIAN_POINT('Ctrl Pts',(107.704469842635,72.9267251261952,633.537703348572));
#267160=CARTESIAN_POINT('Ctrl Pts',(113.443927583196,64.4501995169392,631.537703348572));
#267161=CARTESIAN_POINT('Ctrl Pts',(117.786702325803,55.1801850026552,629.537703348572));
#267162=CARTESIAN_POINT('Ctrl Pts',(122.12947706841,45.9101704883713,627.537703348572));
#267163=CARTESIAN_POINT('Ctrl Pts',(124.968635286057,36.0749255918153,625.537703348572));
#267164=CARTESIAN_POINT('Ctrl Pts',(127.807793503704,26.2396806952593,623.537703348572));
#267165=CARTESIAN_POINT('Ctrl Pts',(129.073425698447,16.081381787091,621.537703348572));
#267166=CARTESIAN_POINT('Ctrl Pts',(130.339057893189,5.92308287892268,619.537703348572));
#267167=CARTESIAN_POINT('Ctrl Pts',(130.,-4.30813900827772,617.537703348572));
#267168=CARTESIAN_POINT('Ctrl Pts',(129.660942106811,-14.5393608954781,
615.537703348572));
#267169=CARTESIAN_POINT('Ctrl Pts',(127.725542856289,-24.591579123369,613.537703348572));
#267170=CARTESIAN_POINT('Ctrl Pts',(125.790143605767,-34.6437973512599,
611.537703348572));
#267171=CARTESIAN_POINT('Ctrl Pts',(122.306058950683,-44.269492945671,609.537703348572));
#267172=CARTESIAN_POINT('Ctrl Pts',(118.821974295598,-53.8951885400822,
607.537703348572));
#267173=CARTESIAN_POINT('Ctrl Pts',(113.874993963172,-62.8573449296269,
605.537703348572));
#267174=CARTESIAN_POINT('Ctrl Pts',(108.928013630747,-71.8195013191717,
603.537703348572));
#267175=CARTESIAN_POINT('Ctrl Pts',(102.639948694852,-79.8974404698478,
601.537703348572));
#267176=CARTESIAN_POINT('Ctrl Pts',(96.3518837589563,-87.9753796205239,
599.537703348572));
#267177=CARTESIAN_POINT('Ctrl Pts',(88.8775672472037,-94.9701958612986,
597.537703348572));
#267178=CARTESIAN_POINT('Ctrl Pts',(81.4032507354513,-101.965012102073,
595.537703348572));
#267179=CARTESIAN_POINT('Ctrl Pts',(72.9267251261952,-107.704469842635,
593.537703348572));
#267180=CARTESIAN_POINT('Ctrl Pts',(64.4501995169392,-113.443927583196,
591.537703348572));
#267181=CARTESIAN_POINT('Ctrl Pts',(55.1801850026552,-117.786702325803,
589.537703348572));
#267182=CARTESIAN_POINT('Ctrl Pts',(45.9101704883713,-122.12947706841,587.537703348572));
#267183=CARTESIAN_POINT('Ctrl Pts',(36.0749255918153,-124.968635286057,
585.537703348572));
#267184=CARTESIAN_POINT('Ctrl Pts',(26.2396806952593,-127.807793503704,
583.537703348572));
#267185=CARTESIAN_POINT('Ctrl Pts',(16.081381787091,-129.073425698447,581.537703348572));
#267186=CARTESIAN_POINT('Ctrl Pts',(5.92308287892275,-130.339057893189,
579.537703348572));
#267187=CARTESIAN_POINT('Ctrl Pts',(-4.30813900827771,-130.,577.537703348572));
#267188=CARTESIAN_POINT('Ctrl Pts',(-14.5393608954782,-129.660942106811,
575.537703348572));
#267189=CARTESIAN_POINT('Ctrl Pts',(-24.591579123369,-127.725542856289,
573.537703348572));
#267190=CARTESIAN_POINT('Ctrl Pts',(-34.6437973512598,-125.790143605767,
571.537703348572));
#267191=CARTESIAN_POINT('Ctrl Pts',(-44.269492945671,-122.306058950683,
569.537703348572));
#267192=CARTESIAN_POINT('Ctrl Pts',(-53.8951885400822,-118.821974295598,
567.537703348572));
#267193=CARTESIAN_POINT('Ctrl Pts',(-62.8573449296269,-113.874993963172,
565.537703348572));
#267194=CARTESIAN_POINT('Ctrl Pts',(-71.8195013191717,-108.928013630747,
563.537703348572));
#267195=CARTESIAN_POINT('Ctrl Pts',(-79.8974404698478,-102.639948694852,
561.537703348572));
#267196=CARTESIAN_POINT('Ctrl Pts',(-87.975379620524,-96.3518837589562,
559.537703348572));
#267197=CARTESIAN_POINT('Ctrl Pts',(-94.9701958612986,-88.8775672472037,
557.537703348572));
#267198=CARTESIAN_POINT('Ctrl Pts',(-101.965012102073,-81.4032507354513,
555.537703348572));
#267199=CARTESIAN_POINT('Ctrl Pts',(-107.704469842635,-72.9267251261952,
553.537703348572));
#267200=CARTESIAN_POINT('Ctrl Pts',(-113.443927583196,-64.4501995169392,
551.537703348572));
#267201=CARTESIAN_POINT('Ctrl Pts',(-117.786702325803,-55.1801850026553,
549.537703348572));
#267202=CARTESIAN_POINT('Ctrl Pts',(-122.12947706841,-45.9101704883713,
547.537703348572));
#267203=CARTESIAN_POINT('Ctrl Pts',(-124.968635286057,-36.0749255918153,
545.537703348572));
#267204=CARTESIAN_POINT('Ctrl Pts',(-127.807793503704,-26.2396806952593,
543.537703348572));
#267205=CARTESIAN_POINT('Ctrl Pts',(-129.073425698447,-16.081381787091,
541.537703348572));
#267206=CARTESIAN_POINT('Ctrl Pts',(-130.339057893189,-5.92308287892275,
539.537703348572));
#267207=CARTESIAN_POINT('Ctrl Pts',(-130.,4.30813900827773,537.537703348572));
#267208=CARTESIAN_POINT('Ctrl Pts',(-130.,-4.30813900827845,692.462296651428));
#267209=CARTESIAN_POINT('Ctrl Pts',(-130.339057893189,5.92308287892195,
690.462296651428));
#267210=CARTESIAN_POINT('Ctrl Pts',(-129.073425698447,16.0813817870903,
688.462296651428));
#267211=CARTESIAN_POINT('Ctrl Pts',(-127.807793503705,26.2396806952586,
686.462296651429));
#267212=CARTESIAN_POINT('Ctrl Pts',(-124.968635286058,36.0749255918146,
684.462296651428));
#267213=CARTESIAN_POINT('Ctrl Pts',(-122.129477068411,45.9101704883706,
682.462296651429));
#267214=CARTESIAN_POINT('Ctrl Pts',(-117.786702325804,55.1801850026546,
680.462296651428));
#267215=CARTESIAN_POINT('Ctrl Pts',(-113.443927583196,64.4501995169386,
678.462296651428));
#267216=CARTESIAN_POINT('Ctrl Pts',(-107.704469842635,72.9267251261946,
676.462296651429));
#267217=CARTESIAN_POINT('Ctrl Pts',(-101.965012102074,81.4032507354507,
674.462296651429));
#267218=CARTESIAN_POINT('Ctrl Pts',(-94.9701958612992,88.8775672472032,
672.462296651428));
#267219=CARTESIAN_POINT('Ctrl Pts',(-87.9753796205245,96.3518837589558,
670.462296651429));
#267220=CARTESIAN_POINT('Ctrl Pts',(-79.8974404698484,102.639948694851,
668.462296651428));
#267221=CARTESIAN_POINT('Ctrl Pts',(-71.8195013191724,108.928013630747,
666.462296651428));
#267222=CARTESIAN_POINT('Ctrl Pts',(-62.8573449296276,113.874993963172,
664.462296651428));
#267223=CARTESIAN_POINT('Ctrl Pts',(-53.8951885400828,118.821974295598,
662.462296651429));
#267224=CARTESIAN_POINT('Ctrl Pts',(-44.2694929456717,122.306058950682,
660.462296651428));
#267225=CARTESIAN_POINT('Ctrl Pts',(-34.6437973512606,125.790143605767,
658.462296651428));
#267226=CARTESIAN_POINT('Ctrl Pts',(-24.5915791233697,127.725542856289,
656.462296651429));
#267227=CARTESIAN_POINT('Ctrl Pts',(-14.5393608954789,129.660942106811,
654.462296651428));
#267228=CARTESIAN_POINT('Ctrl Pts',(-4.30813900827846,130.,652.462296651428));
#267229=CARTESIAN_POINT('Ctrl Pts',(5.92308287892194,130.339057893189,650.462296651429));
#267230=CARTESIAN_POINT('Ctrl Pts',(16.0813817870903,129.073425698447,648.462296651428));
#267231=CARTESIAN_POINT('Ctrl Pts',(26.2396806952586,127.807793503705,646.462296651428));
#267232=CARTESIAN_POINT('Ctrl Pts',(36.0749255918146,124.968635286058,644.462296651428));
#267233=CARTESIAN_POINT('Ctrl Pts',(45.9101704883706,122.129477068411,642.462296651428));
#267234=CARTESIAN_POINT('Ctrl Pts',(55.1801850026546,117.786702325804,640.462296651428));
#267235=CARTESIAN_POINT('Ctrl Pts',(64.4501995169386,113.443927583196,638.462296651429));
#267236=CARTESIAN_POINT('Ctrl Pts',(72.9267251261946,107.704469842635,636.462296651428));
#267237=CARTESIAN_POINT('Ctrl Pts',(81.4032507354506,101.965012102074,634.462296651428));
#267238=CARTESIAN_POINT('Ctrl Pts',(88.8775672472032,94.9701958612992,632.462296651428));
#267239=CARTESIAN_POINT('Ctrl Pts',(96.3518837589558,87.9753796205245,630.462296651428));
#267240=CARTESIAN_POINT('Ctrl Pts',(102.639948694851,79.8974404698484,628.462296651428));
#267241=CARTESIAN_POINT('Ctrl Pts',(108.928013630747,71.8195013191724,626.462296651429));
#267242=CARTESIAN_POINT('Ctrl Pts',(113.874993963172,62.8573449296276,624.462296651428));
#267243=CARTESIAN_POINT('Ctrl Pts',(118.821974295598,53.8951885400829,622.462296651428));
#267244=CARTESIAN_POINT('Ctrl Pts',(122.306058950682,44.2694929456717,620.462296651428));
#267245=CARTESIAN_POINT('Ctrl Pts',(125.790143605767,34.6437973512606,618.462296651428));
#267246=CARTESIAN_POINT('Ctrl Pts',(127.725542856289,24.5915791233698,616.462296651428));
#267247=CARTESIAN_POINT('Ctrl Pts',(129.660942106811,14.5393608954789,614.462296651429));
#267248=CARTESIAN_POINT('Ctrl Pts',(130.,4.30813900827846,612.462296651428));
#267249=CARTESIAN_POINT('Ctrl Pts',(130.339057893189,-5.92308287892194,
610.462296651428));
#267250=CARTESIAN_POINT('Ctrl Pts',(129.073425698447,-16.0813817870903,
608.462296651428));
#267251=CARTESIAN_POINT('Ctrl Pts',(127.807793503705,-26.2396806952586,
606.462296651428));
#267252=CARTESIAN_POINT('Ctrl Pts',(124.968635286058,-36.0749255918146,
604.462296651428));
#267253=CARTESIAN_POINT('Ctrl Pts',(122.129477068411,-45.9101704883706,
602.462296651429));
#267254=CARTESIAN_POINT('Ctrl Pts',(117.786702325804,-55.1801850026546,
600.462296651428));
#267255=CARTESIAN_POINT('Ctrl Pts',(113.443927583196,-64.4501995169386,
598.462296651428));
#267256=CARTESIAN_POINT('Ctrl Pts',(107.704469842635,-72.9267251261946,
596.462296651428));
#267257=CARTESIAN_POINT('Ctrl Pts',(101.965012102074,-81.4032507354506,
594.462296651428));
#267258=CARTESIAN_POINT('Ctrl Pts',(94.9701958612992,-88.8775672472032,
592.462296651428));
#267259=CARTESIAN_POINT('Ctrl Pts',(87.9753796205246,-96.3518837589557,
590.462296651429));
#267260=CARTESIAN_POINT('Ctrl Pts',(79.8974404698484,-102.639948694851,
588.462296651428));
#267261=CARTESIAN_POINT('Ctrl Pts',(71.8195013191723,-108.928013630747,
586.462296651428));
#267262=CARTESIAN_POINT('Ctrl Pts',(62.8573449296276,-113.874993963172,
584.462296651428));
#267263=CARTESIAN_POINT('Ctrl Pts',(53.8951885400829,-118.821974295598,
582.462296651428));
#267264=CARTESIAN_POINT('Ctrl Pts',(44.2694929456717,-122.306058950682,
580.462296651428));
#267265=CARTESIAN_POINT('Ctrl Pts',(34.6437973512606,-125.790143605767,
578.462296651429));
#267266=CARTESIAN_POINT('Ctrl Pts',(24.5915791233698,-127.725542856289,
576.462296651428));
#267267=CARTESIAN_POINT('Ctrl Pts',(14.5393608954789,-129.660942106811,
574.462296651428));
#267268=CARTESIAN_POINT('Ctrl Pts',(4.30813900827847,-130.,572.462296651428));
#267269=CARTESIAN_POINT('Ctrl Pts',(-5.92308287892199,-130.339057893189,
570.462296651428));
#267270=CARTESIAN_POINT('Ctrl Pts',(-16.0813817870903,-129.073425698447,
568.462296651428));
#267271=CARTESIAN_POINT('Ctrl Pts',(-26.2396806952585,-127.807793503705,
566.462296651429));
#267272=CARTESIAN_POINT('Ctrl Pts',(-36.0749255918146,-124.968635286058,
564.462296651428));
#267273=CARTESIAN_POINT('Ctrl Pts',(-45.9101704883706,-122.129477068411,
562.462296651428));
#267274=CARTESIAN_POINT('Ctrl Pts',(-55.1801850026546,-117.786702325804,
560.462296651428));
#267275=CARTESIAN_POINT('Ctrl Pts',(-64.4501995169385,-113.443927583197,
558.462296651429));
#267276=CARTESIAN_POINT('Ctrl Pts',(-72.9267251261946,-107.704469842635,
556.462296651428));
#267277=CARTESIAN_POINT('Ctrl Pts',(-81.4032507354507,-101.965012102074,
554.462296651429));
#267278=CARTESIAN_POINT('Ctrl Pts',(-88.8775672472032,-94.9701958612992,
552.462296651428));
#267279=CARTESIAN_POINT('Ctrl Pts',(-96.3518837589557,-87.9753796205246,
550.462296651428));
#267280=CARTESIAN_POINT('Ctrl Pts',(-102.639948694851,-79.8974404698484,
548.462296651428));
#267281=CARTESIAN_POINT('Ctrl Pts',(-108.928013630747,-71.8195013191723,
546.462296651429));
#267282=CARTESIAN_POINT('Ctrl Pts',(-113.874993963172,-62.8573449296276,
544.462296651428));
#267283=CARTESIAN_POINT('Ctrl Pts',(-118.821974295598,-53.8951885400829,
542.462296651429));
#267284=CARTESIAN_POINT('Ctrl Pts',(-122.306058950682,-44.2694929456718,
540.462296651428));
#267285=CARTESIAN_POINT('Ctrl Pts',(-125.790143605767,-34.6437973512606,
538.462296651428));
#267286=CARTESIAN_POINT('Ctrl Pts',(-127.725542856289,-24.5915791233698,
536.462296651428));
#267287=CARTESIAN_POINT('Ctrl Pts',(-129.660942106811,-14.5393608954789,
534.462296651429));
#267288=CARTESIAN_POINT('Ctrl Pts',(-130.,-4.30813900827845,532.462296651428));
#267289=CARTESIAN_POINT('Ctrl Pts',(-129.934615416877,5.96286660784587,
690.450909781394));
#267290=CARTESIAN_POINT('Ctrl Pts',(-129.701667605591,11.038945994198,689.455068342531));
#267291=CARTESIAN_POINT('Ctrl Pts',(-129.073425698447,16.0813817870903,
688.462296651428));
#267292=CARTESIAN_POINT('Ctrl Pts',(-127.807793503705,26.2396806952586,
686.462296651429));
#267293=CARTESIAN_POINT('Ctrl Pts',(-124.968635286058,36.0749255918146,
684.462296651428));
#267294=CARTESIAN_POINT('Ctrl Pts',(-122.129477068411,45.9101704883706,
682.462296651429));
#267295=CARTESIAN_POINT('Ctrl Pts',(-117.786702325804,55.1801850026546,
680.462296651428));
#267296=CARTESIAN_POINT('Ctrl Pts',(-113.443927583196,64.4501995169386,
678.462296651428));
#267297=CARTESIAN_POINT('Ctrl Pts',(-107.704469842635,72.9267251261946,
676.462296651429));
#267298=CARTESIAN_POINT('Ctrl Pts',(-101.965012102074,81.4032507354507,
674.462296651429));
#267299=CARTESIAN_POINT('Ctrl Pts',(-94.9701958612992,88.8775672472032,
672.462296651428));
#267300=CARTESIAN_POINT('Ctrl Pts',(-87.9753796205245,96.3518837589558,
670.462296651429));
#267301=CARTESIAN_POINT('Ctrl Pts',(-79.8974404698484,102.639948694851,
668.462296651428));
#267302=CARTESIAN_POINT('Ctrl Pts',(-71.8195013191724,108.928013630747,
666.462296651429));
#267303=CARTESIAN_POINT('Ctrl Pts',(-62.8573449296276,113.874993963172,
664.462296651428));
#267304=CARTESIAN_POINT('Ctrl Pts',(-53.8951885400828,118.821974295598,
662.462296651429));
#267305=CARTESIAN_POINT('Ctrl Pts',(-44.2694929456717,122.306058950682,
660.462296651428));
#267306=CARTESIAN_POINT('Ctrl Pts',(-34.6437973512606,125.790143605767,
658.462296651429));
#267307=CARTESIAN_POINT('Ctrl Pts',(-24.5915791233697,127.725542856289,
656.462296651429));
#267308=CARTESIAN_POINT('Ctrl Pts',(-14.5393608954789,129.660942106811,
654.462296651428));
#267309=CARTESIAN_POINT('Ctrl Pts',(-4.30813900827846,130.,652.462296651428));
#267310=CARTESIAN_POINT('Ctrl Pts',(5.92308287892194,130.339057893189,650.462296651429));
#267311=CARTESIAN_POINT('Ctrl Pts',(16.0813817870903,129.073425698447,648.462296651428));
#267312=CARTESIAN_POINT('Ctrl Pts',(26.2396806952586,127.807793503705,646.462296651429));
#267313=CARTESIAN_POINT('Ctrl Pts',(36.0749255918146,124.968635286058,644.462296651428));
#267314=CARTESIAN_POINT('Ctrl Pts',(45.9101704883706,122.129477068411,642.462296651428));
#267315=CARTESIAN_POINT('Ctrl Pts',(55.1801850026546,117.786702325804,640.462296651428));
#267316=CARTESIAN_POINT('Ctrl Pts',(64.4501995169386,113.443927583196,638.462296651428));
#267317=CARTESIAN_POINT('Ctrl Pts',(72.9267251261946,107.704469842635,636.462296651428));
#267318=CARTESIAN_POINT('Ctrl Pts',(81.4032507354506,101.965012102074,634.462296651428));
#267319=CARTESIAN_POINT('Ctrl Pts',(88.8775672472032,94.9701958612992,632.462296651428));
#267320=CARTESIAN_POINT('Ctrl Pts',(96.3518837589558,87.9753796205245,630.462296651428));
#267321=CARTESIAN_POINT('Ctrl Pts',(102.639948694851,79.8974404698484,628.462296651428));
#267322=CARTESIAN_POINT('Ctrl Pts',(108.928013630747,71.8195013191724,626.462296651428));
#267323=CARTESIAN_POINT('Ctrl Pts',(113.874993963172,62.8573449296276,624.462296651428));
#267324=CARTESIAN_POINT('Ctrl Pts',(118.821974295598,53.8951885400829,622.462296651428));
#267325=CARTESIAN_POINT('Ctrl Pts',(122.306058950682,44.2694929456717,620.462296651428));
#267326=CARTESIAN_POINT('Ctrl Pts',(125.790143605767,34.6437973512606,618.462296651428));
#267327=CARTESIAN_POINT('Ctrl Pts',(127.725542856289,24.5915791233698,616.462296651428));
#267328=CARTESIAN_POINT('Ctrl Pts',(129.660942106811,14.5393608954789,614.462296651429));
#267329=CARTESIAN_POINT('Ctrl Pts',(130.,4.30813900827846,612.462296651428));
#267330=CARTESIAN_POINT('Ctrl Pts',(130.339057893189,-5.92308287892194,
610.462296651428));
#267331=CARTESIAN_POINT('Ctrl Pts',(129.073425698447,-16.0813817870903,
608.462296651428));
#267332=CARTESIAN_POINT('Ctrl Pts',(127.807793503705,-26.2396806952586,
606.462296651428));
#267333=CARTESIAN_POINT('Ctrl Pts',(124.968635286058,-36.0749255918146,
604.462296651428));
#267334=CARTESIAN_POINT('Ctrl Pts',(122.129477068411,-45.9101704883706,
602.462296651429));
#267335=CARTESIAN_POINT('Ctrl Pts',(117.786702325804,-55.1801850026546,
600.462296651428));
#267336=CARTESIAN_POINT('Ctrl Pts',(113.443927583196,-64.4501995169386,
598.462296651428));
#267337=CARTESIAN_POINT('Ctrl Pts',(107.704469842635,-72.9267251261946,
596.462296651428));
#267338=CARTESIAN_POINT('Ctrl Pts',(101.965012102074,-81.4032507354506,
594.462296651428));
#267339=CARTESIAN_POINT('Ctrl Pts',(94.9701958612992,-88.8775672472032,
592.462296651428));
#267340=CARTESIAN_POINT('Ctrl Pts',(87.9753796205245,-96.3518837589557,
590.462296651429));
#267341=CARTESIAN_POINT('Ctrl Pts',(79.8974404698484,-102.639948694851,
588.462296651428));
#267342=CARTESIAN_POINT('Ctrl Pts',(71.8195013191723,-108.928013630747,
586.462296651428));
#267343=CARTESIAN_POINT('Ctrl Pts',(62.8573449296276,-113.874993963172,
584.462296651428));
#267344=CARTESIAN_POINT('Ctrl Pts',(53.8951885400829,-118.821974295598,
582.462296651428));
#267345=CARTESIAN_POINT('Ctrl Pts',(44.2694929456717,-122.306058950682,
580.462296651428));
#267346=CARTESIAN_POINT('Ctrl Pts',(34.6437973512606,-125.790143605767,
578.462296651429));
#267347=CARTESIAN_POINT('Ctrl Pts',(24.5915791233698,-127.725542856289,
576.462296651428));
#267348=CARTESIAN_POINT('Ctrl Pts',(14.5393608954789,-129.660942106811,
574.462296651428));
#267349=CARTESIAN_POINT('Ctrl Pts',(4.30813900827847,-130.,572.462296651428));
#267350=CARTESIAN_POINT('Ctrl Pts',(-5.92308287892199,-130.339057893189,
570.462296651428));
#267351=CARTESIAN_POINT('Ctrl Pts',(-16.0813817870903,-129.073425698447,
568.462296651428));
#267352=CARTESIAN_POINT('Ctrl Pts',(-26.2396806952585,-127.807793503705,
566.462296651429));
#267353=CARTESIAN_POINT('Ctrl Pts',(-36.0749255918146,-124.968635286058,
564.462296651428));
#267354=CARTESIAN_POINT('Ctrl Pts',(-45.9101704883706,-122.129477068411,
562.462296651428));
#267355=CARTESIAN_POINT('Ctrl Pts',(-55.1801850026546,-117.786702325804,
560.462296651428));
#267356=CARTESIAN_POINT('Ctrl Pts',(-64.4501995169385,-113.443927583197,
558.462296651429));
#267357=CARTESIAN_POINT('Ctrl Pts',(-72.9267251261946,-107.704469842635,
556.462296651428));
#267358=CARTESIAN_POINT('Ctrl Pts',(-81.4032507354507,-101.965012102074,
554.462296651429));
#267359=CARTESIAN_POINT('Ctrl Pts',(-88.8775672472032,-94.9701958612992,
552.462296651428));
#267360=CARTESIAN_POINT('Ctrl Pts',(-96.3518837589557,-87.9753796205245,
550.462296651428));
#267361=CARTESIAN_POINT('Ctrl Pts',(-102.639948694851,-79.8974404698484,
548.462296651428));
#267362=CARTESIAN_POINT('Ctrl Pts',(-108.928013630747,-71.8195013191723,
546.462296651429));
#267363=CARTESIAN_POINT('Ctrl Pts',(-113.874993963172,-62.8573449296276,
544.462296651428));
#267364=CARTESIAN_POINT('Ctrl Pts',(-118.821974295598,-53.8951885400829,
542.462296651429));
#267365=CARTESIAN_POINT('Ctrl Pts',(-122.306058950682,-44.2694929456718,
540.462296651428));
#267366=CARTESIAN_POINT('Ctrl Pts',(-125.790143605767,-34.6437973512606,
538.462296651428));
#267367=CARTESIAN_POINT('Ctrl Pts',(-127.725542856289,-24.5915791233698,
536.462296651428));
#267368=CARTESIAN_POINT('Ctrl Pts',(-129.382196958681,-15.9871278397995,
534.750345898172));
#267369=CARTESIAN_POINT('Ctrl Pts',(-129.869812400585,-7.23822414349998,
533.035792462989));
#267370=CARTESIAN_POINT('Ctrl Pts',(-129.869812400585,7.23822414349888,
696.964207537012));
#267371=CARTESIAN_POINT('Ctrl Pts',(-129.382196958681,15.9871278397986,
695.249654101829));
#267372=CARTESIAN_POINT('Ctrl Pts',(-127.725542856289,24.591579123369,693.537703348572));
#267373=CARTESIAN_POINT('Ctrl Pts',(-125.790143605767,34.6437973512599,
691.537703348572));
#267374=CARTESIAN_POINT('Ctrl Pts',(-122.306058950683,44.269492945671,689.537703348572));
#267375=CARTESIAN_POINT('Ctrl Pts',(-118.821974295598,53.8951885400822,
687.537703348572));
#267376=CARTESIAN_POINT('Ctrl Pts',(-113.874993963172,62.8573449296269,
685.537703348572));
#267377=CARTESIAN_POINT('Ctrl Pts',(-108.928013630747,71.8195013191717,
683.537703348572));
#267378=CARTESIAN_POINT('Ctrl Pts',(-102.639948694852,79.8974404698478,
681.537703348572));
#267379=CARTESIAN_POINT('Ctrl Pts',(-96.3518837589562,87.9753796205239,
679.537703348572));
#267380=CARTESIAN_POINT('Ctrl Pts',(-88.8775672472037,94.9701958612987,
677.537703348572));
#267381=CARTESIAN_POINT('Ctrl Pts',(-81.4032507354512,101.965012102073,
675.537703348572));
#267382=CARTESIAN_POINT('Ctrl Pts',(-72.9267251261952,107.704469842635,
673.537703348572));
#267383=CARTESIAN_POINT('Ctrl Pts',(-64.4501995169392,113.443927583196,
671.537703348572));
#267384=CARTESIAN_POINT('Ctrl Pts',(-55.1801850026552,117.786702325803,
669.537703348572));
#267385=CARTESIAN_POINT('Ctrl Pts',(-45.9101704883713,122.12947706841,667.537703348572));
#267386=CARTESIAN_POINT('Ctrl Pts',(-36.0749255918153,124.968635286057,
665.537703348572));
#267387=CARTESIAN_POINT('Ctrl Pts',(-26.2396806952593,127.807793503704,
663.537703348572));
#267388=CARTESIAN_POINT('Ctrl Pts',(-16.081381787091,129.073425698447,661.537703348572));
#267389=CARTESIAN_POINT('Ctrl Pts',(-5.92308287892268,130.339057893189,
659.537703348572));
#267390=CARTESIAN_POINT('Ctrl Pts',(4.30813900827772,130.,657.537703348572));
#267391=CARTESIAN_POINT('Ctrl Pts',(14.5393608954781,129.660942106811,655.537703348572));
#267392=CARTESIAN_POINT('Ctrl Pts',(24.591579123369,127.725542856289,653.537703348572));
#267393=CARTESIAN_POINT('Ctrl Pts',(34.6437973512599,125.790143605767,651.537703348572));
#267394=CARTESIAN_POINT('Ctrl Pts',(44.269492945671,122.306058950683,649.537703348572));
#267395=CARTESIAN_POINT('Ctrl Pts',(53.8951885400822,118.821974295598,647.537703348572));
#267396=CARTESIAN_POINT('Ctrl Pts',(62.8573449296269,113.874993963172,645.537703348572));
#267397=CARTESIAN_POINT('Ctrl Pts',(71.8195013191717,108.928013630747,643.537703348572));
#267398=CARTESIAN_POINT('Ctrl Pts',(79.8974404698478,102.639948694852,641.537703348572));
#267399=CARTESIAN_POINT('Ctrl Pts',(87.9753796205239,96.3518837589562,639.537703348572));
#267400=CARTESIAN_POINT('Ctrl Pts',(94.9701958612986,88.8775672472037,637.537703348572));
#267401=CARTESIAN_POINT('Ctrl Pts',(101.965012102073,81.4032507354512,635.537703348572));
#267402=CARTESIAN_POINT('Ctrl Pts',(107.704469842635,72.9267251261952,633.537703348572));
#267403=CARTESIAN_POINT('Ctrl Pts',(113.443927583196,64.4501995169392,631.537703348572));
#267404=CARTESIAN_POINT('Ctrl Pts',(117.786702325803,55.1801850026552,629.537703348572));
#267405=CARTESIAN_POINT('Ctrl Pts',(122.12947706841,45.9101704883713,627.537703348572));
#267406=CARTESIAN_POINT('Ctrl Pts',(124.968635286057,36.0749255918153,625.537703348572));
#267407=CARTESIAN_POINT('Ctrl Pts',(127.807793503704,26.2396806952593,623.537703348572));
#267408=CARTESIAN_POINT('Ctrl Pts',(129.073425698447,16.081381787091,621.537703348572));
#267409=CARTESIAN_POINT('Ctrl Pts',(130.339057893189,5.92308287892268,619.537703348572));
#267410=CARTESIAN_POINT('Ctrl Pts',(130.,-4.30813900827772,617.537703348572));
#267411=CARTESIAN_POINT('Ctrl Pts',(129.660942106811,-14.5393608954781,
615.537703348572));
#267412=CARTESIAN_POINT('Ctrl Pts',(127.725542856289,-24.591579123369,613.537703348572));
#267413=CARTESIAN_POINT('Ctrl Pts',(125.790143605767,-34.6437973512599,
611.537703348572));
#267414=CARTESIAN_POINT('Ctrl Pts',(122.306058950683,-44.269492945671,609.537703348572));
#267415=CARTESIAN_POINT('Ctrl Pts',(118.821974295598,-53.8951885400822,
607.537703348572));
#267416=CARTESIAN_POINT('Ctrl Pts',(113.874993963172,-62.8573449296269,
605.537703348572));
#267417=CARTESIAN_POINT('Ctrl Pts',(108.928013630747,-71.8195013191717,
603.537703348572));
#267418=CARTESIAN_POINT('Ctrl Pts',(102.639948694852,-79.8974404698478,
601.537703348572));
#267419=CARTESIAN_POINT('Ctrl Pts',(96.3518837589563,-87.9753796205239,
599.537703348572));
#267420=CARTESIAN_POINT('Ctrl Pts',(88.8775672472037,-94.9701958612986,
597.537703348572));
#267421=CARTESIAN_POINT('Ctrl Pts',(81.4032507354513,-101.965012102073,
595.537703348572));
#267422=CARTESIAN_POINT('Ctrl Pts',(72.9267251261952,-107.704469842635,
593.537703348572));
#267423=CARTESIAN_POINT('Ctrl Pts',(64.4501995169392,-113.443927583196,
591.537703348572));
#267424=CARTESIAN_POINT('Ctrl Pts',(55.1801850026552,-117.786702325803,
589.537703348572));
#267425=CARTESIAN_POINT('Ctrl Pts',(45.9101704883713,-122.12947706841,587.537703348572));
#267426=CARTESIAN_POINT('Ctrl Pts',(36.0749255918153,-124.968635286057,
585.537703348572));
#267427=CARTESIAN_POINT('Ctrl Pts',(26.2396806952593,-127.807793503704,
583.537703348572));
#267428=CARTESIAN_POINT('Ctrl Pts',(16.081381787091,-129.073425698447,581.537703348572));
#267429=CARTESIAN_POINT('Ctrl Pts',(5.92308287892275,-130.339057893189,
579.537703348572));
#267430=CARTESIAN_POINT('Ctrl Pts',(-4.30813900827771,-130.,577.537703348572));
#267431=CARTESIAN_POINT('Ctrl Pts',(-14.5393608954782,-129.660942106811,
575.537703348572));
#267432=CARTESIAN_POINT('Ctrl Pts',(-24.591579123369,-127.725542856289,
573.537703348572));
#267433=CARTESIAN_POINT('Ctrl Pts',(-34.6437973512598,-125.790143605767,
571.537703348572));
#267434=CARTESIAN_POINT('Ctrl Pts',(-44.269492945671,-122.306058950683,
569.537703348572));
#267435=CARTESIAN_POINT('Ctrl Pts',(-53.8951885400822,-118.821974295598,
567.537703348572));
#267436=CARTESIAN_POINT('Ctrl Pts',(-62.8573449296269,-113.874993963172,
565.537703348572));
#267437=CARTESIAN_POINT('Ctrl Pts',(-71.8195013191717,-108.928013630747,
563.537703348572));
#267438=CARTESIAN_POINT('Ctrl Pts',(-79.8974404698478,-102.639948694852,
561.537703348572));
#267439=CARTESIAN_POINT('Ctrl Pts',(-87.975379620524,-96.3518837589562,
559.537703348572));
#267440=CARTESIAN_POINT('Ctrl Pts',(-94.9701958612986,-88.8775672472037,
557.537703348572));
#267441=CARTESIAN_POINT('Ctrl Pts',(-101.965012102073,-81.4032507354513,
555.537703348572));
#267442=CARTESIAN_POINT('Ctrl Pts',(-107.704469842635,-72.9267251261952,
553.537703348572));
#267443=CARTESIAN_POINT('Ctrl Pts',(-113.443927583196,-64.4501995169392,
551.537703348572));
#267444=CARTESIAN_POINT('Ctrl Pts',(-117.786702325803,-55.1801850026553,
549.537703348572));
#267445=CARTESIAN_POINT('Ctrl Pts',(-122.12947706841,-45.9101704883713,
547.537703348572));
#267446=CARTESIAN_POINT('Ctrl Pts',(-124.968635286057,-36.0749255918153,
545.537703348572));
#267447=CARTESIAN_POINT('Ctrl Pts',(-127.807793503704,-26.2396806952593,
543.537703348572));
#267448=CARTESIAN_POINT('Ctrl Pts',(-129.073425698447,-16.081381787091,
541.537703348572));
#267449=CARTESIAN_POINT('Ctrl Pts',(-129.701667605591,-11.038945994199,
540.54493165747));
#267450=CARTESIAN_POINT('Ctrl Pts',(-129.934615416877,-5.96286660784691,
539.549090218607));
#267451=CARTESIAN_POINT('Ctrl Pts',(-160.,4.30813900827767,697.537703348572));
#267452=CARTESIAN_POINT('Ctrl Pts',(-159.660942106811,16.9004121002166,
695.537703348572));
#267453=CARTESIAN_POINT('Ctrl Pts',(-157.356193074143,29.2846130745759,
693.537703348572));
#267454=CARTESIAN_POINT('Ctrl Pts',(-155.051444041476,41.6688140489352,
691.537703348572));
#267455=CARTESIAN_POINT('Ctrl Pts',(-150.837754439537,53.5400027769194,
689.537703348572));
#267456=CARTESIAN_POINT('Ctrl Pts',(-146.624064837599,65.4111915049037,
687.537703348572));
#267457=CARTESIAN_POINT('Ctrl Pts',(-140.605189688823,76.4770599218133,
685.537703348572));
#267458=CARTESIAN_POINT('Ctrl Pts',(-134.586314540048,87.542928338723,683.537703348572));
#267459=CARTESIAN_POINT('Ctrl Pts',(-126.9104585261,97.530998038622,681.537703348572));
#267460=CARTESIAN_POINT('Ctrl Pts',(-119.234602512152,107.519067738521,
679.537703348572));
#267461=CARTESIAN_POINT('Ctrl Pts',(-110.0907706828,116.183399296895,677.537703348572));
#267462=CARTESIAN_POINT('Ctrl Pts',(-100.946938853448,124.847730855269,
675.537703348572));
#267463=CARTESIAN_POINT('Ctrl Pts',(-90.5602826949695,131.974979673883,
673.537703348572));
#267464=CARTESIAN_POINT('Ctrl Pts',(-80.1736265364906,139.102228492497,
671.537703348572));
#267465=CARTESIAN_POINT('Ctrl Pts',(-68.7998999948417,144.516898051454,
669.537703348572));
#267466=CARTESIAN_POINT('Ctrl Pts',(-57.4261734531929,149.931567610411,
667.537703348572));
#267467=CARTESIAN_POINT('Ctrl Pts',(-45.3454354230638,153.500330774912,
665.537703348572));
#267468=CARTESIAN_POINT('Ctrl Pts',(-33.2646973929347,157.069093939413,
663.537703348572));
#267469=CARTESIAN_POINT('Ctrl Pts',(-20.774415738298,158.704075916301,661.537703348572));
#267470=CARTESIAN_POINT('Ctrl Pts',(-8.28413408366129,160.339057893189,
659.537703348572));
#267471=CARTESIAN_POINT('Ctrl Pts',(4.30813900827766,160.,657.537703348572));
#267472=CARTESIAN_POINT('Ctrl Pts',(16.9004121002166,159.660942106811,655.537703348572));
#267473=CARTESIAN_POINT('Ctrl Pts',(29.2846130745759,157.356193074143,653.537703348572));
#267474=CARTESIAN_POINT('Ctrl Pts',(41.6688140489352,155.051444041476,651.537703348572));
#267475=CARTESIAN_POINT('Ctrl Pts',(53.5400027769194,150.837754439537,649.537703348572));
#267476=CARTESIAN_POINT('Ctrl Pts',(65.4111915049037,146.624064837599,647.537703348572));
#267477=CARTESIAN_POINT('Ctrl Pts',(76.4770599218133,140.605189688823,645.537703348572));
#267478=CARTESIAN_POINT('Ctrl Pts',(87.542928338723,134.586314540048,643.537703348572));
#267479=CARTESIAN_POINT('Ctrl Pts',(97.530998038622,126.9104585261,641.537703348572));
#267480=CARTESIAN_POINT('Ctrl Pts',(107.519067738521,119.234602512152,639.537703348572));
#267481=CARTESIAN_POINT('Ctrl Pts',(116.183399296895,110.0907706828,637.537703348572));
#267482=CARTESIAN_POINT('Ctrl Pts',(124.847730855269,100.946938853448,635.537703348572));
#267483=CARTESIAN_POINT('Ctrl Pts',(131.974979673883,90.5602826949695,633.537703348572));
#267484=CARTESIAN_POINT('Ctrl Pts',(139.102228492497,80.1736265364906,631.537703348572));
#267485=CARTESIAN_POINT('Ctrl Pts',(144.516898051454,68.7998999948417,629.537703348572));
#267486=CARTESIAN_POINT('Ctrl Pts',(149.931567610411,57.4261734531929,627.537703348572));
#267487=CARTESIAN_POINT('Ctrl Pts',(153.500330774912,45.3454354230638,625.537703348572));
#267488=CARTESIAN_POINT('Ctrl Pts',(157.069093939413,33.2646973929347,623.537703348572));
#267489=CARTESIAN_POINT('Ctrl Pts',(158.704075916301,20.774415738298,621.537703348572));
#267490=CARTESIAN_POINT('Ctrl Pts',(160.339057893189,8.28413408366131,619.537703348572));
#267491=CARTESIAN_POINT('Ctrl Pts',(160.,-4.30813900827765,617.537703348572));
#267492=CARTESIAN_POINT('Ctrl Pts',(159.660942106811,-16.9004121002166,
615.537703348572));
#267493=CARTESIAN_POINT('Ctrl Pts',(157.356193074143,-29.2846130745759,
613.537703348572));
#267494=CARTESIAN_POINT('Ctrl Pts',(155.051444041476,-41.6688140489352,
611.537703348572));
#267495=CARTESIAN_POINT('Ctrl Pts',(150.837754439537,-53.5400027769194,
609.537703348572));
#267496=CARTESIAN_POINT('Ctrl Pts',(146.624064837599,-65.4111915049036,
607.537703348572));
#267497=CARTESIAN_POINT('Ctrl Pts',(140.605189688823,-76.4770599218133,
605.537703348572));
#267498=CARTESIAN_POINT('Ctrl Pts',(134.586314540048,-87.5429283387229,
603.537703348572));
#267499=CARTESIAN_POINT('Ctrl Pts',(126.9104585261,-97.530998038622,601.537703348572));
#267500=CARTESIAN_POINT('Ctrl Pts',(119.234602512152,-107.519067738521,
599.537703348572));
#267501=CARTESIAN_POINT('Ctrl Pts',(110.0907706828,-116.183399296895,597.537703348572));
#267502=CARTESIAN_POINT('Ctrl Pts',(100.946938853448,-124.847730855269,
595.537703348572));
#267503=CARTESIAN_POINT('Ctrl Pts',(90.5602826949695,-131.974979673883,
593.537703348572));
#267504=CARTESIAN_POINT('Ctrl Pts',(80.1736265364905,-139.102228492497,
591.537703348572));
#267505=CARTESIAN_POINT('Ctrl Pts',(68.7998999948417,-144.516898051454,
589.537703348572));
#267506=CARTESIAN_POINT('Ctrl Pts',(57.426173453193,-149.931567610411,587.537703348572));
#267507=CARTESIAN_POINT('Ctrl Pts',(45.3454354230638,-153.500330774912,
585.537703348572));
#267508=CARTESIAN_POINT('Ctrl Pts',(33.2646973929347,-157.069093939413,
583.537703348572));
#267509=CARTESIAN_POINT('Ctrl Pts',(20.774415738298,-158.704075916301,581.537703348572));
#267510=CARTESIAN_POINT('Ctrl Pts',(8.28413408366139,-160.339057893189,
579.537703348572));
#267511=CARTESIAN_POINT('Ctrl Pts',(-4.30813900827764,-160.,577.537703348572));
#267512=CARTESIAN_POINT('Ctrl Pts',(-16.9004121002167,-159.660942106811,
575.537703348572));
#267513=CARTESIAN_POINT('Ctrl Pts',(-29.2846130745759,-157.356193074143,
573.537703348572));
#267514=CARTESIAN_POINT('Ctrl Pts',(-41.6688140489351,-155.051444041476,
571.537703348572));
#267515=CARTESIAN_POINT('Ctrl Pts',(-53.5400027769194,-150.837754439537,
569.537703348572));
#267516=CARTESIAN_POINT('Ctrl Pts',(-65.4111915049037,-146.624064837599,
567.537703348572));
#267517=CARTESIAN_POINT('Ctrl Pts',(-76.4770599218133,-140.605189688823,
565.537703348572));
#267518=CARTESIAN_POINT('Ctrl Pts',(-87.5429283387229,-134.586314540048,
563.537703348572));
#267519=CARTESIAN_POINT('Ctrl Pts',(-97.530998038622,-126.9104585261,561.537703348572));
#267520=CARTESIAN_POINT('Ctrl Pts',(-107.519067738521,-119.234602512152,
559.537703348572));
#267521=CARTESIAN_POINT('Ctrl Pts',(-116.183399296895,-110.0907706828,557.537703348572));
#267522=CARTESIAN_POINT('Ctrl Pts',(-124.847730855269,-100.946938853448,
555.537703348572));
#267523=CARTESIAN_POINT('Ctrl Pts',(-131.974979673883,-90.5602826949695,
553.537703348572));
#267524=CARTESIAN_POINT('Ctrl Pts',(-139.102228492497,-80.1736265364905,
551.537703348572));
#267525=CARTESIAN_POINT('Ctrl Pts',(-144.516898051454,-68.7998999948417,
549.537703348572));
#267526=CARTESIAN_POINT('Ctrl Pts',(-149.931567610411,-57.426173453193,
547.537703348572));
#267527=CARTESIAN_POINT('Ctrl Pts',(-153.500330774912,-45.3454354230638,
545.537703348572));
#267528=CARTESIAN_POINT('Ctrl Pts',(-157.069093939413,-33.2646973929347,
543.537703348572));
#267529=CARTESIAN_POINT('Ctrl Pts',(-158.704075916301,-20.774415738298,
541.537703348572));
#267530=CARTESIAN_POINT('Ctrl Pts',(-160.339057893189,-8.2841340836614,
539.537703348572));
#267531=CARTESIAN_POINT('Ctrl Pts',(-160.,4.30813900827767,537.537703348572));
#267532=CARTESIAN_POINT('Ctrl Pts',(-130.,4.30813900827773,697.537703348572));
#267533=CARTESIAN_POINT('Ctrl Pts',(-129.660942106811,14.5393608954781,
695.537703348572));
#267534=CARTESIAN_POINT('Ctrl Pts',(-127.725542856289,24.591579123369,693.537703348572));
#267535=CARTESIAN_POINT('Ctrl Pts',(-125.790143605767,34.6437973512599,
691.537703348572));
#267536=CARTESIAN_POINT('Ctrl Pts',(-122.306058950683,44.269492945671,689.537703348572));
#267537=CARTESIAN_POINT('Ctrl Pts',(-118.821974295598,53.8951885400822,
687.537703348572));
#267538=CARTESIAN_POINT('Ctrl Pts',(-113.874993963172,62.8573449296269,
685.537703348572));
#267539=CARTESIAN_POINT('Ctrl Pts',(-108.928013630747,71.8195013191717,
683.537703348572));
#267540=CARTESIAN_POINT('Ctrl Pts',(-102.639948694852,79.8974404698478,
681.537703348572));
#267541=CARTESIAN_POINT('Ctrl Pts',(-96.3518837589562,87.9753796205239,
679.537703348572));
#267542=CARTESIAN_POINT('Ctrl Pts',(-88.8775672472037,94.9701958612987,
677.537703348572));
#267543=CARTESIAN_POINT('Ctrl Pts',(-81.4032507354512,101.965012102073,
675.537703348572));
#267544=CARTESIAN_POINT('Ctrl Pts',(-72.9267251261952,107.704469842635,
673.537703348572));
#267545=CARTESIAN_POINT('Ctrl Pts',(-64.4501995169392,113.443927583196,
671.537703348572));
#267546=CARTESIAN_POINT('Ctrl Pts',(-55.1801850026552,117.786702325803,
669.537703348572));
#267547=CARTESIAN_POINT('Ctrl Pts',(-45.9101704883713,122.12947706841,667.537703348572));
#267548=CARTESIAN_POINT('Ctrl Pts',(-36.0749255918153,124.968635286057,
665.537703348572));
#267549=CARTESIAN_POINT('Ctrl Pts',(-26.2396806952593,127.807793503704,
663.537703348572));
#267550=CARTESIAN_POINT('Ctrl Pts',(-16.081381787091,129.073425698447,661.537703348572));
#267551=CARTESIAN_POINT('Ctrl Pts',(-5.92308287892268,130.339057893189,
659.537703348572));
#267552=CARTESIAN_POINT('Ctrl Pts',(4.30813900827772,130.,657.537703348572));
#267553=CARTESIAN_POINT('Ctrl Pts',(14.5393608954781,129.660942106811,655.537703348572));
#267554=CARTESIAN_POINT('Ctrl Pts',(24.591579123369,127.725542856289,653.537703348572));
#267555=CARTESIAN_POINT('Ctrl Pts',(34.6437973512599,125.790143605767,651.537703348572));
#267556=CARTESIAN_POINT('Ctrl Pts',(44.269492945671,122.306058950683,649.537703348572));
#267557=CARTESIAN_POINT('Ctrl Pts',(53.8951885400822,118.821974295598,647.537703348572));
#267558=CARTESIAN_POINT('Ctrl Pts',(62.8573449296269,113.874993963172,645.537703348572));
#267559=CARTESIAN_POINT('Ctrl Pts',(71.8195013191717,108.928013630747,643.537703348572));
#267560=CARTESIAN_POINT('Ctrl Pts',(79.8974404698478,102.639948694852,641.537703348572));
#267561=CARTESIAN_POINT('Ctrl Pts',(87.9753796205239,96.3518837589562,639.537703348572));
#267562=CARTESIAN_POINT('Ctrl Pts',(94.9701958612986,88.8775672472037,637.537703348572));
#267563=CARTESIAN_POINT('Ctrl Pts',(101.965012102073,81.4032507354512,635.537703348572));
#267564=CARTESIAN_POINT('Ctrl Pts',(107.704469842635,72.9267251261952,633.537703348572));
#267565=CARTESIAN_POINT('Ctrl Pts',(113.443927583196,64.4501995169392,631.537703348572));
#267566=CARTESIAN_POINT('Ctrl Pts',(117.786702325803,55.1801850026552,629.537703348572));
#267567=CARTESIAN_POINT('Ctrl Pts',(122.12947706841,45.9101704883713,627.537703348572));
#267568=CARTESIAN_POINT('Ctrl Pts',(124.968635286057,36.0749255918153,625.537703348572));
#267569=CARTESIAN_POINT('Ctrl Pts',(127.807793503704,26.2396806952593,623.537703348572));
#267570=CARTESIAN_POINT('Ctrl Pts',(129.073425698447,16.081381787091,621.537703348572));
#267571=CARTESIAN_POINT('Ctrl Pts',(130.339057893189,5.92308287892268,619.537703348572));
#267572=CARTESIAN_POINT('Ctrl Pts',(130.,-4.30813900827772,617.537703348572));
#267573=CARTESIAN_POINT('Ctrl Pts',(129.660942106811,-14.5393608954781,
615.537703348572));
#267574=CARTESIAN_POINT('Ctrl Pts',(127.725542856289,-24.591579123369,613.537703348572));
#267575=CARTESIAN_POINT('Ctrl Pts',(125.790143605767,-34.6437973512599,
611.537703348572));
#267576=CARTESIAN_POINT('Ctrl Pts',(122.306058950683,-44.269492945671,609.537703348572));
#267577=CARTESIAN_POINT('Ctrl Pts',(118.821974295598,-53.8951885400822,
607.537703348572));
#267578=CARTESIAN_POINT('Ctrl Pts',(113.874993963172,-62.8573449296269,
605.537703348572));
#267579=CARTESIAN_POINT('Ctrl Pts',(108.928013630747,-71.8195013191717,
603.537703348572));
#267580=CARTESIAN_POINT('Ctrl Pts',(102.639948694852,-79.8974404698478,
601.537703348572));
#267581=CARTESIAN_POINT('Ctrl Pts',(96.3518837589563,-87.9753796205239,
599.537703348572));
#267582=CARTESIAN_POINT('Ctrl Pts',(88.8775672472037,-94.9701958612986,
597.537703348572));
#267583=CARTESIAN_POINT('Ctrl Pts',(81.4032507354513,-101.965012102073,
595.537703348572));
#267584=CARTESIAN_POINT('Ctrl Pts',(72.9267251261952,-107.704469842635,
593.537703348572));
#267585=CARTESIAN_POINT('Ctrl Pts',(64.4501995169392,-113.443927583196,
591.537703348572));
#267586=CARTESIAN_POINT('Ctrl Pts',(55.1801850026552,-117.786702325803,
589.537703348572));
#267587=CARTESIAN_POINT('Ctrl Pts',(45.9101704883713,-122.12947706841,587.537703348572));
#267588=CARTESIAN_POINT('Ctrl Pts',(36.0749255918153,-124.968635286057,
585.537703348572));
#267589=CARTESIAN_POINT('Ctrl Pts',(26.2396806952593,-127.807793503704,
583.537703348572));
#267590=CARTESIAN_POINT('Ctrl Pts',(16.081381787091,-129.073425698447,581.537703348572));
#267591=CARTESIAN_POINT('Ctrl Pts',(5.92308287892275,-130.339057893189,
579.537703348572));
#267592=CARTESIAN_POINT('Ctrl Pts',(-4.30813900827771,-130.,577.537703348572));
#267593=CARTESIAN_POINT('Ctrl Pts',(-14.5393608954782,-129.660942106811,
575.537703348572));
#267594=CARTESIAN_POINT('Ctrl Pts',(-24.591579123369,-127.725542856289,
573.537703348572));
#267595=CARTESIAN_POINT('Ctrl Pts',(-34.6437973512598,-125.790143605767,
571.537703348572));
#267596=CARTESIAN_POINT('Ctrl Pts',(-44.269492945671,-122.306058950683,
569.537703348572));
#267597=CARTESIAN_POINT('Ctrl Pts',(-53.8951885400822,-118.821974295598,
567.537703348572));
#267598=CARTESIAN_POINT('Ctrl Pts',(-62.8573449296269,-113.874993963172,
565.537703348572));
#267599=CARTESIAN_POINT('Ctrl Pts',(-71.8195013191717,-108.928013630747,
563.537703348572));
#267600=CARTESIAN_POINT('Ctrl Pts',(-79.8974404698478,-102.639948694852,
561.537703348572));
#267601=CARTESIAN_POINT('Ctrl Pts',(-87.975379620524,-96.3518837589562,
559.537703348572));
#267602=CARTESIAN_POINT('Ctrl Pts',(-94.9701958612986,-88.8775672472037,
557.537703348572));
#267603=CARTESIAN_POINT('Ctrl Pts',(-101.965012102073,-81.4032507354513,
555.537703348572));
#267604=CARTESIAN_POINT('Ctrl Pts',(-107.704469842635,-72.9267251261952,
553.537703348572));
#267605=CARTESIAN_POINT('Ctrl Pts',(-113.443927583196,-64.4501995169392,
551.537703348572));
#267606=CARTESIAN_POINT('Ctrl Pts',(-117.786702325803,-55.1801850026553,
549.537703348572));
#267607=CARTESIAN_POINT('Ctrl Pts',(-122.12947706841,-45.9101704883713,
547.537703348572));
#267608=CARTESIAN_POINT('Ctrl Pts',(-124.968635286057,-36.0749255918153,
545.537703348572));
#267609=CARTESIAN_POINT('Ctrl Pts',(-127.807793503704,-26.2396806952593,
543.537703348572));
#267610=CARTESIAN_POINT('Ctrl Pts',(-129.073425698447,-16.081381787091,
541.537703348572));
#267611=CARTESIAN_POINT('Ctrl Pts',(-130.339057893189,-5.92308287892275,
539.537703348572));
#267612=CARTESIAN_POINT('Ctrl Pts',(-130.,4.30813900827773,537.537703348572));
#267613=CARTESIAN_POINT('Ctrl Pts',(-159.895664541343,7.20669984090177,
697.076891283416));
#267614=CARTESIAN_POINT('Ctrl Pts',(-159.394142202012,18.3340187941072,
695.306181476978));
#267615=CARTESIAN_POINT('Ctrl Pts',(-157.356193074143,29.2846130745759,
693.537703348572));
#267616=CARTESIAN_POINT('Ctrl Pts',(-155.051444041476,41.6688140489352,
691.537703348572));
#267617=CARTESIAN_POINT('Ctrl Pts',(-150.837754439537,53.5400027769194,
689.537703348572));
#267618=CARTESIAN_POINT('Ctrl Pts',(-146.624064837599,65.4111915049037,
687.537703348572));
#267619=CARTESIAN_POINT('Ctrl Pts',(-140.605189688823,76.4770599218133,
685.537703348572));
#267620=CARTESIAN_POINT('Ctrl Pts',(-134.586314540048,87.542928338723,683.537703348572));
#267621=CARTESIAN_POINT('Ctrl Pts',(-126.9104585261,97.530998038622,681.537703348572));
#267622=CARTESIAN_POINT('Ctrl Pts',(-119.234602512152,107.519067738521,
679.537703348572));
#267623=CARTESIAN_POINT('Ctrl Pts',(-110.0907706828,116.183399296895,677.537703348572));
#267624=CARTESIAN_POINT('Ctrl Pts',(-100.946938853448,124.847730855269,
675.537703348572));
#267625=CARTESIAN_POINT('Ctrl Pts',(-90.5602826949695,131.974979673883,
673.537703348572));
#267626=CARTESIAN_POINT('Ctrl Pts',(-80.1736265364906,139.102228492497,
671.537703348572));
#267627=CARTESIAN_POINT('Ctrl Pts',(-68.7998999948417,144.516898051454,
669.537703348572));
#267628=CARTESIAN_POINT('Ctrl Pts',(-57.4261734531929,149.931567610411,
667.537703348572));
#267629=CARTESIAN_POINT('Ctrl Pts',(-45.3454354230638,153.500330774912,
665.537703348572));
#267630=CARTESIAN_POINT('Ctrl Pts',(-33.2646973929347,157.069093939413,
663.537703348572));
#267631=CARTESIAN_POINT('Ctrl Pts',(-20.774415738298,158.704075916301,661.537703348572));
#267632=CARTESIAN_POINT('Ctrl Pts',(-8.28413408366129,160.339057893189,
659.537703348572));
#267633=CARTESIAN_POINT('Ctrl Pts',(4.30813900827766,160.,657.537703348572));
#267634=CARTESIAN_POINT('Ctrl Pts',(16.9004121002166,159.660942106811,655.537703348572));
#267635=CARTESIAN_POINT('Ctrl Pts',(29.2846130745759,157.356193074143,653.537703348572));
#267636=CARTESIAN_POINT('Ctrl Pts',(41.6688140489352,155.051444041476,651.537703348572));
#267637=CARTESIAN_POINT('Ctrl Pts',(53.5400027769194,150.837754439537,649.537703348572));
#267638=CARTESIAN_POINT('Ctrl Pts',(65.4111915049037,146.624064837599,647.537703348572));
#267639=CARTESIAN_POINT('Ctrl Pts',(76.4770599218133,140.605189688823,645.537703348572));
#267640=CARTESIAN_POINT('Ctrl Pts',(87.542928338723,134.586314540048,643.537703348572));
#267641=CARTESIAN_POINT('Ctrl Pts',(97.530998038622,126.9104585261,641.537703348572));
#267642=CARTESIAN_POINT('Ctrl Pts',(107.519067738521,119.234602512152,639.537703348572));
#267643=CARTESIAN_POINT('Ctrl Pts',(116.183399296895,110.0907706828,637.537703348572));
#267644=CARTESIAN_POINT('Ctrl Pts',(124.847730855269,100.946938853448,635.537703348572));
#267645=CARTESIAN_POINT('Ctrl Pts',(131.974979673883,90.5602826949695,633.537703348572));
#267646=CARTESIAN_POINT('Ctrl Pts',(139.102228492497,80.1736265364906,631.537703348572));
#267647=CARTESIAN_POINT('Ctrl Pts',(144.516898051454,68.7998999948417,629.537703348572));
#267648=CARTESIAN_POINT('Ctrl Pts',(149.931567610411,57.4261734531929,627.537703348572));
#267649=CARTESIAN_POINT('Ctrl Pts',(153.500330774912,45.3454354230638,625.537703348572));
#267650=CARTESIAN_POINT('Ctrl Pts',(157.069093939413,33.2646973929347,623.537703348572));
#267651=CARTESIAN_POINT('Ctrl Pts',(158.704075916301,20.774415738298,621.537703348572));
#267652=CARTESIAN_POINT('Ctrl Pts',(160.339057893189,8.28413408366131,619.537703348572));
#267653=CARTESIAN_POINT('Ctrl Pts',(160.,-4.30813900827765,617.537703348572));
#267654=CARTESIAN_POINT('Ctrl Pts',(159.660942106811,-16.9004121002166,
615.537703348572));
#267655=CARTESIAN_POINT('Ctrl Pts',(157.356193074143,-29.2846130745759,
613.537703348572));
#267656=CARTESIAN_POINT('Ctrl Pts',(155.051444041476,-41.6688140489352,
611.537703348572));
#267657=CARTESIAN_POINT('Ctrl Pts',(150.837754439537,-53.5400027769194,
609.537703348572));
#267658=CARTESIAN_POINT('Ctrl Pts',(146.624064837599,-65.4111915049036,
607.537703348572));
#267659=CARTESIAN_POINT('Ctrl Pts',(140.605189688823,-76.4770599218133,
605.537703348572));
#267660=CARTESIAN_POINT('Ctrl Pts',(134.586314540048,-87.5429283387229,
603.537703348572));
#267661=CARTESIAN_POINT('Ctrl Pts',(126.9104585261,-97.530998038622,601.537703348572));
#267662=CARTESIAN_POINT('Ctrl Pts',(119.234602512152,-107.519067738521,
599.537703348572));
#267663=CARTESIAN_POINT('Ctrl Pts',(110.0907706828,-116.183399296895,597.537703348572));
#267664=CARTESIAN_POINT('Ctrl Pts',(100.946938853448,-124.847730855269,
595.537703348572));
#267665=CARTESIAN_POINT('Ctrl Pts',(90.5602826949695,-131.974979673883,
593.537703348572));
#267666=CARTESIAN_POINT('Ctrl Pts',(80.1736265364905,-139.102228492497,
591.537703348572));
#267667=CARTESIAN_POINT('Ctrl Pts',(68.7998999948417,-144.516898051454,
589.537703348572));
#267668=CARTESIAN_POINT('Ctrl Pts',(57.426173453193,-149.931567610411,587.537703348572));
#267669=CARTESIAN_POINT('Ctrl Pts',(45.3454354230638,-153.500330774912,
585.537703348572));
#267670=CARTESIAN_POINT('Ctrl Pts',(33.2646973929347,-157.069093939413,
583.537703348572));
#267671=CARTESIAN_POINT('Ctrl Pts',(20.774415738298,-158.704075916301,581.537703348572));
#267672=CARTESIAN_POINT('Ctrl Pts',(8.28413408366139,-160.339057893189,
579.537703348572));
#267673=CARTESIAN_POINT('Ctrl Pts',(-4.30813900827764,-160.,577.537703348572));
#267674=CARTESIAN_POINT('Ctrl Pts',(-16.9004121002167,-159.660942106811,
575.537703348572));
#267675=CARTESIAN_POINT('Ctrl Pts',(-29.2846130745759,-157.356193074143,
573.537703348572));
#267676=CARTESIAN_POINT('Ctrl Pts',(-41.6688140489351,-155.051444041476,
571.537703348572));
#267677=CARTESIAN_POINT('Ctrl Pts',(-53.5400027769194,-150.837754439537,
569.537703348572));
#267678=CARTESIAN_POINT('Ctrl Pts',(-65.4111915049037,-146.624064837599,
567.537703348572));
#267679=CARTESIAN_POINT('Ctrl Pts',(-76.4770599218133,-140.605189688823,
565.537703348572));
#267680=CARTESIAN_POINT('Ctrl Pts',(-87.5429283387229,-134.586314540048,
563.537703348572));
#267681=CARTESIAN_POINT('Ctrl Pts',(-97.530998038622,-126.9104585261,561.537703348572));
#267682=CARTESIAN_POINT('Ctrl Pts',(-107.519067738521,-119.234602512152,
559.537703348572));
#267683=CARTESIAN_POINT('Ctrl Pts',(-116.183399296895,-110.0907706828,557.537703348572));
#267684=CARTESIAN_POINT('Ctrl Pts',(-124.847730855269,-100.946938853448,
555.537703348572));
#267685=CARTESIAN_POINT('Ctrl Pts',(-131.974979673883,-90.5602826949695,
553.537703348572));
#267686=CARTESIAN_POINT('Ctrl Pts',(-139.102228492497,-80.1736265364905,
551.537703348572));
#267687=CARTESIAN_POINT('Ctrl Pts',(-144.516898051454,-68.7998999948417,
549.537703348572));
#267688=CARTESIAN_POINT('Ctrl Pts',(-149.931567610411,-57.426173453193,
547.537703348572));
#267689=CARTESIAN_POINT('Ctrl Pts',(-153.500330774912,-45.3454354230638,
545.537703348572));
#267690=CARTESIAN_POINT('Ctrl Pts',(-157.069093939413,-33.2646973929347,
543.537703348572));
#267691=CARTESIAN_POINT('Ctrl Pts',(-158.704075916301,-20.774415738298,
541.537703348572));
#267692=CARTESIAN_POINT('Ctrl Pts',(-159.653854600275,-13.5186762622036,
540.375881753716));
#267693=CARTESIAN_POINT('Ctrl Pts',(-159.937609420477,-6.20654127333065,
539.210563551645));
#267694=CARTESIAN_POINT('Ctrl Pts',(-160.,-4.30813900827851,692.462296651429));
#267695=CARTESIAN_POINT('Ctrl Pts',(-160.339057893189,8.28413408366045,
690.462296651429));
#267696=CARTESIAN_POINT('Ctrl Pts',(-158.704075916301,20.7744157382972,
688.462296651429));
#267697=CARTESIAN_POINT('Ctrl Pts',(-157.069093939413,33.2646973929339,
686.462296651429));
#267698=CARTESIAN_POINT('Ctrl Pts',(-153.500330774912,45.345435423063,684.462296651429));
#267699=CARTESIAN_POINT('Ctrl Pts',(-149.931567610412,57.4261734531921,
682.462296651429));
#267700=CARTESIAN_POINT('Ctrl Pts',(-144.516898051455,68.7998999948409,
680.462296651429));
#267701=CARTESIAN_POINT('Ctrl Pts',(-139.102228492498,80.1736265364898,
678.462296651429));
#267702=CARTESIAN_POINT('Ctrl Pts',(-131.974979673884,90.5602826949688,
676.462296651429));
#267703=CARTESIAN_POINT('Ctrl Pts',(-124.84773085527,100.946938853448,674.462296651429));
#267704=CARTESIAN_POINT('Ctrl Pts',(-116.183399296896,110.0907706828,672.462296651429));
#267705=CARTESIAN_POINT('Ctrl Pts',(-107.519067738522,119.234602512151,
670.462296651429));
#267706=CARTESIAN_POINT('Ctrl Pts',(-97.5309980386227,126.9104585261,668.462296651429));
#267707=CARTESIAN_POINT('Ctrl Pts',(-87.5429283387237,134.586314540048,
666.462296651429));
#267708=CARTESIAN_POINT('Ctrl Pts',(-76.4770599218141,140.605189688823,
664.462296651429));
#267709=CARTESIAN_POINT('Ctrl Pts',(-65.4111915049045,146.624064837598,
662.462296651429));
#267710=CARTESIAN_POINT('Ctrl Pts',(-53.5400027769202,150.837754439537,
660.462296651429));
#267711=CARTESIAN_POINT('Ctrl Pts',(-41.668814048936,155.051444041475,658.462296651429));
#267712=CARTESIAN_POINT('Ctrl Pts',(-29.2846130745767,157.356193074143,
656.462296651429));
#267713=CARTESIAN_POINT('Ctrl Pts',(-16.9004121002175,159.660942106811,
654.462296651428));
#267714=CARTESIAN_POINT('Ctrl Pts',(-4.30813900827852,160.,652.462296651429));
#267715=CARTESIAN_POINT('Ctrl Pts',(8.28413408366043,160.339057893189,650.462296651429));
#267716=CARTESIAN_POINT('Ctrl Pts',(20.7744157382972,158.704075916301,648.462296651428));
#267717=CARTESIAN_POINT('Ctrl Pts',(33.2646973929339,157.069093939413,646.462296651429));
#267718=CARTESIAN_POINT('Ctrl Pts',(45.345435423063,153.500330774912,644.462296651428));
#267719=CARTESIAN_POINT('Ctrl Pts',(57.4261734531921,149.931567610412,642.462296651428));
#267720=CARTESIAN_POINT('Ctrl Pts',(68.7998999948409,144.516898051455,640.462296651428));
#267721=CARTESIAN_POINT('Ctrl Pts',(80.1736265364898,139.102228492498,638.462296651429));
#267722=CARTESIAN_POINT('Ctrl Pts',(90.5602826949688,131.974979673884,636.462296651428));
#267723=CARTESIAN_POINT('Ctrl Pts',(100.946938853448,124.84773085527,634.462296651428));
#267724=CARTESIAN_POINT('Ctrl Pts',(110.0907706828,116.183399296896,632.462296651429));
#267725=CARTESIAN_POINT('Ctrl Pts',(119.234602512151,107.519067738522,630.462296651429));
#267726=CARTESIAN_POINT('Ctrl Pts',(126.9104585261,97.5309980386227,628.462296651429));
#267727=CARTESIAN_POINT('Ctrl Pts',(134.586314540048,87.5429283387237,626.462296651429));
#267728=CARTESIAN_POINT('Ctrl Pts',(140.605189688823,76.4770599218141,624.462296651429));
#267729=CARTESIAN_POINT('Ctrl Pts',(146.624064837598,65.4111915049045,622.462296651429));
#267730=CARTESIAN_POINT('Ctrl Pts',(150.837754439537,53.5400027769202,620.462296651429));
#267731=CARTESIAN_POINT('Ctrl Pts',(155.051444041475,41.668814048936,618.462296651429));
#267732=CARTESIAN_POINT('Ctrl Pts',(157.356193074143,29.2846130745767,616.462296651429));
#267733=CARTESIAN_POINT('Ctrl Pts',(159.660942106811,16.9004121002175,614.462296651429));
#267734=CARTESIAN_POINT('Ctrl Pts',(160.,4.30813900827853,612.462296651429));
#267735=CARTESIAN_POINT('Ctrl Pts',(160.339057893189,-8.28413408366043,
610.462296651429));
#267736=CARTESIAN_POINT('Ctrl Pts',(158.704075916301,-20.7744157382971,
608.462296651429));
#267737=CARTESIAN_POINT('Ctrl Pts',(157.069093939413,-33.2646973929339,
606.462296651429));
#267738=CARTESIAN_POINT('Ctrl Pts',(153.500330774912,-45.345435423063,604.462296651429));
#267739=CARTESIAN_POINT('Ctrl Pts',(149.931567610412,-57.4261734531921,
602.462296651429));
#267740=CARTESIAN_POINT('Ctrl Pts',(144.516898051455,-68.7998999948409,
600.462296651429));
#267741=CARTESIAN_POINT('Ctrl Pts',(139.102228492498,-80.1736265364898,
598.462296651429));
#267742=CARTESIAN_POINT('Ctrl Pts',(131.974979673884,-90.5602826949688,
596.462296651429));
#267743=CARTESIAN_POINT('Ctrl Pts',(124.84773085527,-100.946938853448,594.462296651428));
#267744=CARTESIAN_POINT('Ctrl Pts',(116.183399296896,-110.0907706828,592.462296651429));
#267745=CARTESIAN_POINT('Ctrl Pts',(107.519067738522,-119.234602512151,
590.462296651429));
#267746=CARTESIAN_POINT('Ctrl Pts',(97.5309980386227,-126.9104585261,588.462296651429));
#267747=CARTESIAN_POINT('Ctrl Pts',(87.5429283387236,-134.586314540048,
586.462296651429));
#267748=CARTESIAN_POINT('Ctrl Pts',(76.4770599218141,-140.605189688823,
584.462296651429));
#267749=CARTESIAN_POINT('Ctrl Pts',(65.4111915049046,-146.624064837598,
582.462296651428));
#267750=CARTESIAN_POINT('Ctrl Pts',(53.5400027769202,-150.837754439537,
580.462296651429));
#267751=CARTESIAN_POINT('Ctrl Pts',(41.6688140489359,-155.051444041475,
578.462296651429));
#267752=CARTESIAN_POINT('Ctrl Pts',(29.2846130745768,-157.356193074143,
576.462296651429));
#267753=CARTESIAN_POINT('Ctrl Pts',(16.9004121002176,-159.660942106811,
574.462296651429));
#267754=CARTESIAN_POINT('Ctrl Pts',(4.30813900827854,-160.,572.462296651429));
#267755=CARTESIAN_POINT('Ctrl Pts',(-8.28413408366049,-160.339057893189,
570.462296651428));
#267756=CARTESIAN_POINT('Ctrl Pts',(-20.7744157382971,-158.704075916301,
568.462296651429));
#267757=CARTESIAN_POINT('Ctrl Pts',(-33.2646973929338,-157.069093939413,
566.462296651429));
#267758=CARTESIAN_POINT('Ctrl Pts',(-45.345435423063,-153.500330774912,
564.462296651429));
#267759=CARTESIAN_POINT('Ctrl Pts',(-57.4261734531921,-149.931567610412,
562.462296651429));
#267760=CARTESIAN_POINT('Ctrl Pts',(-68.7998999948409,-144.516898051455,
560.462296651429));
#267761=CARTESIAN_POINT('Ctrl Pts',(-80.1736265364897,-139.102228492498,
558.462296651429));
#267762=CARTESIAN_POINT('Ctrl Pts',(-90.5602826949688,-131.974979673884,
556.462296651429));
#267763=CARTESIAN_POINT('Ctrl Pts',(-100.946938853448,-124.84773085527,
554.462296651429));
#267764=CARTESIAN_POINT('Ctrl Pts',(-110.0907706828,-116.183399296896,552.462296651429));
#267765=CARTESIAN_POINT('Ctrl Pts',(-119.234602512151,-107.519067738522,
550.462296651429));
#267766=CARTESIAN_POINT('Ctrl Pts',(-126.9104585261,-97.5309980386227,548.462296651429));
#267767=CARTESIAN_POINT('Ctrl Pts',(-134.586314540048,-87.5429283387236,
546.462296651429));
#267768=CARTESIAN_POINT('Ctrl Pts',(-140.605189688823,-76.4770599218141,
544.462296651429));
#267769=CARTESIAN_POINT('Ctrl Pts',(-146.624064837598,-65.4111915049046,
542.462296651429));
#267770=CARTESIAN_POINT('Ctrl Pts',(-150.837754439537,-53.5400027769203,
540.462296651429));
#267771=CARTESIAN_POINT('Ctrl Pts',(-155.051444041475,-41.668814048936,
538.462296651429));
#267772=CARTESIAN_POINT('Ctrl Pts',(-157.356193074143,-29.2846130745768,
536.462296651429));
#267773=CARTESIAN_POINT('Ctrl Pts',(-159.660942106811,-16.9004121002176,
534.462296651429));
#267774=CARTESIAN_POINT('Ctrl Pts',(-160.,-4.30813900827851,532.462296651429));
#267775=CARTESIAN_POINT('Ctrl Pts',(-160.,4.30813900827767,697.537703348572));
#267776=CARTESIAN_POINT('Ctrl Pts',(-159.660942106811,16.9004121002166,
695.537703348572));
#267777=CARTESIAN_POINT('Ctrl Pts',(-157.356193074143,29.2846130745759,
693.537703348572));
#267778=CARTESIAN_POINT('Ctrl Pts',(-155.051444041476,41.6688140489352,
691.537703348572));
#267779=CARTESIAN_POINT('Ctrl Pts',(-150.837754439537,53.5400027769194,
689.537703348572));
#267780=CARTESIAN_POINT('Ctrl Pts',(-146.624064837599,65.4111915049037,
687.537703348572));
#267781=CARTESIAN_POINT('Ctrl Pts',(-140.605189688823,76.4770599218133,
685.537703348572));
#267782=CARTESIAN_POINT('Ctrl Pts',(-134.586314540048,87.542928338723,683.537703348572));
#267783=CARTESIAN_POINT('Ctrl Pts',(-126.9104585261,97.530998038622,681.537703348572));
#267784=CARTESIAN_POINT('Ctrl Pts',(-119.234602512152,107.519067738521,
679.537703348572));
#267785=CARTESIAN_POINT('Ctrl Pts',(-110.0907706828,116.183399296895,677.537703348572));
#267786=CARTESIAN_POINT('Ctrl Pts',(-100.946938853448,124.847730855269,
675.537703348572));
#267787=CARTESIAN_POINT('Ctrl Pts',(-90.5602826949695,131.974979673883,
673.537703348572));
#267788=CARTESIAN_POINT('Ctrl Pts',(-80.1736265364906,139.102228492497,
671.537703348572));
#267789=CARTESIAN_POINT('Ctrl Pts',(-68.7998999948417,144.516898051454,
669.537703348572));
#267790=CARTESIAN_POINT('Ctrl Pts',(-57.4261734531929,149.931567610411,
667.537703348572));
#267791=CARTESIAN_POINT('Ctrl Pts',(-45.3454354230638,153.500330774912,
665.537703348572));
#267792=CARTESIAN_POINT('Ctrl Pts',(-33.2646973929347,157.069093939413,
663.537703348572));
#267793=CARTESIAN_POINT('Ctrl Pts',(-20.774415738298,158.704075916301,661.537703348572));
#267794=CARTESIAN_POINT('Ctrl Pts',(-8.28413408366129,160.339057893189,
659.537703348572));
#267795=CARTESIAN_POINT('Ctrl Pts',(4.30813900827766,160.,657.537703348572));
#267796=CARTESIAN_POINT('Ctrl Pts',(16.9004121002166,159.660942106811,655.537703348572));
#267797=CARTESIAN_POINT('Ctrl Pts',(29.2846130745759,157.356193074143,653.537703348572));
#267798=CARTESIAN_POINT('Ctrl Pts',(41.6688140489352,155.051444041476,651.537703348572));
#267799=CARTESIAN_POINT('Ctrl Pts',(53.5400027769194,150.837754439537,649.537703348572));
#267800=CARTESIAN_POINT('Ctrl Pts',(65.4111915049037,146.624064837599,647.537703348572));
#267801=CARTESIAN_POINT('Ctrl Pts',(76.4770599218133,140.605189688823,645.537703348572));
#267802=CARTESIAN_POINT('Ctrl Pts',(87.542928338723,134.586314540048,643.537703348572));
#267803=CARTESIAN_POINT('Ctrl Pts',(97.530998038622,126.9104585261,641.537703348572));
#267804=CARTESIAN_POINT('Ctrl Pts',(107.519067738521,119.234602512152,639.537703348572));
#267805=CARTESIAN_POINT('Ctrl Pts',(116.183399296895,110.0907706828,637.537703348572));
#267806=CARTESIAN_POINT('Ctrl Pts',(124.847730855269,100.946938853448,635.537703348572));
#267807=CARTESIAN_POINT('Ctrl Pts',(131.974979673883,90.5602826949695,633.537703348572));
#267808=CARTESIAN_POINT('Ctrl Pts',(139.102228492497,80.1736265364906,631.537703348572));
#267809=CARTESIAN_POINT('Ctrl Pts',(144.516898051454,68.7998999948417,629.537703348572));
#267810=CARTESIAN_POINT('Ctrl Pts',(149.931567610411,57.4261734531929,627.537703348572));
#267811=CARTESIAN_POINT('Ctrl Pts',(153.500330774912,45.3454354230638,625.537703348572));
#267812=CARTESIAN_POINT('Ctrl Pts',(157.069093939413,33.2646973929347,623.537703348572));
#267813=CARTESIAN_POINT('Ctrl Pts',(158.704075916301,20.774415738298,621.537703348572));
#267814=CARTESIAN_POINT('Ctrl Pts',(160.339057893189,8.28413408366131,619.537703348572));
#267815=CARTESIAN_POINT('Ctrl Pts',(160.,-4.30813900827765,617.537703348572));
#267816=CARTESIAN_POINT('Ctrl Pts',(159.660942106811,-16.9004121002166,
615.537703348572));
#267817=CARTESIAN_POINT('Ctrl Pts',(157.356193074143,-29.2846130745759,
613.537703348572));
#267818=CARTESIAN_POINT('Ctrl Pts',(155.051444041476,-41.6688140489352,
611.537703348572));
#267819=CARTESIAN_POINT('Ctrl Pts',(150.837754439537,-53.5400027769194,
609.537703348572));
#267820=CARTESIAN_POINT('Ctrl Pts',(146.624064837599,-65.4111915049036,
607.537703348572));
#267821=CARTESIAN_POINT('Ctrl Pts',(140.605189688823,-76.4770599218133,
605.537703348572));
#267822=CARTESIAN_POINT('Ctrl Pts',(134.586314540048,-87.5429283387229,
603.537703348572));
#267823=CARTESIAN_POINT('Ctrl Pts',(126.9104585261,-97.530998038622,601.537703348572));
#267824=CARTESIAN_POINT('Ctrl Pts',(119.234602512152,-107.519067738521,
599.537703348572));
#267825=CARTESIAN_POINT('Ctrl Pts',(110.0907706828,-116.183399296895,597.537703348572));
#267826=CARTESIAN_POINT('Ctrl Pts',(100.946938853448,-124.847730855269,
595.537703348572));
#267827=CARTESIAN_POINT('Ctrl Pts',(90.5602826949695,-131.974979673883,
593.537703348572));
#267828=CARTESIAN_POINT('Ctrl Pts',(80.1736265364905,-139.102228492497,
591.537703348572));
#267829=CARTESIAN_POINT('Ctrl Pts',(68.7998999948417,-144.516898051454,
589.537703348572));
#267830=CARTESIAN_POINT('Ctrl Pts',(57.426173453193,-149.931567610411,587.537703348572));
#267831=CARTESIAN_POINT('Ctrl Pts',(45.3454354230638,-153.500330774912,
585.537703348572));
#267832=CARTESIAN_POINT('Ctrl Pts',(33.2646973929347,-157.069093939413,
583.537703348572));
#267833=CARTESIAN_POINT('Ctrl Pts',(20.774415738298,-158.704075916301,581.537703348572));
#267834=CARTESIAN_POINT('Ctrl Pts',(8.28413408366139,-160.339057893189,
579.537703348572));
#267835=CARTESIAN_POINT('Ctrl Pts',(-4.30813900827764,-160.,577.537703348572));
#267836=CARTESIAN_POINT('Ctrl Pts',(-16.9004121002167,-159.660942106811,
575.537703348572));
#267837=CARTESIAN_POINT('Ctrl Pts',(-29.2846130745759,-157.356193074143,
573.537703348572));
#267838=CARTESIAN_POINT('Ctrl Pts',(-41.6688140489351,-155.051444041476,
571.537703348572));
#267839=CARTESIAN_POINT('Ctrl Pts',(-53.5400027769194,-150.837754439537,
569.537703348572));
#267840=CARTESIAN_POINT('Ctrl Pts',(-65.4111915049037,-146.624064837599,
567.537703348572));
#267841=CARTESIAN_POINT('Ctrl Pts',(-76.4770599218133,-140.605189688823,
565.537703348572));
#267842=CARTESIAN_POINT('Ctrl Pts',(-87.5429283387229,-134.586314540048,
563.537703348572));
#267843=CARTESIAN_POINT('Ctrl Pts',(-97.530998038622,-126.9104585261,561.537703348572));
#267844=CARTESIAN_POINT('Ctrl Pts',(-107.519067738521,-119.234602512152,
559.537703348572));
#267845=CARTESIAN_POINT('Ctrl Pts',(-116.183399296895,-110.0907706828,557.537703348572));
#267846=CARTESIAN_POINT('Ctrl Pts',(-124.847730855269,-100.946938853448,
555.537703348572));
#267847=CARTESIAN_POINT('Ctrl Pts',(-131.974979673883,-90.5602826949695,
553.537703348572));
#267848=CARTESIAN_POINT('Ctrl Pts',(-139.102228492497,-80.1736265364905,
551.537703348572));
#267849=CARTESIAN_POINT('Ctrl Pts',(-144.516898051454,-68.7998999948417,
549.537703348572));
#267850=CARTESIAN_POINT('Ctrl Pts',(-149.931567610411,-57.426173453193,
547.537703348572));
#267851=CARTESIAN_POINT('Ctrl Pts',(-153.500330774912,-45.3454354230638,
545.537703348572));
#267852=CARTESIAN_POINT('Ctrl Pts',(-157.069093939413,-33.2646973929347,
543.537703348572));
#267853=CARTESIAN_POINT('Ctrl Pts',(-158.704075916301,-20.774415738298,
541.537703348572));
#267854=CARTESIAN_POINT('Ctrl Pts',(-160.339057893189,-8.2841340836614,
539.537703348572));
#267855=CARTESIAN_POINT('Ctrl Pts',(-160.,4.30813900827767,537.537703348572));
#267856=CARTESIAN_POINT('Ctrl Pts',(-159.937609420477,6.20654127332979,
690.789436448355));
#267857=CARTESIAN_POINT('Ctrl Pts',(-159.653854600276,13.5186762622027,
689.624118246285));
#267858=CARTESIAN_POINT('Ctrl Pts',(-158.704075916301,20.7744157382972,
688.462296651429));
#267859=CARTESIAN_POINT('Ctrl Pts',(-157.069093939413,33.2646973929339,
686.462296651429));
#267860=CARTESIAN_POINT('Ctrl Pts',(-153.500330774912,45.345435423063,684.462296651429));
#267861=CARTESIAN_POINT('Ctrl Pts',(-149.931567610412,57.4261734531921,
682.462296651429));
#267862=CARTESIAN_POINT('Ctrl Pts',(-144.516898051455,68.7998999948409,
680.462296651429));
#267863=CARTESIAN_POINT('Ctrl Pts',(-139.102228492498,80.1736265364898,
678.462296651429));
#267864=CARTESIAN_POINT('Ctrl Pts',(-131.974979673884,90.5602826949688,
676.462296651429));
#267865=CARTESIAN_POINT('Ctrl Pts',(-124.84773085527,100.946938853448,674.462296651429));
#267866=CARTESIAN_POINT('Ctrl Pts',(-116.183399296896,110.0907706828,672.462296651429));
#267867=CARTESIAN_POINT('Ctrl Pts',(-107.519067738522,119.234602512151,
670.462296651429));
#267868=CARTESIAN_POINT('Ctrl Pts',(-97.5309980386227,126.9104585261,668.462296651429));
#267869=CARTESIAN_POINT('Ctrl Pts',(-87.5429283387237,134.586314540048,
666.462296651429));
#267870=CARTESIAN_POINT('Ctrl Pts',(-76.4770599218141,140.605189688823,
664.462296651429));
#267871=CARTESIAN_POINT('Ctrl Pts',(-65.4111915049045,146.624064837598,
662.462296651429));
#267872=CARTESIAN_POINT('Ctrl Pts',(-53.5400027769202,150.837754439537,
660.462296651429));
#267873=CARTESIAN_POINT('Ctrl Pts',(-41.668814048936,155.051444041475,658.462296651429));
#267874=CARTESIAN_POINT('Ctrl Pts',(-29.2846130745767,157.356193074143,
656.462296651429));
#267875=CARTESIAN_POINT('Ctrl Pts',(-16.9004121002175,159.660942106811,
654.462296651429));
#267876=CARTESIAN_POINT('Ctrl Pts',(-4.30813900827852,160.,652.462296651429));
#267877=CARTESIAN_POINT('Ctrl Pts',(8.28413408366043,160.339057893189,650.462296651429));
#267878=CARTESIAN_POINT('Ctrl Pts',(20.7744157382972,158.704075916301,648.462296651428));
#267879=CARTESIAN_POINT('Ctrl Pts',(33.2646973929339,157.069093939413,646.462296651429));
#267880=CARTESIAN_POINT('Ctrl Pts',(45.345435423063,153.500330774912,644.462296651428));
#267881=CARTESIAN_POINT('Ctrl Pts',(57.4261734531921,149.931567610412,642.462296651428));
#267882=CARTESIAN_POINT('Ctrl Pts',(68.7998999948409,144.516898051455,640.462296651428));
#267883=CARTESIAN_POINT('Ctrl Pts',(80.1736265364898,139.102228492498,638.462296651429));
#267884=CARTESIAN_POINT('Ctrl Pts',(90.5602826949688,131.974979673884,636.462296651428));
#267885=CARTESIAN_POINT('Ctrl Pts',(100.946938853448,124.84773085527,634.462296651428));
#267886=CARTESIAN_POINT('Ctrl Pts',(110.0907706828,116.183399296896,632.462296651429));
#267887=CARTESIAN_POINT('Ctrl Pts',(119.234602512151,107.519067738522,630.462296651429));
#267888=CARTESIAN_POINT('Ctrl Pts',(126.9104585261,97.5309980386227,628.462296651429));
#267889=CARTESIAN_POINT('Ctrl Pts',(134.586314540048,87.5429283387237,626.462296651429));
#267890=CARTESIAN_POINT('Ctrl Pts',(140.605189688823,76.4770599218141,624.462296651429));
#267891=CARTESIAN_POINT('Ctrl Pts',(146.624064837598,65.4111915049045,622.462296651429));
#267892=CARTESIAN_POINT('Ctrl Pts',(150.837754439537,53.5400027769202,620.462296651429));
#267893=CARTESIAN_POINT('Ctrl Pts',(155.051444041475,41.668814048936,618.462296651429));
#267894=CARTESIAN_POINT('Ctrl Pts',(157.356193074143,29.2846130745767,616.462296651429));
#267895=CARTESIAN_POINT('Ctrl Pts',(159.660942106811,16.9004121002175,614.462296651429));
#267896=CARTESIAN_POINT('Ctrl Pts',(160.,4.30813900827853,612.462296651429));
#267897=CARTESIAN_POINT('Ctrl Pts',(160.339057893189,-8.28413408366043,
610.462296651429));
#267898=CARTESIAN_POINT('Ctrl Pts',(158.704075916301,-20.7744157382971,
608.462296651429));
#267899=CARTESIAN_POINT('Ctrl Pts',(157.069093939413,-33.2646973929339,
606.462296651429));
#267900=CARTESIAN_POINT('Ctrl Pts',(153.500330774912,-45.345435423063,604.462296651429));
#267901=CARTESIAN_POINT('Ctrl Pts',(149.931567610412,-57.4261734531921,
602.462296651429));
#267902=CARTESIAN_POINT('Ctrl Pts',(144.516898051455,-68.7998999948409,
600.462296651429));
#267903=CARTESIAN_POINT('Ctrl Pts',(139.102228492498,-80.1736265364898,
598.462296651429));
#267904=CARTESIAN_POINT('Ctrl Pts',(131.974979673884,-90.5602826949688,
596.462296651429));
#267905=CARTESIAN_POINT('Ctrl Pts',(124.84773085527,-100.946938853448,594.462296651429));
#267906=CARTESIAN_POINT('Ctrl Pts',(116.183399296896,-110.0907706828,592.462296651429));
#267907=CARTESIAN_POINT('Ctrl Pts',(107.519067738522,-119.234602512151,
590.462296651429));
#267908=CARTESIAN_POINT('Ctrl Pts',(97.5309980386227,-126.9104585261,588.462296651429));
#267909=CARTESIAN_POINT('Ctrl Pts',(87.5429283387236,-134.586314540048,
586.462296651429));
#267910=CARTESIAN_POINT('Ctrl Pts',(76.4770599218141,-140.605189688823,
584.462296651429));
#267911=CARTESIAN_POINT('Ctrl Pts',(65.4111915049045,-146.624064837598,
582.462296651429));
#267912=CARTESIAN_POINT('Ctrl Pts',(53.5400027769202,-150.837754439537,
580.462296651429));
#267913=CARTESIAN_POINT('Ctrl Pts',(41.6688140489359,-155.051444041475,
578.462296651429));
#267914=CARTESIAN_POINT('Ctrl Pts',(29.2846130745768,-157.356193074143,
576.462296651429));
#267915=CARTESIAN_POINT('Ctrl Pts',(16.9004121002176,-159.660942106811,
574.462296651429));
#267916=CARTESIAN_POINT('Ctrl Pts',(4.30813900827854,-160.,572.462296651429));
#267917=CARTESIAN_POINT('Ctrl Pts',(-8.28413408366049,-160.339057893189,
570.462296651429));
#267918=CARTESIAN_POINT('Ctrl Pts',(-20.7744157382971,-158.704075916301,
568.462296651429));
#267919=CARTESIAN_POINT('Ctrl Pts',(-33.2646973929338,-157.069093939413,
566.462296651429));
#267920=CARTESIAN_POINT('Ctrl Pts',(-45.345435423063,-153.500330774912,
564.462296651429));
#267921=CARTESIAN_POINT('Ctrl Pts',(-57.4261734531921,-149.931567610412,
562.462296651429));
#267922=CARTESIAN_POINT('Ctrl Pts',(-68.7998999948409,-144.516898051455,
560.462296651429));
#267923=CARTESIAN_POINT('Ctrl Pts',(-80.1736265364897,-139.102228492498,
558.462296651429));
#267924=CARTESIAN_POINT('Ctrl Pts',(-90.5602826949688,-131.974979673884,
556.462296651429));
#267925=CARTESIAN_POINT('Ctrl Pts',(-100.946938853448,-124.84773085527,
554.462296651429));
#267926=CARTESIAN_POINT('Ctrl Pts',(-110.0907706828,-116.183399296896,552.462296651429));
#267927=CARTESIAN_POINT('Ctrl Pts',(-119.234602512151,-107.519067738522,
550.462296651429));
#267928=CARTESIAN_POINT('Ctrl Pts',(-126.9104585261,-97.5309980386227,548.462296651429));
#267929=CARTESIAN_POINT('Ctrl Pts',(-134.586314540048,-87.5429283387237,
546.462296651429));
#267930=CARTESIAN_POINT('Ctrl Pts',(-140.605189688823,-76.4770599218141,
544.462296651429));
#267931=CARTESIAN_POINT('Ctrl Pts',(-146.624064837598,-65.4111915049046,
542.462296651429));
#267932=CARTESIAN_POINT('Ctrl Pts',(-150.837754439537,-53.5400027769203,
540.462296651429));
#267933=CARTESIAN_POINT('Ctrl Pts',(-155.051444041475,-41.668814048936,
538.462296651429));
#267934=CARTESIAN_POINT('Ctrl Pts',(-157.356193074143,-29.2846130745768,
536.462296651429));
#267935=CARTESIAN_POINT('Ctrl Pts',(-159.394142202012,-18.3340187941084,
534.693818523023));
#267936=CARTESIAN_POINT('Ctrl Pts',(-159.895664541343,-7.20669984090296,
532.923108716584));
#267937=CARTESIAN_POINT('Ctrl Pts',(-130.,-4.30813900827845,692.462296651428));
#267938=CARTESIAN_POINT('Ctrl Pts',(-130.339057893189,5.92308287892195,
690.462296651428));
#267939=CARTESIAN_POINT('Ctrl Pts',(-129.073425698447,16.0813817870903,
688.462296651428));
#267940=CARTESIAN_POINT('Ctrl Pts',(-127.807793503705,26.2396806952586,
686.462296651429));
#267941=CARTESIAN_POINT('Ctrl Pts',(-124.968635286058,36.0749255918146,
684.462296651428));
#267942=CARTESIAN_POINT('Ctrl Pts',(-122.129477068411,45.9101704883706,
682.462296651429));
#267943=CARTESIAN_POINT('Ctrl Pts',(-117.786702325804,55.1801850026546,
680.462296651428));
#267944=CARTESIAN_POINT('Ctrl Pts',(-113.443927583196,64.4501995169386,
678.462296651428));
#267945=CARTESIAN_POINT('Ctrl Pts',(-107.704469842635,72.9267251261946,
676.462296651429));
#267946=CARTESIAN_POINT('Ctrl Pts',(-101.965012102074,81.4032507354507,
674.462296651429));
#267947=CARTESIAN_POINT('Ctrl Pts',(-94.9701958612992,88.8775672472032,
672.462296651428));
#267948=CARTESIAN_POINT('Ctrl Pts',(-87.9753796205245,96.3518837589558,
670.462296651429));
#267949=CARTESIAN_POINT('Ctrl Pts',(-79.8974404698484,102.639948694851,
668.462296651428));
#267950=CARTESIAN_POINT('Ctrl Pts',(-71.8195013191724,108.928013630747,
666.462296651428));
#267951=CARTESIAN_POINT('Ctrl Pts',(-62.8573449296276,113.874993963172,
664.462296651428));
#267952=CARTESIAN_POINT('Ctrl Pts',(-53.8951885400828,118.821974295598,
662.462296651429));
#267953=CARTESIAN_POINT('Ctrl Pts',(-44.2694929456717,122.306058950682,
660.462296651428));
#267954=CARTESIAN_POINT('Ctrl Pts',(-34.6437973512606,125.790143605767,
658.462296651428));
#267955=CARTESIAN_POINT('Ctrl Pts',(-24.5915791233697,127.725542856289,
656.462296651429));
#267956=CARTESIAN_POINT('Ctrl Pts',(-14.5393608954789,129.660942106811,
654.462296651428));
#267957=CARTESIAN_POINT('Ctrl Pts',(-4.30813900827846,130.,652.462296651428));
#267958=CARTESIAN_POINT('Ctrl Pts',(5.92308287892194,130.339057893189,650.462296651429));
#267959=CARTESIAN_POINT('Ctrl Pts',(16.0813817870903,129.073425698447,648.462296651428));
#267960=CARTESIAN_POINT('Ctrl Pts',(26.2396806952586,127.807793503705,646.462296651428));
#267961=CARTESIAN_POINT('Ctrl Pts',(36.0749255918146,124.968635286058,644.462296651428));
#267962=CARTESIAN_POINT('Ctrl Pts',(45.9101704883706,122.129477068411,642.462296651428));
#267963=CARTESIAN_POINT('Ctrl Pts',(55.1801850026546,117.786702325804,640.462296651428));
#267964=CARTESIAN_POINT('Ctrl Pts',(64.4501995169386,113.443927583196,638.462296651429));
#267965=CARTESIAN_POINT('Ctrl Pts',(72.9267251261946,107.704469842635,636.462296651428));
#267966=CARTESIAN_POINT('Ctrl Pts',(81.4032507354506,101.965012102074,634.462296651428));
#267967=CARTESIAN_POINT('Ctrl Pts',(88.8775672472032,94.9701958612992,632.462296651428));
#267968=CARTESIAN_POINT('Ctrl Pts',(96.3518837589558,87.9753796205245,630.462296651428));
#267969=CARTESIAN_POINT('Ctrl Pts',(102.639948694851,79.8974404698484,628.462296651428));
#267970=CARTESIAN_POINT('Ctrl Pts',(108.928013630747,71.8195013191724,626.462296651429));
#267971=CARTESIAN_POINT('Ctrl Pts',(113.874993963172,62.8573449296276,624.462296651428));
#267972=CARTESIAN_POINT('Ctrl Pts',(118.821974295598,53.8951885400829,622.462296651428));
#267973=CARTESIAN_POINT('Ctrl Pts',(122.306058950682,44.2694929456717,620.462296651428));
#267974=CARTESIAN_POINT('Ctrl Pts',(125.790143605767,34.6437973512606,618.462296651428));
#267975=CARTESIAN_POINT('Ctrl Pts',(127.725542856289,24.5915791233698,616.462296651428));
#267976=CARTESIAN_POINT('Ctrl Pts',(129.660942106811,14.5393608954789,614.462296651429));
#267977=CARTESIAN_POINT('Ctrl Pts',(130.,4.30813900827846,612.462296651428));
#267978=CARTESIAN_POINT('Ctrl Pts',(130.339057893189,-5.92308287892194,
610.462296651428));
#267979=CARTESIAN_POINT('Ctrl Pts',(129.073425698447,-16.0813817870903,
608.462296651428));
#267980=CARTESIAN_POINT('Ctrl Pts',(127.807793503705,-26.2396806952586,
606.462296651428));
#267981=CARTESIAN_POINT('Ctrl Pts',(124.968635286058,-36.0749255918146,
604.462296651428));
#267982=CARTESIAN_POINT('Ctrl Pts',(122.129477068411,-45.9101704883706,
602.462296651429));
#267983=CARTESIAN_POINT('Ctrl Pts',(117.786702325804,-55.1801850026546,
600.462296651428));
#267984=CARTESIAN_POINT('Ctrl Pts',(113.443927583196,-64.4501995169386,
598.462296651428));
#267985=CARTESIAN_POINT('Ctrl Pts',(107.704469842635,-72.9267251261946,
596.462296651428));
#267986=CARTESIAN_POINT('Ctrl Pts',(101.965012102074,-81.4032507354506,
594.462296651428));
#267987=CARTESIAN_POINT('Ctrl Pts',(94.9701958612992,-88.8775672472032,
592.462296651428));
#267988=CARTESIAN_POINT('Ctrl Pts',(87.9753796205246,-96.3518837589557,
590.462296651429));
#267989=CARTESIAN_POINT('Ctrl Pts',(79.8974404698484,-102.639948694851,
588.462296651428));
#267990=CARTESIAN_POINT('Ctrl Pts',(71.8195013191723,-108.928013630747,
586.462296651428));
#267991=CARTESIAN_POINT('Ctrl Pts',(62.8573449296276,-113.874993963172,
584.462296651428));
#267992=CARTESIAN_POINT('Ctrl Pts',(53.8951885400829,-118.821974295598,
582.462296651428));
#267993=CARTESIAN_POINT('Ctrl Pts',(44.2694929456717,-122.306058950682,
580.462296651428));
#267994=CARTESIAN_POINT('Ctrl Pts',(34.6437973512606,-125.790143605767,
578.462296651429));
#267995=CARTESIAN_POINT('Ctrl Pts',(24.5915791233698,-127.725542856289,
576.462296651428));
#267996=CARTESIAN_POINT('Ctrl Pts',(14.5393608954789,-129.660942106811,
574.462296651428));
#267997=CARTESIAN_POINT('Ctrl Pts',(4.30813900827847,-130.,572.462296651428));
#267998=CARTESIAN_POINT('Ctrl Pts',(-5.92308287892199,-130.339057893189,
570.462296651428));
#267999=CARTESIAN_POINT('Ctrl Pts',(-16.0813817870903,-129.073425698447,
568.462296651428));
#268000=CARTESIAN_POINT('Ctrl Pts',(-26.2396806952585,-127.807793503705,
566.462296651429));
#268001=CARTESIAN_POINT('Ctrl Pts',(-36.0749255918146,-124.968635286058,
564.462296651428));
#268002=CARTESIAN_POINT('Ctrl Pts',(-45.9101704883706,-122.129477068411,
562.462296651428));
#268003=CARTESIAN_POINT('Ctrl Pts',(-55.1801850026546,-117.786702325804,
560.462296651428));
#268004=CARTESIAN_POINT('Ctrl Pts',(-64.4501995169385,-113.443927583197,
558.462296651429));
#268005=CARTESIAN_POINT('Ctrl Pts',(-72.9267251261946,-107.704469842635,
556.462296651428));
#268006=CARTESIAN_POINT('Ctrl Pts',(-81.4032507354507,-101.965012102074,
554.462296651429));
#268007=CARTESIAN_POINT('Ctrl Pts',(-88.8775672472032,-94.9701958612992,
552.462296651428));
#268008=CARTESIAN_POINT('Ctrl Pts',(-96.3518837589557,-87.9753796205246,
550.462296651428));
#268009=CARTESIAN_POINT('Ctrl Pts',(-102.639948694851,-79.8974404698484,
548.462296651428));
#268010=CARTESIAN_POINT('Ctrl Pts',(-108.928013630747,-71.8195013191723,
546.462296651429));
#268011=CARTESIAN_POINT('Ctrl Pts',(-113.874993963172,-62.8573449296276,
544.462296651428));
#268012=CARTESIAN_POINT('Ctrl Pts',(-118.821974295598,-53.8951885400829,
542.462296651429));
#268013=CARTESIAN_POINT('Ctrl Pts',(-122.306058950682,-44.2694929456718,
540.462296651428));
#268014=CARTESIAN_POINT('Ctrl Pts',(-125.790143605767,-34.6437973512606,
538.462296651428));
#268015=CARTESIAN_POINT('Ctrl Pts',(-127.725542856289,-24.5915791233698,
536.462296651428));
#268016=CARTESIAN_POINT('Ctrl Pts',(-129.660942106811,-14.5393608954789,
534.462296651429));
#268017=CARTESIAN_POINT('Ctrl Pts',(-130.,-4.30813900827845,532.462296651428));
#268018=CARTESIAN_POINT('Ctrl Pts',(-160.,-4.30813900827851,692.462296651429));
#268019=CARTESIAN_POINT('Ctrl Pts',(-160.339057893189,8.28413408366045,
690.462296651429));
#268020=CARTESIAN_POINT('Ctrl Pts',(-158.704075916301,20.7744157382972,
688.462296651429));
#268021=CARTESIAN_POINT('Ctrl Pts',(-157.069093939413,33.2646973929339,
686.462296651429));
#268022=CARTESIAN_POINT('Ctrl Pts',(-153.500330774912,45.345435423063,684.462296651429));
#268023=CARTESIAN_POINT('Ctrl Pts',(-149.931567610412,57.4261734531921,
682.462296651429));
#268024=CARTESIAN_POINT('Ctrl Pts',(-144.516898051455,68.7998999948409,
680.462296651429));
#268025=CARTESIAN_POINT('Ctrl Pts',(-139.102228492498,80.1736265364898,
678.462296651429));
#268026=CARTESIAN_POINT('Ctrl Pts',(-131.974979673884,90.5602826949688,
676.462296651429));
#268027=CARTESIAN_POINT('Ctrl Pts',(-124.84773085527,100.946938853448,674.462296651429));
#268028=CARTESIAN_POINT('Ctrl Pts',(-116.183399296896,110.0907706828,672.462296651429));
#268029=CARTESIAN_POINT('Ctrl Pts',(-107.519067738522,119.234602512151,
670.462296651429));
#268030=CARTESIAN_POINT('Ctrl Pts',(-97.5309980386227,126.9104585261,668.462296651429));
#268031=CARTESIAN_POINT('Ctrl Pts',(-87.5429283387237,134.586314540048,
666.462296651429));
#268032=CARTESIAN_POINT('Ctrl Pts',(-76.4770599218141,140.605189688823,
664.462296651429));
#268033=CARTESIAN_POINT('Ctrl Pts',(-65.4111915049045,146.624064837598,
662.462296651429));
#268034=CARTESIAN_POINT('Ctrl Pts',(-53.5400027769202,150.837754439537,
660.462296651429));
#268035=CARTESIAN_POINT('Ctrl Pts',(-41.668814048936,155.051444041475,658.462296651429));
#268036=CARTESIAN_POINT('Ctrl Pts',(-29.2846130745767,157.356193074143,
656.462296651429));
#268037=CARTESIAN_POINT('Ctrl Pts',(-16.9004121002175,159.660942106811,
654.462296651428));
#268038=CARTESIAN_POINT('Ctrl Pts',(-4.30813900827852,160.,652.462296651429));
#268039=CARTESIAN_POINT('Ctrl Pts',(8.28413408366043,160.339057893189,650.462296651429));
#268040=CARTESIAN_POINT('Ctrl Pts',(20.7744157382972,158.704075916301,648.462296651428));
#268041=CARTESIAN_POINT('Ctrl Pts',(33.2646973929339,157.069093939413,646.462296651429));
#268042=CARTESIAN_POINT('Ctrl Pts',(45.345435423063,153.500330774912,644.462296651428));
#268043=CARTESIAN_POINT('Ctrl Pts',(57.4261734531921,149.931567610412,642.462296651428));
#268044=CARTESIAN_POINT('Ctrl Pts',(68.7998999948409,144.516898051455,640.462296651428));
#268045=CARTESIAN_POINT('Ctrl Pts',(80.1736265364898,139.102228492498,638.462296651429));
#268046=CARTESIAN_POINT('Ctrl Pts',(90.5602826949688,131.974979673884,636.462296651428));
#268047=CARTESIAN_POINT('Ctrl Pts',(100.946938853448,124.84773085527,634.462296651428));
#268048=CARTESIAN_POINT('Ctrl Pts',(110.0907706828,116.183399296896,632.462296651429));
#268049=CARTESIAN_POINT('Ctrl Pts',(119.234602512151,107.519067738522,630.462296651429));
#268050=CARTESIAN_POINT('Ctrl Pts',(126.9104585261,97.5309980386227,628.462296651429));
#268051=CARTESIAN_POINT('Ctrl Pts',(134.586314540048,87.5429283387237,626.462296651429));
#268052=CARTESIAN_POINT('Ctrl Pts',(140.605189688823,76.4770599218141,624.462296651429));
#268053=CARTESIAN_POINT('Ctrl Pts',(146.624064837598,65.4111915049045,622.462296651429));
#268054=CARTESIAN_POINT('Ctrl Pts',(150.837754439537,53.5400027769202,620.462296651429));
#268055=CARTESIAN_POINT('Ctrl Pts',(155.051444041475,41.668814048936,618.462296651429));
#268056=CARTESIAN_POINT('Ctrl Pts',(157.356193074143,29.2846130745767,616.462296651429));
#268057=CARTESIAN_POINT('Ctrl Pts',(159.660942106811,16.9004121002175,614.462296651429));
#268058=CARTESIAN_POINT('Ctrl Pts',(160.,4.30813900827853,612.462296651429));
#268059=CARTESIAN_POINT('Ctrl Pts',(160.339057893189,-8.28413408366043,
610.462296651429));
#268060=CARTESIAN_POINT('Ctrl Pts',(158.704075916301,-20.7744157382971,
608.462296651429));
#268061=CARTESIAN_POINT('Ctrl Pts',(157.069093939413,-33.2646973929339,
606.462296651429));
#268062=CARTESIAN_POINT('Ctrl Pts',(153.500330774912,-45.345435423063,604.462296651429));
#268063=CARTESIAN_POINT('Ctrl Pts',(149.931567610412,-57.4261734531921,
602.462296651429));
#268064=CARTESIAN_POINT('Ctrl Pts',(144.516898051455,-68.7998999948409,
600.462296651429));
#268065=CARTESIAN_POINT('Ctrl Pts',(139.102228492498,-80.1736265364898,
598.462296651429));
#268066=CARTESIAN_POINT('Ctrl Pts',(131.974979673884,-90.5602826949688,
596.462296651429));
#268067=CARTESIAN_POINT('Ctrl Pts',(124.84773085527,-100.946938853448,594.462296651428));
#268068=CARTESIAN_POINT('Ctrl Pts',(116.183399296896,-110.0907706828,592.462296651429));
#268069=CARTESIAN_POINT('Ctrl Pts',(107.519067738522,-119.234602512151,
590.462296651429));
#268070=CARTESIAN_POINT('Ctrl Pts',(97.5309980386227,-126.9104585261,588.462296651429));
#268071=CARTESIAN_POINT('Ctrl Pts',(87.5429283387236,-134.586314540048,
586.462296651429));
#268072=CARTESIAN_POINT('Ctrl Pts',(76.4770599218141,-140.605189688823,
584.462296651429));
#268073=CARTESIAN_POINT('Ctrl Pts',(65.4111915049046,-146.624064837598,
582.462296651428));
#268074=CARTESIAN_POINT('Ctrl Pts',(53.5400027769202,-150.837754439537,
580.462296651429));
#268075=CARTESIAN_POINT('Ctrl Pts',(41.6688140489359,-155.051444041475,
578.462296651429));
#268076=CARTESIAN_POINT('Ctrl Pts',(29.2846130745768,-157.356193074143,
576.462296651429));
#268077=CARTESIAN_POINT('Ctrl Pts',(16.9004121002176,-159.660942106811,
574.462296651429));
#268078=CARTESIAN_POINT('Ctrl Pts',(4.30813900827854,-160.,572.462296651429));
#268079=CARTESIAN_POINT('Ctrl Pts',(-8.28413408366049,-160.339057893189,
570.462296651428));
#268080=CARTESIAN_POINT('Ctrl Pts',(-20.7744157382971,-158.704075916301,
568.462296651429));
#268081=CARTESIAN_POINT('Ctrl Pts',(-33.2646973929338,-157.069093939413,
566.462296651429));
#268082=CARTESIAN_POINT('Ctrl Pts',(-45.345435423063,-153.500330774912,
564.462296651429));
#268083=CARTESIAN_POINT('Ctrl Pts',(-57.4261734531921,-149.931567610412,
562.462296651429));
#268084=CARTESIAN_POINT('Ctrl Pts',(-68.7998999948409,-144.516898051455,
560.462296651429));
#268085=CARTESIAN_POINT('Ctrl Pts',(-80.1736265364897,-139.102228492498,
558.462296651429));
#268086=CARTESIAN_POINT('Ctrl Pts',(-90.5602826949688,-131.974979673884,
556.462296651429));
#268087=CARTESIAN_POINT('Ctrl Pts',(-100.946938853448,-124.84773085527,
554.462296651429));
#268088=CARTESIAN_POINT('Ctrl Pts',(-110.0907706828,-116.183399296896,552.462296651429));
#268089=CARTESIAN_POINT('Ctrl Pts',(-119.234602512151,-107.519067738522,
550.462296651429));
#268090=CARTESIAN_POINT('Ctrl Pts',(-126.9104585261,-97.5309980386227,548.462296651429));
#268091=CARTESIAN_POINT('Ctrl Pts',(-134.586314540048,-87.5429283387236,
546.462296651429));
#268092=CARTESIAN_POINT('Ctrl Pts',(-140.605189688823,-76.4770599218141,
544.462296651429));
#268093=CARTESIAN_POINT('Ctrl Pts',(-146.624064837598,-65.4111915049046,
542.462296651429));
#268094=CARTESIAN_POINT('Ctrl Pts',(-150.837754439537,-53.5400027769203,
540.462296651429));
#268095=CARTESIAN_POINT('Ctrl Pts',(-155.051444041475,-41.668814048936,
538.462296651429));
#268096=CARTESIAN_POINT('Ctrl Pts',(-157.356193074143,-29.2846130745768,
536.462296651429));
#268097=CARTESIAN_POINT('Ctrl Pts',(-159.660942106811,-16.9004121002176,
534.462296651429));
#268098=CARTESIAN_POINT('Ctrl Pts',(-160.,-4.30813900827851,532.462296651429));
#268099=CARTESIAN_POINT('Origin',(-160.,3.64291929955129E-14,535.));
#268100=CARTESIAN_POINT('',(-160.,1.56720635279146E-14,535.));
#268101=CARTESIAN_POINT('',(-160.,-4.30813900827827,538.90811221526));
#268102=CARTESIAN_POINT('Ctrl Pts',(-160.,-2.35367281220533E-13,535.));
#268103=CARTESIAN_POINT('Ctrl Pts',(-160.,-0.0199151703951082,535.01805734453));
#268104=CARTESIAN_POINT('Ctrl Pts',(-160.,-0.039830432424492,535.036114587998));
#268105=CARTESIAN_POINT('Ctrl Pts',(-160.,-0.059745511185169,535.05417203359));
#268106=CARTESIAN_POINT('Ctrl Pts',(-160.,-1.4761797871856,536.338484547738));
#268107=CARTESIAN_POINT('Ctrl Pts',(-160.,-2.89215276710114,537.623305748502));
#268108=CARTESIAN_POINT('Ctrl Pts',(-160.,-4.30813900827838,538.90811221526));
#268109=CARTESIAN_POINT('',(-160.,-4.30813900827851,532.462296651429));
#268110=CARTESIAN_POINT('',(-160.,-4.21537804662364E-13,535.));
#268111=CARTESIAN_POINT('',(-160.,4.30813900827783,531.091887784741));
#268112=CARTESIAN_POINT('Ctrl Pts',(-160.,-4.30813900827851,532.462296651429));
#268113=CARTESIAN_POINT('Ctrl Pts',(-160.,-1.43594781991725,532.006113535419));
#268114=CARTESIAN_POINT('Ctrl Pts',(-160.,1.43604209808292,531.548664093541));
#268115=CARTESIAN_POINT('Ctrl Pts',(-160.,4.30813900827783,531.091887784741));
#268116=CARTESIAN_POINT('Ctrl Pts',(-160.,4.30813900827787,531.091887784741));
#268117=CARTESIAN_POINT('Ctrl Pts',(-160.,2.89215276710099,532.376694251499));
#268118=CARTESIAN_POINT('Ctrl Pts',(-160.,1.47617978720989,533.66151545229));
#268119=CARTESIAN_POINT('Ctrl Pts',(-160.,0.0597455111844823,534.945827966411));
#268120=CARTESIAN_POINT('Ctrl Pts',(-160.,0.0398304324235108,534.963885412002));
#268121=CARTESIAN_POINT('Ctrl Pts',(-160.,0.019915170394957,534.981942655471));
#268122=CARTESIAN_POINT('Ctrl Pts',(-160.,1.72084568816899E-14,535.000000000001));
#268123=CARTESIAN_POINT('',(-160.,4.30813900827767,537.537703348572));
#268124=CARTESIAN_POINT('',(-160.,-4.21537804662364E-13,535.));
#268125=CARTESIAN_POINT('Ctrl Pts',(-160.,-4.30813900827827,538.90811221526));
#268126=CARTESIAN_POINT('Ctrl Pts',(-160.,-1.43604209806711,538.451335906457));
#268127=CARTESIAN_POINT('Ctrl Pts',(-160.,1.43594781992473,537.99388646458));
#268128=CARTESIAN_POINT('Ctrl Pts',(-160.,4.30813900827767,537.537703348572));
#268129=CARTESIAN_POINT('Ctrl Pts',(-160.,-4.30813900827851,692.462296651429));
#268130=CARTESIAN_POINT('Ctrl Pts',(-160.339057893189,8.28413408366045,
690.462296651429));
#268131=CARTESIAN_POINT('Ctrl Pts',(-158.704075916301,20.7744157382972,
688.462296651429));
#268132=CARTESIAN_POINT('Ctrl Pts',(-157.069093939413,33.2646973929339,
686.462296651429));
#268133=CARTESIAN_POINT('Ctrl Pts',(-153.500330774912,45.345435423063,684.462296651429));
#268134=CARTESIAN_POINT('Ctrl Pts',(-149.931567610412,57.4261734531921,
682.462296651429));
#268135=CARTESIAN_POINT('Ctrl Pts',(-144.516898051455,68.7998999948409,
680.462296651429));
#268136=CARTESIAN_POINT('Ctrl Pts',(-139.102228492498,80.1736265364898,
678.462296651429));
#268137=CARTESIAN_POINT('Ctrl Pts',(-131.974979673884,90.5602826949688,
676.462296651429));
#268138=CARTESIAN_POINT('Ctrl Pts',(-124.84773085527,100.946938853448,674.462296651429));
#268139=CARTESIAN_POINT('Ctrl Pts',(-116.183399296896,110.0907706828,672.462296651429));
#268140=CARTESIAN_POINT('Ctrl Pts',(-107.519067738522,119.234602512151,
670.462296651429));
#268141=CARTESIAN_POINT('Ctrl Pts',(-97.5309980386227,126.9104585261,668.462296651429));
#268142=CARTESIAN_POINT('Ctrl Pts',(-87.5429283387237,134.586314540048,
666.462296651429));
#268143=CARTESIAN_POINT('Ctrl Pts',(-76.4770599218141,140.605189688823,
664.462296651429));
#268144=CARTESIAN_POINT('Ctrl Pts',(-65.4111915049045,146.624064837598,
662.462296651429));
#268145=CARTESIAN_POINT('Ctrl Pts',(-53.5400027769202,150.837754439537,
660.462296651429));
#268146=CARTESIAN_POINT('Ctrl Pts',(-41.668814048936,155.051444041475,658.462296651429));
#268147=CARTESIAN_POINT('Ctrl Pts',(-29.2846130745767,157.356193074143,
656.462296651429));
#268148=CARTESIAN_POINT('Ctrl Pts',(-16.9004121002175,159.660942106811,
654.462296651428));
#268149=CARTESIAN_POINT('Ctrl Pts',(-4.30813900827852,160.,652.462296651429));
#268150=CARTESIAN_POINT('Ctrl Pts',(8.28413408366043,160.339057893189,650.462296651429));
#268151=CARTESIAN_POINT('Ctrl Pts',(20.7744157382972,158.704075916301,648.462296651428));
#268152=CARTESIAN_POINT('Ctrl Pts',(33.2646973929339,157.069093939413,646.462296651429));
#268153=CARTESIAN_POINT('Ctrl Pts',(45.345435423063,153.500330774912,644.462296651428));
#268154=CARTESIAN_POINT('Ctrl Pts',(57.4261734531921,149.931567610412,642.462296651428));
#268155=CARTESIAN_POINT('Ctrl Pts',(68.7998999948409,144.516898051455,640.462296651428));
#268156=CARTESIAN_POINT('Ctrl Pts',(80.1736265364898,139.102228492498,638.462296651429));
#268157=CARTESIAN_POINT('Ctrl Pts',(90.5602826949688,131.974979673884,636.462296651428));
#268158=CARTESIAN_POINT('Ctrl Pts',(100.946938853448,124.84773085527,634.462296651428));
#268159=CARTESIAN_POINT('Ctrl Pts',(110.0907706828,116.183399296896,632.462296651429));
#268160=CARTESIAN_POINT('Ctrl Pts',(119.234602512151,107.519067738522,630.462296651429));
#268161=CARTESIAN_POINT('Ctrl Pts',(126.9104585261,97.5309980386227,628.462296651429));
#268162=CARTESIAN_POINT('Ctrl Pts',(134.586314540048,87.5429283387237,626.462296651429));
#268163=CARTESIAN_POINT('Ctrl Pts',(140.605189688823,76.4770599218141,624.462296651429));
#268164=CARTESIAN_POINT('Ctrl Pts',(146.624064837598,65.4111915049045,622.462296651429));
#268165=CARTESIAN_POINT('Ctrl Pts',(150.837754439537,53.5400027769202,620.462296651429));
#268166=CARTESIAN_POINT('Ctrl Pts',(155.051444041475,41.668814048936,618.462296651429));
#268167=CARTESIAN_POINT('Ctrl Pts',(157.356193074143,29.2846130745767,616.462296651429));
#268168=CARTESIAN_POINT('Ctrl Pts',(159.660942106811,16.9004121002175,614.462296651429));
#268169=CARTESIAN_POINT('Ctrl Pts',(160.,4.30813900827853,612.462296651429));
#268170=CARTESIAN_POINT('Ctrl Pts',(160.339057893189,-8.28413408366043,
610.462296651429));
#268171=CARTESIAN_POINT('Ctrl Pts',(158.704075916301,-20.7744157382971,
608.462296651429));
#268172=CARTESIAN_POINT('Ctrl Pts',(157.069093939413,-33.2646973929339,
606.462296651429));
#268173=CARTESIAN_POINT('Ctrl Pts',(153.500330774912,-45.345435423063,604.462296651429));
#268174=CARTESIAN_POINT('Ctrl Pts',(149.931567610412,-57.4261734531921,
602.462296651429));
#268175=CARTESIAN_POINT('Ctrl Pts',(144.516898051455,-68.7998999948409,
600.462296651429));
#268176=CARTESIAN_POINT('Ctrl Pts',(139.102228492498,-80.1736265364898,
598.462296651429));
#268177=CARTESIAN_POINT('Ctrl Pts',(131.974979673884,-90.5602826949688,
596.462296651429));
#268178=CARTESIAN_POINT('Ctrl Pts',(124.84773085527,-100.946938853448,594.462296651428));
#268179=CARTESIAN_POINT('Ctrl Pts',(116.183399296896,-110.0907706828,592.462296651429));
#268180=CARTESIAN_POINT('Ctrl Pts',(107.519067738522,-119.234602512151,
590.462296651429));
#268181=CARTESIAN_POINT('Ctrl Pts',(97.5309980386227,-126.9104585261,588.462296651429));
#268182=CARTESIAN_POINT('Ctrl Pts',(87.5429283387236,-134.586314540048,
586.462296651429));
#268183=CARTESIAN_POINT('Ctrl Pts',(76.4770599218141,-140.605189688823,
584.462296651429));
#268184=CARTESIAN_POINT('Ctrl Pts',(65.4111915049046,-146.624064837598,
582.462296651428));
#268185=CARTESIAN_POINT('Ctrl Pts',(53.5400027769202,-150.837754439537,
580.462296651429));
#268186=CARTESIAN_POINT('Ctrl Pts',(41.6688140489359,-155.051444041475,
578.462296651429));
#268187=CARTESIAN_POINT('Ctrl Pts',(29.2846130745768,-157.356193074143,
576.462296651429));
#268188=CARTESIAN_POINT('Ctrl Pts',(16.9004121002176,-159.660942106811,
574.462296651429));
#268189=CARTESIAN_POINT('Ctrl Pts',(4.30813900827854,-160.,572.462296651429));
#268190=CARTESIAN_POINT('Ctrl Pts',(-8.28413408366049,-160.339057893189,
570.462296651428));
#268191=CARTESIAN_POINT('Ctrl Pts',(-20.7744157382971,-158.704075916301,
568.462296651429));
#268192=CARTESIAN_POINT('Ctrl Pts',(-33.2646973929338,-157.069093939413,
566.462296651429));
#268193=CARTESIAN_POINT('Ctrl Pts',(-45.345435423063,-153.500330774912,
564.462296651429));
#268194=CARTESIAN_POINT('Ctrl Pts',(-57.4261734531921,-149.931567610412,
562.462296651429));
#268195=CARTESIAN_POINT('Ctrl Pts',(-68.7998999948409,-144.516898051455,
560.462296651429));
#268196=CARTESIAN_POINT('Ctrl Pts',(-80.1736265364897,-139.102228492498,
558.462296651429));
#268197=CARTESIAN_POINT('Ctrl Pts',(-90.5602826949688,-131.974979673884,
556.462296651429));
#268198=CARTESIAN_POINT('Ctrl Pts',(-100.946938853448,-124.84773085527,
554.462296651429));
#268199=CARTESIAN_POINT('Ctrl Pts',(-110.0907706828,-116.183399296896,552.462296651429));
#268200=CARTESIAN_POINT('Ctrl Pts',(-119.234602512151,-107.519067738522,
550.462296651429));
#268201=CARTESIAN_POINT('Ctrl Pts',(-126.9104585261,-97.5309980386227,548.462296651429));
#268202=CARTESIAN_POINT('Ctrl Pts',(-134.586314540048,-87.5429283387236,
546.462296651429));
#268203=CARTESIAN_POINT('Ctrl Pts',(-140.605189688823,-76.4770599218141,
544.462296651429));
#268204=CARTESIAN_POINT('Ctrl Pts',(-146.624064837598,-65.4111915049046,
542.462296651429));
#268205=CARTESIAN_POINT('Ctrl Pts',(-150.837754439537,-53.5400027769203,
540.462296651429));
#268206=CARTESIAN_POINT('Ctrl Pts',(-155.051444041475,-41.668814048936,
538.462296651429));
#268207=CARTESIAN_POINT('Ctrl Pts',(-157.356193074143,-29.2846130745768,
536.462296651429));
#268208=CARTESIAN_POINT('Ctrl Pts',(-159.660942106811,-16.9004121002176,
534.462296651429));
#268209=CARTESIAN_POINT('Ctrl Pts',(-160.,-4.30813900827851,532.462296651429));
#268210=CARTESIAN_POINT('Ctrl Pts',(-160.,4.30813900827767,697.537703348572));
#268211=CARTESIAN_POINT('Ctrl Pts',(-159.660942106811,16.9004121002166,
695.537703348572));
#268212=CARTESIAN_POINT('Ctrl Pts',(-157.356193074143,29.2846130745759,
693.537703348572));
#268213=CARTESIAN_POINT('Ctrl Pts',(-155.051444041476,41.6688140489352,
691.537703348572));
#268214=CARTESIAN_POINT('Ctrl Pts',(-150.837754439537,53.5400027769194,
689.537703348572));
#268215=CARTESIAN_POINT('Ctrl Pts',(-146.624064837599,65.4111915049037,
687.537703348572));
#268216=CARTESIAN_POINT('Ctrl Pts',(-140.605189688823,76.4770599218133,
685.537703348572));
#268217=CARTESIAN_POINT('Ctrl Pts',(-134.586314540048,87.542928338723,683.537703348572));
#268218=CARTESIAN_POINT('Ctrl Pts',(-126.9104585261,97.530998038622,681.537703348572));
#268219=CARTESIAN_POINT('Ctrl Pts',(-119.234602512152,107.519067738521,
679.537703348572));
#268220=CARTESIAN_POINT('Ctrl Pts',(-110.0907706828,116.183399296895,677.537703348572));
#268221=CARTESIAN_POINT('Ctrl Pts',(-100.946938853448,124.847730855269,
675.537703348572));
#268222=CARTESIAN_POINT('Ctrl Pts',(-90.5602826949695,131.974979673883,
673.537703348572));
#268223=CARTESIAN_POINT('Ctrl Pts',(-80.1736265364906,139.102228492497,
671.537703348572));
#268224=CARTESIAN_POINT('Ctrl Pts',(-68.7998999948417,144.516898051454,
669.537703348572));
#268225=CARTESIAN_POINT('Ctrl Pts',(-57.4261734531929,149.931567610411,
667.537703348572));
#268226=CARTESIAN_POINT('Ctrl Pts',(-45.3454354230638,153.500330774912,
665.537703348572));
#268227=CARTESIAN_POINT('Ctrl Pts',(-33.2646973929347,157.069093939413,
663.537703348572));
#268228=CARTESIAN_POINT('Ctrl Pts',(-20.774415738298,158.704075916301,661.537703348572));
#268229=CARTESIAN_POINT('Ctrl Pts',(-8.28413408366129,160.339057893189,
659.537703348572));
#268230=CARTESIAN_POINT('Ctrl Pts',(4.30813900827766,160.,657.537703348572));
#268231=CARTESIAN_POINT('Ctrl Pts',(16.9004121002166,159.660942106811,655.537703348572));
#268232=CARTESIAN_POINT('Ctrl Pts',(29.2846130745759,157.356193074143,653.537703348572));
#268233=CARTESIAN_POINT('Ctrl Pts',(41.6688140489352,155.051444041476,651.537703348572));
#268234=CARTESIAN_POINT('Ctrl Pts',(53.5400027769194,150.837754439537,649.537703348572));
#268235=CARTESIAN_POINT('Ctrl Pts',(65.4111915049037,146.624064837599,647.537703348572));
#268236=CARTESIAN_POINT('Ctrl Pts',(76.4770599218133,140.605189688823,645.537703348572));
#268237=CARTESIAN_POINT('Ctrl Pts',(87.542928338723,134.586314540048,643.537703348572));
#268238=CARTESIAN_POINT('Ctrl Pts',(97.530998038622,126.9104585261,641.537703348572));
#268239=CARTESIAN_POINT('Ctrl Pts',(107.519067738521,119.234602512152,639.537703348572));
#268240=CARTESIAN_POINT('Ctrl Pts',(116.183399296895,110.0907706828,637.537703348572));
#268241=CARTESIAN_POINT('Ctrl Pts',(124.847730855269,100.946938853448,635.537703348572));
#268242=CARTESIAN_POINT('Ctrl Pts',(131.974979673883,90.5602826949695,633.537703348572));
#268243=CARTESIAN_POINT('Ctrl Pts',(139.102228492497,80.1736265364906,631.537703348572));
#268244=CARTESIAN_POINT('Ctrl Pts',(144.516898051454,68.7998999948417,629.537703348572));
#268245=CARTESIAN_POINT('Ctrl Pts',(149.931567610411,57.4261734531929,627.537703348572));
#268246=CARTESIAN_POINT('Ctrl Pts',(153.500330774912,45.3454354230638,625.537703348572));
#268247=CARTESIAN_POINT('Ctrl Pts',(157.069093939413,33.2646973929347,623.537703348572));
#268248=CARTESIAN_POINT('Ctrl Pts',(158.704075916301,20.774415738298,621.537703348572));
#268249=CARTESIAN_POINT('Ctrl Pts',(160.339057893189,8.28413408366131,619.537703348572));
#268250=CARTESIAN_POINT('Ctrl Pts',(160.,-4.30813900827765,617.537703348572));
#268251=CARTESIAN_POINT('Ctrl Pts',(159.660942106811,-16.9004121002166,
615.537703348572));
#268252=CARTESIAN_POINT('Ctrl Pts',(157.356193074143,-29.2846130745759,
613.537703348572));
#268253=CARTESIAN_POINT('Ctrl Pts',(155.051444041476,-41.6688140489352,
611.537703348572));
#268254=CARTESIAN_POINT('Ctrl Pts',(150.837754439537,-53.5400027769194,
609.537703348572));
#268255=CARTESIAN_POINT('Ctrl Pts',(146.624064837599,-65.4111915049036,
607.537703348572));
#268256=CARTESIAN_POINT('Ctrl Pts',(140.605189688823,-76.4770599218133,
605.537703348572));
#268257=CARTESIAN_POINT('Ctrl Pts',(134.586314540048,-87.5429283387229,
603.537703348572));
#268258=CARTESIAN_POINT('Ctrl Pts',(126.9104585261,-97.530998038622,601.537703348572));
#268259=CARTESIAN_POINT('Ctrl Pts',(119.234602512152,-107.519067738521,
599.537703348572));
#268260=CARTESIAN_POINT('Ctrl Pts',(110.0907706828,-116.183399296895,597.537703348572));
#268261=CARTESIAN_POINT('Ctrl Pts',(100.946938853448,-124.847730855269,
595.537703348572));
#268262=CARTESIAN_POINT('Ctrl Pts',(90.5602826949695,-131.974979673883,
593.537703348572));
#268263=CARTESIAN_POINT('Ctrl Pts',(80.1736265364905,-139.102228492497,
591.537703348572));
#268264=CARTESIAN_POINT('Ctrl Pts',(68.7998999948417,-144.516898051454,
589.537703348572));
#268265=CARTESIAN_POINT('Ctrl Pts',(57.426173453193,-149.931567610411,587.537703348572));
#268266=CARTESIAN_POINT('Ctrl Pts',(45.3454354230638,-153.500330774912,
585.537703348572));
#268267=CARTESIAN_POINT('Ctrl Pts',(33.2646973929347,-157.069093939413,
583.537703348572));
#268268=CARTESIAN_POINT('Ctrl Pts',(20.774415738298,-158.704075916301,581.537703348572));
#268269=CARTESIAN_POINT('Ctrl Pts',(8.28413408366139,-160.339057893189,
579.537703348572));
#268270=CARTESIAN_POINT('Ctrl Pts',(-4.30813900827764,-160.,577.537703348572));
#268271=CARTESIAN_POINT('Ctrl Pts',(-16.9004121002167,-159.660942106811,
575.537703348572));
#268272=CARTESIAN_POINT('Ctrl Pts',(-29.2846130745759,-157.356193074143,
573.537703348572));
#268273=CARTESIAN_POINT('Ctrl Pts',(-41.6688140489351,-155.051444041476,
571.537703348572));
#268274=CARTESIAN_POINT('Ctrl Pts',(-53.5400027769194,-150.837754439537,
569.537703348572));
#268275=CARTESIAN_POINT('Ctrl Pts',(-65.4111915049037,-146.624064837599,
567.537703348572));
#268276=CARTESIAN_POINT('Ctrl Pts',(-76.4770599218133,-140.605189688823,
565.537703348572));
#268277=CARTESIAN_POINT('Ctrl Pts',(-87.5429283387229,-134.586314540048,
563.537703348572));
#268278=CARTESIAN_POINT('Ctrl Pts',(-97.530998038622,-126.9104585261,561.537703348572));
#268279=CARTESIAN_POINT('Ctrl Pts',(-107.519067738521,-119.234602512152,
559.537703348572));
#268280=CARTESIAN_POINT('Ctrl Pts',(-116.183399296895,-110.0907706828,557.537703348572));
#268281=CARTESIAN_POINT('Ctrl Pts',(-124.847730855269,-100.946938853448,
555.537703348572));
#268282=CARTESIAN_POINT('Ctrl Pts',(-131.974979673883,-90.5602826949695,
553.537703348572));
#268283=CARTESIAN_POINT('Ctrl Pts',(-139.102228492497,-80.1736265364905,
551.537703348572));
#268284=CARTESIAN_POINT('Ctrl Pts',(-144.516898051454,-68.7998999948417,
549.537703348572));
#268285=CARTESIAN_POINT('Ctrl Pts',(-149.931567610411,-57.426173453193,
547.537703348572));
#268286=CARTESIAN_POINT('Ctrl Pts',(-153.500330774912,-45.3454354230638,
545.537703348572));
#268287=CARTESIAN_POINT('Ctrl Pts',(-157.069093939413,-33.2646973929347,
543.537703348572));
#268288=CARTESIAN_POINT('Ctrl Pts',(-158.704075916301,-20.774415738298,
541.537703348572));
#268289=CARTESIAN_POINT('Ctrl Pts',(-160.339057893189,-8.2841340836614,
539.537703348572));
#268290=CARTESIAN_POINT('Ctrl Pts',(-160.,4.30813900827767,537.537703348572));
#268291=CARTESIAN_POINT('Origin',(4.03737035481473,0.209103844008918,539.53762260761));
#268292=CARTESIAN_POINT('Ctrl Pts',(-160.,4.30813900827767,697.537703348572));
#268293=CARTESIAN_POINT('Ctrl Pts',(-159.660942106811,16.9004121002166,
695.537703348572));
#268294=CARTESIAN_POINT('Ctrl Pts',(-157.356193074143,29.2846130745759,
693.537703348572));
#268295=CARTESIAN_POINT('Ctrl Pts',(-155.051444041476,41.6688140489352,
691.537703348572));
#268296=CARTESIAN_POINT('Ctrl Pts',(-150.837754439537,53.5400027769194,
689.537703348572));
#268297=CARTESIAN_POINT('Ctrl Pts',(-146.624064837599,65.4111915049037,
687.537703348572));
#268298=CARTESIAN_POINT('Ctrl Pts',(-140.605189688823,76.4770599218133,
685.537703348572));
#268299=CARTESIAN_POINT('Ctrl Pts',(-134.586314540048,87.542928338723,683.537703348572));
#268300=CARTESIAN_POINT('Ctrl Pts',(-126.9104585261,97.530998038622,681.537703348572));
#268301=CARTESIAN_POINT('Ctrl Pts',(-119.234602512152,107.519067738521,
679.537703348572));
#268302=CARTESIAN_POINT('Ctrl Pts',(-110.0907706828,116.183399296895,677.537703348572));
#268303=CARTESIAN_POINT('Ctrl Pts',(-100.946938853448,124.847730855269,
675.537703348572));
#268304=CARTESIAN_POINT('Ctrl Pts',(-90.5602826949695,131.974979673883,
673.537703348572));
#268305=CARTESIAN_POINT('Ctrl Pts',(-80.1736265364906,139.102228492497,
671.537703348572));
#268306=CARTESIAN_POINT('Ctrl Pts',(-68.7998999948417,144.516898051454,
669.537703348572));
#268307=CARTESIAN_POINT('Ctrl Pts',(-57.4261734531929,149.931567610411,
667.537703348572));
#268308=CARTESIAN_POINT('Ctrl Pts',(-45.3454354230638,153.500330774912,
665.537703348572));
#268309=CARTESIAN_POINT('Ctrl Pts',(-33.2646973929347,157.069093939413,
663.537703348572));
#268310=CARTESIAN_POINT('Ctrl Pts',(-20.774415738298,158.704075916301,661.537703348572));
#268311=CARTESIAN_POINT('Ctrl Pts',(-8.28413408366129,160.339057893189,
659.537703348572));
#268312=CARTESIAN_POINT('Ctrl Pts',(4.30813900827766,160.,657.537703348572));
#268313=CARTESIAN_POINT('Ctrl Pts',(16.9004121002166,159.660942106811,655.537703348572));
#268314=CARTESIAN_POINT('Ctrl Pts',(29.2846130745759,157.356193074143,653.537703348572));
#268315=CARTESIAN_POINT('Ctrl Pts',(41.6688140489352,155.051444041476,651.537703348572));
#268316=CARTESIAN_POINT('Ctrl Pts',(53.5400027769194,150.837754439537,649.537703348572));
#268317=CARTESIAN_POINT('Ctrl Pts',(65.4111915049037,146.624064837599,647.537703348572));
#268318=CARTESIAN_POINT('Ctrl Pts',(76.4770599218133,140.605189688823,645.537703348572));
#268319=CARTESIAN_POINT('Ctrl Pts',(87.542928338723,134.586314540048,643.537703348572));
#268320=CARTESIAN_POINT('Ctrl Pts',(97.530998038622,126.9104585261,641.537703348572));
#268321=CARTESIAN_POINT('Ctrl Pts',(107.519067738521,119.234602512152,639.537703348572));
#268322=CARTESIAN_POINT('Ctrl Pts',(116.183399296895,110.0907706828,637.537703348572));
#268323=CARTESIAN_POINT('Ctrl Pts',(124.847730855269,100.946938853448,635.537703348572));
#268324=CARTESIAN_POINT('Ctrl Pts',(131.974979673883,90.5602826949695,633.537703348572));
#268325=CARTESIAN_POINT('Ctrl Pts',(139.102228492497,80.1736265364906,631.537703348572));
#268326=CARTESIAN_POINT('Ctrl Pts',(144.516898051454,68.7998999948417,629.537703348572));
#268327=CARTESIAN_POINT('Ctrl Pts',(149.931567610411,57.4261734531929,627.537703348572));
#268328=CARTESIAN_POINT('Ctrl Pts',(153.500330774912,45.3454354230638,625.537703348572));
#268329=CARTESIAN_POINT('Ctrl Pts',(157.069093939413,33.2646973929347,623.537703348572));
#268330=CARTESIAN_POINT('Ctrl Pts',(158.704075916301,20.774415738298,621.537703348572));
#268331=CARTESIAN_POINT('Ctrl Pts',(160.339057893189,8.28413408366131,619.537703348572));
#268332=CARTESIAN_POINT('Ctrl Pts',(160.,-4.30813900827765,617.537703348572));
#268333=CARTESIAN_POINT('Ctrl Pts',(159.660942106811,-16.9004121002166,
615.537703348572));
#268334=CARTESIAN_POINT('Ctrl Pts',(157.356193074143,-29.2846130745759,
613.537703348572));
#268335=CARTESIAN_POINT('Ctrl Pts',(155.051444041476,-41.6688140489352,
611.537703348572));
#268336=CARTESIAN_POINT('Ctrl Pts',(150.837754439537,-53.5400027769194,
609.537703348572));
#268337=CARTESIAN_POINT('Ctrl Pts',(146.624064837599,-65.4111915049036,
607.537703348572));
#268338=CARTESIAN_POINT('Ctrl Pts',(140.605189688823,-76.4770599218133,
605.537703348572));
#268339=CARTESIAN_POINT('Ctrl Pts',(134.586314540048,-87.5429283387229,
603.537703348572));
#268340=CARTESIAN_POINT('Ctrl Pts',(126.9104585261,-97.530998038622,601.537703348572));
#268341=CARTESIAN_POINT('Ctrl Pts',(119.234602512152,-107.519067738521,
599.537703348572));
#268342=CARTESIAN_POINT('Ctrl Pts',(110.0907706828,-116.183399296895,597.537703348572));
#268343=CARTESIAN_POINT('Ctrl Pts',(100.946938853448,-124.847730855269,
595.537703348572));
#268344=CARTESIAN_POINT('Ctrl Pts',(90.5602826949695,-131.974979673883,
593.537703348572));
#268345=CARTESIAN_POINT('Ctrl Pts',(80.1736265364905,-139.102228492497,
591.537703348572));
#268346=CARTESIAN_POINT('Ctrl Pts',(68.7998999948417,-144.516898051454,
589.537703348572));
#268347=CARTESIAN_POINT('Ctrl Pts',(57.426173453193,-149.931567610411,587.537703348572));
#268348=CARTESIAN_POINT('Ctrl Pts',(45.3454354230638,-153.500330774912,
585.537703348572));
#268349=CARTESIAN_POINT('Ctrl Pts',(33.2646973929347,-157.069093939413,
583.537703348572));
#268350=CARTESIAN_POINT('Ctrl Pts',(20.774415738298,-158.704075916301,581.537703348572));
#268351=CARTESIAN_POINT('Ctrl Pts',(8.28413408366139,-160.339057893189,
579.537703348572));
#268352=CARTESIAN_POINT('Ctrl Pts',(-4.30813900827764,-160.,577.537703348572));
#268353=CARTESIAN_POINT('Ctrl Pts',(-16.9004121002167,-159.660942106811,
575.537703348572));
#268354=CARTESIAN_POINT('Ctrl Pts',(-29.2846130745759,-157.356193074143,
573.537703348572));
#268355=CARTESIAN_POINT('Ctrl Pts',(-41.6688140489351,-155.051444041476,
571.537703348572));
#268356=CARTESIAN_POINT('Ctrl Pts',(-53.5400027769194,-150.837754439537,
569.537703348572));
#268357=CARTESIAN_POINT('Ctrl Pts',(-65.4111915049037,-146.624064837599,
567.537703348572));
#268358=CARTESIAN_POINT('Ctrl Pts',(-76.4770599218133,-140.605189688823,
565.537703348572));
#268359=CARTESIAN_POINT('Ctrl Pts',(-87.5429283387229,-134.586314540048,
563.537703348572));
#268360=CARTESIAN_POINT('Ctrl Pts',(-97.530998038622,-126.9104585261,561.537703348572));
#268361=CARTESIAN_POINT('Ctrl Pts',(-107.519067738521,-119.234602512152,
559.537703348572));
#268362=CARTESIAN_POINT('Ctrl Pts',(-116.183399296895,-110.0907706828,557.537703348572));
#268363=CARTESIAN_POINT('Ctrl Pts',(-124.847730855269,-100.946938853448,
555.537703348572));
#268364=CARTESIAN_POINT('Ctrl Pts',(-131.974979673883,-90.5602826949695,
553.537703348572));
#268365=CARTESIAN_POINT('Ctrl Pts',(-139.102228492497,-80.1736265364905,
551.537703348572));
#268366=CARTESIAN_POINT('Ctrl Pts',(-144.516898051454,-68.7998999948417,
549.537703348572));
#268367=CARTESIAN_POINT('Ctrl Pts',(-149.931567610411,-57.426173453193,
547.537703348572));
#268368=CARTESIAN_POINT('Ctrl Pts',(-153.500330774912,-45.3454354230638,
545.537703348572));
#268369=CARTESIAN_POINT('Ctrl Pts',(-157.069093939413,-33.2646973929347,
543.537703348572));
#268370=CARTESIAN_POINT('Ctrl Pts',(-158.704075916301,-20.774415738298,
541.537703348572));
#268371=CARTESIAN_POINT('Ctrl Pts',(-160.339057893189,-8.2841340836614,
539.537703348572));
#268372=CARTESIAN_POINT('Ctrl Pts',(-160.,4.30813900827767,537.537703348572));
#268373=CARTESIAN_POINT('Ctrl Pts',(-130.,4.30813900827773,697.537703348572));
#268374=CARTESIAN_POINT('Ctrl Pts',(-129.660942106811,14.5393608954781,
695.537703348572));
#268375=CARTESIAN_POINT('Ctrl Pts',(-127.725542856289,24.591579123369,693.537703348572));
#268376=CARTESIAN_POINT('Ctrl Pts',(-125.790143605767,34.6437973512599,
691.537703348572));
#268377=CARTESIAN_POINT('Ctrl Pts',(-122.306058950683,44.269492945671,689.537703348572));
#268378=CARTESIAN_POINT('Ctrl Pts',(-118.821974295598,53.8951885400822,
687.537703348572));
#268379=CARTESIAN_POINT('Ctrl Pts',(-113.874993963172,62.8573449296269,
685.537703348572));
#268380=CARTESIAN_POINT('Ctrl Pts',(-108.928013630747,71.8195013191717,
683.537703348572));
#268381=CARTESIAN_POINT('Ctrl Pts',(-102.639948694852,79.8974404698478,
681.537703348572));
#268382=CARTESIAN_POINT('Ctrl Pts',(-96.3518837589562,87.9753796205239,
679.537703348572));
#268383=CARTESIAN_POINT('Ctrl Pts',(-88.8775672472037,94.9701958612987,
677.537703348572));
#268384=CARTESIAN_POINT('Ctrl Pts',(-81.4032507354512,101.965012102073,
675.537703348572));
#268385=CARTESIAN_POINT('Ctrl Pts',(-72.9267251261952,107.704469842635,
673.537703348572));
#268386=CARTESIAN_POINT('Ctrl Pts',(-64.4501995169392,113.443927583196,
671.537703348572));
#268387=CARTESIAN_POINT('Ctrl Pts',(-55.1801850026552,117.786702325803,
669.537703348572));
#268388=CARTESIAN_POINT('Ctrl Pts',(-45.9101704883713,122.12947706841,667.537703348572));
#268389=CARTESIAN_POINT('Ctrl Pts',(-36.0749255918153,124.968635286057,
665.537703348572));
#268390=CARTESIAN_POINT('Ctrl Pts',(-26.2396806952593,127.807793503704,
663.537703348572));
#268391=CARTESIAN_POINT('Ctrl Pts',(-16.081381787091,129.073425698447,661.537703348572));
#268392=CARTESIAN_POINT('Ctrl Pts',(-5.92308287892268,130.339057893189,
659.537703348572));
#268393=CARTESIAN_POINT('Ctrl Pts',(4.30813900827772,130.,657.537703348572));
#268394=CARTESIAN_POINT('Ctrl Pts',(14.5393608954781,129.660942106811,655.537703348572));
#268395=CARTESIAN_POINT('Ctrl Pts',(24.591579123369,127.725542856289,653.537703348572));
#268396=CARTESIAN_POINT('Ctrl Pts',(34.6437973512599,125.790143605767,651.537703348572));
#268397=CARTESIAN_POINT('Ctrl Pts',(44.269492945671,122.306058950683,649.537703348572));
#268398=CARTESIAN_POINT('Ctrl Pts',(53.8951885400822,118.821974295598,647.537703348572));
#268399=CARTESIAN_POINT('Ctrl Pts',(62.8573449296269,113.874993963172,645.537703348572));
#268400=CARTESIAN_POINT('Ctrl Pts',(71.8195013191717,108.928013630747,643.537703348572));
#268401=CARTESIAN_POINT('Ctrl Pts',(79.8974404698478,102.639948694852,641.537703348572));
#268402=CARTESIAN_POINT('Ctrl Pts',(87.9753796205239,96.3518837589562,639.537703348572));
#268403=CARTESIAN_POINT('Ctrl Pts',(94.9701958612986,88.8775672472037,637.537703348572));
#268404=CARTESIAN_POINT('Ctrl Pts',(101.965012102073,81.4032507354512,635.537703348572));
#268405=CARTESIAN_POINT('Ctrl Pts',(107.704469842635,72.9267251261952,633.537703348572));
#268406=CARTESIAN_POINT('Ctrl Pts',(113.443927583196,64.4501995169392,631.537703348572));
#268407=CARTESIAN_POINT('Ctrl Pts',(117.786702325803,55.1801850026552,629.537703348572));
#268408=CARTESIAN_POINT('Ctrl Pts',(122.12947706841,45.9101704883713,627.537703348572));
#268409=CARTESIAN_POINT('Ctrl Pts',(124.968635286057,36.0749255918153,625.537703348572));
#268410=CARTESIAN_POINT('Ctrl Pts',(127.807793503704,26.2396806952593,623.537703348572));
#268411=CARTESIAN_POINT('Ctrl Pts',(129.073425698447,16.081381787091,621.537703348572));
#268412=CARTESIAN_POINT('Ctrl Pts',(130.339057893189,5.92308287892268,619.537703348572));
#268413=CARTESIAN_POINT('Ctrl Pts',(130.,-4.30813900827772,617.537703348572));
#268414=CARTESIAN_POINT('Ctrl Pts',(129.660942106811,-14.5393608954781,
615.537703348572));
#268415=CARTESIAN_POINT('Ctrl Pts',(127.725542856289,-24.591579123369,613.537703348572));
#268416=CARTESIAN_POINT('Ctrl Pts',(125.790143605767,-34.6437973512599,
611.537703348572));
#268417=CARTESIAN_POINT('Ctrl Pts',(122.306058950683,-44.269492945671,609.537703348572));
#268418=CARTESIAN_POINT('Ctrl Pts',(118.821974295598,-53.8951885400822,
607.537703348572));
#268419=CARTESIAN_POINT('Ctrl Pts',(113.874993963172,-62.8573449296269,
605.537703348572));
#268420=CARTESIAN_POINT('Ctrl Pts',(108.928013630747,-71.8195013191717,
603.537703348572));
#268421=CARTESIAN_POINT('Ctrl Pts',(102.639948694852,-79.8974404698478,
601.537703348572));
#268422=CARTESIAN_POINT('Ctrl Pts',(96.3518837589563,-87.9753796205239,
599.537703348572));
#268423=CARTESIAN_POINT('Ctrl Pts',(88.8775672472037,-94.9701958612986,
597.537703348572));
#268424=CARTESIAN_POINT('Ctrl Pts',(81.4032507354513,-101.965012102073,
595.537703348572));
#268425=CARTESIAN_POINT('Ctrl Pts',(72.9267251261952,-107.704469842635,
593.537703348572));
#268426=CARTESIAN_POINT('Ctrl Pts',(64.4501995169392,-113.443927583196,
591.537703348572));
#268427=CARTESIAN_POINT('Ctrl Pts',(55.1801850026552,-117.786702325803,
589.537703348572));
#268428=CARTESIAN_POINT('Ctrl Pts',(45.9101704883713,-122.12947706841,587.537703348572));
#268429=CARTESIAN_POINT('Ctrl Pts',(36.0749255918153,-124.968635286057,
585.537703348572));
#268430=CARTESIAN_POINT('Ctrl Pts',(26.2396806952593,-127.807793503704,
583.537703348572));
#268431=CARTESIAN_POINT('Ctrl Pts',(16.081381787091,-129.073425698447,581.537703348572));
#268432=CARTESIAN_POINT('Ctrl Pts',(5.92308287892275,-130.339057893189,
579.537703348572));
#268433=CARTESIAN_POINT('Ctrl Pts',(-4.30813900827771,-130.,577.537703348572));
#268434=CARTESIAN_POINT('Ctrl Pts',(-14.5393608954782,-129.660942106811,
575.537703348572));
#268435=CARTESIAN_POINT('Ctrl Pts',(-24.591579123369,-127.725542856289,
573.537703348572));
#268436=CARTESIAN_POINT('Ctrl Pts',(-34.6437973512598,-125.790143605767,
571.537703348572));
#268437=CARTESIAN_POINT('Ctrl Pts',(-44.269492945671,-122.306058950683,
569.537703348572));
#268438=CARTESIAN_POINT('Ctrl Pts',(-53.8951885400822,-118.821974295598,
567.537703348572));
#268439=CARTESIAN_POINT('Ctrl Pts',(-62.8573449296269,-113.874993963172,
565.537703348572));
#268440=CARTESIAN_POINT('Ctrl Pts',(-71.8195013191717,-108.928013630747,
563.537703348572));
#268441=CARTESIAN_POINT('Ctrl Pts',(-79.8974404698478,-102.639948694852,
561.537703348572));
#268442=CARTESIAN_POINT('Ctrl Pts',(-87.975379620524,-96.3518837589562,
559.537703348572));
#268443=CARTESIAN_POINT('Ctrl Pts',(-94.9701958612986,-88.8775672472037,
557.537703348572));
#268444=CARTESIAN_POINT('Ctrl Pts',(-101.965012102073,-81.4032507354513,
555.537703348572));
#268445=CARTESIAN_POINT('Ctrl Pts',(-107.704469842635,-72.9267251261952,
553.537703348572));
#268446=CARTESIAN_POINT('Ctrl Pts',(-113.443927583196,-64.4501995169392,
551.537703348572));
#268447=CARTESIAN_POINT('Ctrl Pts',(-117.786702325803,-55.1801850026553,
549.537703348572));
#268448=CARTESIAN_POINT('Ctrl Pts',(-122.12947706841,-45.9101704883713,
547.537703348572));
#268449=CARTESIAN_POINT('Ctrl Pts',(-124.968635286057,-36.0749255918153,
545.537703348572));
#268450=CARTESIAN_POINT('Ctrl Pts',(-127.807793503704,-26.2396806952593,
543.537703348572));
#268451=CARTESIAN_POINT('Ctrl Pts',(-129.073425698447,-16.081381787091,
541.537703348572));
#268452=CARTESIAN_POINT('Ctrl Pts',(-130.339057893189,-5.92308287892275,
539.537703348572));
#268453=CARTESIAN_POINT('Ctrl Pts',(-130.,4.30813900827773,537.537703348572));
#268454=CARTESIAN_POINT('Ctrl Pts',(-130.,-4.30813900827845,532.462296651428));
#268455=CARTESIAN_POINT('Ctrl Pts',(-130.339057893189,5.92308287892195,
530.462296651429));
#268456=CARTESIAN_POINT('Ctrl Pts',(-129.073425698447,16.0813817870903,
528.462296651428));
#268457=CARTESIAN_POINT('Ctrl Pts',(-127.807793503705,26.2396806952586,
526.462296651429));
#268458=CARTESIAN_POINT('Ctrl Pts',(-124.968635286058,36.0749255918146,
524.462296651428));
#268459=CARTESIAN_POINT('Ctrl Pts',(-122.129477068411,45.9101704883706,
522.462296651428));
#268460=CARTESIAN_POINT('Ctrl Pts',(-117.786702325804,55.1801850026546,
520.462296651428));
#268461=CARTESIAN_POINT('Ctrl Pts',(-113.443927583196,64.4501995169386,
518.462296651428));
#268462=CARTESIAN_POINT('Ctrl Pts',(-107.704469842635,72.9267251261946,
516.462296651428));
#268463=CARTESIAN_POINT('Ctrl Pts',(-101.965012102074,81.4032507354507,
514.462296651428));
#268464=CARTESIAN_POINT('Ctrl Pts',(-94.9701958612992,88.8775672472032,
512.462296651428));
#268465=CARTESIAN_POINT('Ctrl Pts',(-87.9753796205245,96.3518837589558,
510.462296651429));
#268466=CARTESIAN_POINT('Ctrl Pts',(-79.8974404698484,102.639948694851,
508.462296651428));
#268467=CARTESIAN_POINT('Ctrl Pts',(-71.8195013191724,108.928013630747,
506.462296651428));
#268468=CARTESIAN_POINT('Ctrl Pts',(-62.8573449296276,113.874993963172,
504.462296651428));
#268469=CARTESIAN_POINT('Ctrl Pts',(-53.8951885400828,118.821974295598,
502.462296651428));
#268470=CARTESIAN_POINT('Ctrl Pts',(-44.2694929456717,122.306058950682,
500.462296651428));
#268471=CARTESIAN_POINT('Ctrl Pts',(-34.6437973512606,125.790143605767,
498.462296651429));
#268472=CARTESIAN_POINT('Ctrl Pts',(-24.5915791233697,127.725542856289,
496.462296651428));
#268473=CARTESIAN_POINT('Ctrl Pts',(-14.5393608954789,129.660942106811,
494.462296651428));
#268474=CARTESIAN_POINT('Ctrl Pts',(-4.30813900827846,130.,492.462296651428));
#268475=CARTESIAN_POINT('Ctrl Pts',(5.92308287892194,130.339057893189,490.462296651429));
#268476=CARTESIAN_POINT('Ctrl Pts',(16.0813817870903,129.073425698447,488.462296651428));
#268477=CARTESIAN_POINT('Ctrl Pts',(26.2396806952586,127.807793503705,486.462296651428));
#268478=CARTESIAN_POINT('Ctrl Pts',(36.0749255918146,124.968635286058,484.462296651428));
#268479=CARTESIAN_POINT('Ctrl Pts',(45.9101704883706,122.129477068411,482.462296651428));
#268480=CARTESIAN_POINT('Ctrl Pts',(55.1801850026546,117.786702325804,480.462296651428));
#268481=CARTESIAN_POINT('Ctrl Pts',(64.4501995169386,113.443927583196,478.462296651429));
#268482=CARTESIAN_POINT('Ctrl Pts',(72.9267251261946,107.704469842635,476.462296651428));
#268483=CARTESIAN_POINT('Ctrl Pts',(81.4032507354506,101.965012102074,474.462296651428));
#268484=CARTESIAN_POINT('Ctrl Pts',(88.8775672472032,94.9701958612992,472.462296651428));
#268485=CARTESIAN_POINT('Ctrl Pts',(96.3518837589558,87.9753796205245,470.462296651428));
#268486=CARTESIAN_POINT('Ctrl Pts',(102.639948694851,79.8974404698484,468.462296651428));
#268487=CARTESIAN_POINT('Ctrl Pts',(108.928013630747,71.8195013191724,466.462296651428));
#268488=CARTESIAN_POINT('Ctrl Pts',(113.874993963172,62.8573449296276,464.462296651428));
#268489=CARTESIAN_POINT('Ctrl Pts',(118.821974295598,53.8951885400829,462.462296651428));
#268490=CARTESIAN_POINT('Ctrl Pts',(122.306058950682,44.2694929456717,460.462296651428));
#268491=CARTESIAN_POINT('Ctrl Pts',(125.790143605767,34.6437973512606,458.462296651429));
#268492=CARTESIAN_POINT('Ctrl Pts',(127.725542856289,24.5915791233698,456.462296651428));
#268493=CARTESIAN_POINT('Ctrl Pts',(129.660942106811,14.5393608954789,454.462296651429));
#268494=CARTESIAN_POINT('Ctrl Pts',(130.,4.30813900827846,452.462296651428));
#268495=CARTESIAN_POINT('Ctrl Pts',(130.339057893189,-5.92308287892194,
450.462296651428));
#268496=CARTESIAN_POINT('Ctrl Pts',(129.073425698447,-16.0813817870903,
448.462296651429));
#268497=CARTESIAN_POINT('Ctrl Pts',(127.807793503705,-26.2396806952586,
446.462296651429));
#268498=CARTESIAN_POINT('Ctrl Pts',(124.968635286058,-36.0749255918146,
444.462296651429));
#268499=CARTESIAN_POINT('Ctrl Pts',(122.129477068411,-45.9101704883706,
442.462296651429));
#268500=CARTESIAN_POINT('Ctrl Pts',(117.786702325804,-55.1801850026546,
440.462296651428));
#268501=CARTESIAN_POINT('Ctrl Pts',(113.443927583196,-64.4501995169386,
438.462296651429));
#268502=CARTESIAN_POINT('Ctrl Pts',(107.704469842635,-72.9267251261946,
436.462296651428));
#268503=CARTESIAN_POINT('Ctrl Pts',(101.965012102074,-81.4032507354506,
434.462296651429));
#268504=CARTESIAN_POINT('Ctrl Pts',(94.9701958612992,-88.8775672472032,
432.462296651428));
#268505=CARTESIAN_POINT('Ctrl Pts',(87.9753796205246,-96.3518837589557,
430.462296651429));
#268506=CARTESIAN_POINT('Ctrl Pts',(79.8974404698484,-102.639948694851,
428.462296651429));
#268507=CARTESIAN_POINT('Ctrl Pts',(71.8195013191723,-108.928013630747,
426.462296651428));
#268508=CARTESIAN_POINT('Ctrl Pts',(62.8573449296276,-113.874993963172,
424.462296651428));
#268509=CARTESIAN_POINT('Ctrl Pts',(53.8951885400829,-118.821974295598,
422.462296651428));
#268510=CARTESIAN_POINT('Ctrl Pts',(44.2694929456717,-122.306058950682,
420.462296651428));
#268511=CARTESIAN_POINT('Ctrl Pts',(34.6437973512606,-125.790143605767,
418.462296651429));
#268512=CARTESIAN_POINT('Ctrl Pts',(24.5915791233698,-127.725542856289,
416.462296651428));
#268513=CARTESIAN_POINT('Ctrl Pts',(14.5393608954789,-129.660942106811,
414.462296651429));
#268514=CARTESIAN_POINT('Ctrl Pts',(4.30813900827847,-130.,412.462296651428));
#268515=CARTESIAN_POINT('Ctrl Pts',(-5.92308287892199,-130.339057893189,
410.462296651428));
#268516=CARTESIAN_POINT('Ctrl Pts',(-16.0813817870903,-129.073425698447,
408.462296651428));
#268517=CARTESIAN_POINT('Ctrl Pts',(-26.2396806952585,-127.807793503705,
406.462296651429));
#268518=CARTESIAN_POINT('Ctrl Pts',(-36.0749255918146,-124.968635286058,
404.462296651428));
#268519=CARTESIAN_POINT('Ctrl Pts',(-45.9101704883706,-122.129477068411,
402.462296651429));
#268520=CARTESIAN_POINT('Ctrl Pts',(-55.1801850026546,-117.786702325804,
400.462296651428));
#268521=CARTESIAN_POINT('Ctrl Pts',(-64.4501995169385,-113.443927583197,
398.462296651429));
#268522=CARTESIAN_POINT('Ctrl Pts',(-72.9267251261946,-107.704469842635,
396.462296651428));
#268523=CARTESIAN_POINT('Ctrl Pts',(-81.4032507354507,-101.965012102074,
394.462296651429));
#268524=CARTESIAN_POINT('Ctrl Pts',(-88.8775672472032,-94.9701958612992,
392.462296651428));
#268525=CARTESIAN_POINT('Ctrl Pts',(-96.3518837589557,-87.9753796205246,
390.462296651428));
#268526=CARTESIAN_POINT('Ctrl Pts',(-102.639948694851,-79.8974404698484,
388.462296651428));
#268527=CARTESIAN_POINT('Ctrl Pts',(-108.928013630747,-71.8195013191723,
386.462296651428));
#268528=CARTESIAN_POINT('Ctrl Pts',(-113.874993963172,-62.8573449296276,
384.462296651428));
#268529=CARTESIAN_POINT('Ctrl Pts',(-118.821974295598,-53.8951885400829,
382.462296651429));
#268530=CARTESIAN_POINT('Ctrl Pts',(-122.306058950682,-44.2694929456718,
380.462296651428));
#268531=CARTESIAN_POINT('Ctrl Pts',(-125.790143605767,-34.6437973512606,
378.462296651429));
#268532=CARTESIAN_POINT('Ctrl Pts',(-127.725542856289,-24.5915791233698,
376.462296651428));
#268533=CARTESIAN_POINT('Ctrl Pts',(-129.660942106811,-14.5393608954789,
374.462296651428));
#268534=CARTESIAN_POINT('Ctrl Pts',(-130.,-4.30813900827845,372.462296651428));
#268535=CARTESIAN_POINT('Ctrl Pts',(-160.,-4.30813900827851,532.462296651429));
#268536=CARTESIAN_POINT('Ctrl Pts',(-160.339057893189,8.28413408366045,
530.462296651429));
#268537=CARTESIAN_POINT('Ctrl Pts',(-158.704075916301,20.7744157382972,
528.462296651429));
#268538=CARTESIAN_POINT('Ctrl Pts',(-157.069093939413,33.2646973929339,
526.462296651429));
#268539=CARTESIAN_POINT('Ctrl Pts',(-153.500330774912,45.345435423063,524.462296651428));
#268540=CARTESIAN_POINT('Ctrl Pts',(-149.931567610412,57.4261734531921,
522.462296651429));
#268541=CARTESIAN_POINT('Ctrl Pts',(-144.516898051455,68.7998999948409,
520.462296651428));
#268542=CARTESIAN_POINT('Ctrl Pts',(-139.102228492498,80.1736265364898,
518.462296651428));
#268543=CARTESIAN_POINT('Ctrl Pts',(-131.974979673884,90.5602826949688,
516.462296651428));
#268544=CARTESIAN_POINT('Ctrl Pts',(-124.84773085527,100.946938853448,514.462296651429));
#268545=CARTESIAN_POINT('Ctrl Pts',(-116.183399296896,110.0907706828,512.462296651428));
#268546=CARTESIAN_POINT('Ctrl Pts',(-107.519067738522,119.234602512151,
510.462296651429));
#268547=CARTESIAN_POINT('Ctrl Pts',(-97.5309980386227,126.9104585261,508.462296651429));
#268548=CARTESIAN_POINT('Ctrl Pts',(-87.5429283387237,134.586314540048,
506.462296651428));
#268549=CARTESIAN_POINT('Ctrl Pts',(-76.4770599218141,140.605189688823,
504.462296651429));
#268550=CARTESIAN_POINT('Ctrl Pts',(-65.4111915049045,146.624064837598,
502.462296651429));
#268551=CARTESIAN_POINT('Ctrl Pts',(-53.5400027769202,150.837754439537,
500.462296651429));
#268552=CARTESIAN_POINT('Ctrl Pts',(-41.668814048936,155.051444041475,498.462296651429));
#268553=CARTESIAN_POINT('Ctrl Pts',(-29.2846130745767,157.356193074143,
496.462296651429));
#268554=CARTESIAN_POINT('Ctrl Pts',(-16.9004121002175,159.660942106811,
494.462296651429));
#268555=CARTESIAN_POINT('Ctrl Pts',(-4.30813900827852,160.,492.462296651428));
#268556=CARTESIAN_POINT('Ctrl Pts',(8.28413408366043,160.339057893189,490.462296651429));
#268557=CARTESIAN_POINT('Ctrl Pts',(20.7744157382972,158.704075916301,488.462296651429));
#268558=CARTESIAN_POINT('Ctrl Pts',(33.2646973929339,157.069093939413,486.462296651429));
#268559=CARTESIAN_POINT('Ctrl Pts',(45.345435423063,153.500330774912,484.462296651429));
#268560=CARTESIAN_POINT('Ctrl Pts',(57.4261734531921,149.931567610412,482.462296651429));
#268561=CARTESIAN_POINT('Ctrl Pts',(68.7998999948409,144.516898051455,480.462296651428));
#268562=CARTESIAN_POINT('Ctrl Pts',(80.1736265364898,139.102228492498,478.462296651429));
#268563=CARTESIAN_POINT('Ctrl Pts',(90.5602826949688,131.974979673884,476.462296651428));
#268564=CARTESIAN_POINT('Ctrl Pts',(100.946938853448,124.84773085527,474.462296651429));
#268565=CARTESIAN_POINT('Ctrl Pts',(110.0907706828,116.183399296896,472.462296651429));
#268566=CARTESIAN_POINT('Ctrl Pts',(119.234602512151,107.519067738522,470.462296651429));
#268567=CARTESIAN_POINT('Ctrl Pts',(126.9104585261,97.5309980386227,468.462296651429));
#268568=CARTESIAN_POINT('Ctrl Pts',(134.586314540048,87.5429283387237,466.462296651429));
#268569=CARTESIAN_POINT('Ctrl Pts',(140.605189688823,76.4770599218141,464.462296651429));
#268570=CARTESIAN_POINT('Ctrl Pts',(146.624064837598,65.4111915049045,462.462296651429));
#268571=CARTESIAN_POINT('Ctrl Pts',(150.837754439537,53.5400027769202,460.462296651429));
#268572=CARTESIAN_POINT('Ctrl Pts',(155.051444041475,41.668814048936,458.462296651429));
#268573=CARTESIAN_POINT('Ctrl Pts',(157.356193074143,29.2846130745767,456.462296651429));
#268574=CARTESIAN_POINT('Ctrl Pts',(159.660942106811,16.9004121002175,454.462296651429));
#268575=CARTESIAN_POINT('Ctrl Pts',(160.,4.30813900827853,452.462296651429));
#268576=CARTESIAN_POINT('Ctrl Pts',(160.339057893189,-8.28413408366043,
450.462296651429));
#268577=CARTESIAN_POINT('Ctrl Pts',(158.704075916301,-20.7744157382971,
448.462296651429));
#268578=CARTESIAN_POINT('Ctrl Pts',(157.069093939413,-33.2646973929339,
446.462296651429));
#268579=CARTESIAN_POINT('Ctrl Pts',(153.500330774912,-45.345435423063,444.462296651429));
#268580=CARTESIAN_POINT('Ctrl Pts',(149.931567610412,-57.4261734531921,
442.462296651429));
#268581=CARTESIAN_POINT('Ctrl Pts',(144.516898051455,-68.7998999948409,
440.462296651429));
#268582=CARTESIAN_POINT('Ctrl Pts',(139.102228492498,-80.1736265364898,
438.462296651429));
#268583=CARTESIAN_POINT('Ctrl Pts',(131.974979673884,-90.5602826949688,
436.462296651429));
#268584=CARTESIAN_POINT('Ctrl Pts',(124.84773085527,-100.946938853448,434.462296651429));
#268585=CARTESIAN_POINT('Ctrl Pts',(116.183399296896,-110.0907706828,432.462296651429));
#268586=CARTESIAN_POINT('Ctrl Pts',(107.519067738522,-119.234602512151,
430.462296651429));
#268587=CARTESIAN_POINT('Ctrl Pts',(97.5309980386227,-126.9104585261,428.462296651429));
#268588=CARTESIAN_POINT('Ctrl Pts',(87.5429283387236,-134.586314540048,
426.462296651429));
#268589=CARTESIAN_POINT('Ctrl Pts',(76.4770599218141,-140.605189688823,
424.462296651429));
#268590=CARTESIAN_POINT('Ctrl Pts',(65.4111915049046,-146.624064837598,
422.462296651429));
#268591=CARTESIAN_POINT('Ctrl Pts',(53.5400027769202,-150.837754439537,
420.462296651429));
#268592=CARTESIAN_POINT('Ctrl Pts',(41.6688140489359,-155.051444041475,
418.462296651429));
#268593=CARTESIAN_POINT('Ctrl Pts',(29.2846130745768,-157.356193074143,
416.462296651429));
#268594=CARTESIAN_POINT('Ctrl Pts',(16.9004121002176,-159.660942106811,
414.462296651429));
#268595=CARTESIAN_POINT('Ctrl Pts',(4.30813900827854,-160.,412.462296651429));
#268596=CARTESIAN_POINT('Ctrl Pts',(-8.28413408366049,-160.339057893189,
410.462296651429));
#268597=CARTESIAN_POINT('Ctrl Pts',(-20.7744157382971,-158.704075916301,
408.462296651429));
#268598=CARTESIAN_POINT('Ctrl Pts',(-33.2646973929338,-157.069093939413,
406.462296651429));
#268599=CARTESIAN_POINT('Ctrl Pts',(-45.345435423063,-153.500330774912,
404.462296651429));
#268600=CARTESIAN_POINT('Ctrl Pts',(-57.4261734531921,-149.931567610412,
402.462296651429));
#268601=CARTESIAN_POINT('Ctrl Pts',(-68.7998999948409,-144.516898051455,
400.462296651429));
#268602=CARTESIAN_POINT('Ctrl Pts',(-80.1736265364897,-139.102228492498,
398.462296651429));
#268603=CARTESIAN_POINT('Ctrl Pts',(-90.5602826949688,-131.974979673884,
396.462296651429));
#268604=CARTESIAN_POINT('Ctrl Pts',(-100.946938853448,-124.84773085527,
394.462296651429));
#268605=CARTESIAN_POINT('Ctrl Pts',(-110.0907706828,-116.183399296896,392.462296651429));
#268606=CARTESIAN_POINT('Ctrl Pts',(-119.234602512151,-107.519067738522,
390.462296651429));
#268607=CARTESIAN_POINT('Ctrl Pts',(-126.9104585261,-97.5309980386227,388.462296651429));
#268608=CARTESIAN_POINT('Ctrl Pts',(-134.586314540048,-87.5429283387236,
386.462296651429));
#268609=CARTESIAN_POINT('Ctrl Pts',(-140.605189688823,-76.4770599218141,
384.462296651429));
#268610=CARTESIAN_POINT('Ctrl Pts',(-146.624064837598,-65.4111915049046,
382.462296651429));
#268611=CARTESIAN_POINT('Ctrl Pts',(-150.837754439537,-53.5400027769203,
380.462296651429));
#268612=CARTESIAN_POINT('Ctrl Pts',(-155.051444041475,-41.668814048936,
378.462296651429));
#268613=CARTESIAN_POINT('Ctrl Pts',(-157.356193074143,-29.2846130745768,
376.462296651429));
#268614=CARTESIAN_POINT('Ctrl Pts',(-159.660942106811,-16.9004121002176,
374.462296651429));
#268615=CARTESIAN_POINT('Ctrl Pts',(-160.,-4.30813900827851,372.462296651429));
#268616=CARTESIAN_POINT('Origin',(4.03737035483175,-0.209103843988196,530.46237739249));
#268617=CARTESIAN_POINT('Ctrl Pts',(-160.,-4.30813900827851,532.462296651429));
#268618=CARTESIAN_POINT('Ctrl Pts',(-160.339057893189,8.28413408366045,
530.462296651429));
#268619=CARTESIAN_POINT('Ctrl Pts',(-158.704075916301,20.7744157382972,
528.462296651429));
#268620=CARTESIAN_POINT('Ctrl Pts',(-157.069093939413,33.2646973929339,
526.462296651429));
#268621=CARTESIAN_POINT('Ctrl Pts',(-153.500330774912,45.345435423063,524.462296651428));
#268622=CARTESIAN_POINT('Ctrl Pts',(-149.931567610412,57.4261734531921,
522.462296651429));
#268623=CARTESIAN_POINT('Ctrl Pts',(-144.516898051455,68.7998999948409,
520.462296651428));
#268624=CARTESIAN_POINT('Ctrl Pts',(-139.102228492498,80.1736265364898,
518.462296651428));
#268625=CARTESIAN_POINT('Ctrl Pts',(-131.974979673884,90.5602826949688,
516.462296651428));
#268626=CARTESIAN_POINT('Ctrl Pts',(-124.84773085527,100.946938853448,514.462296651429));
#268627=CARTESIAN_POINT('Ctrl Pts',(-116.183399296896,110.0907706828,512.462296651428));
#268628=CARTESIAN_POINT('Ctrl Pts',(-107.519067738522,119.234602512151,
510.462296651429));
#268629=CARTESIAN_POINT('Ctrl Pts',(-97.5309980386227,126.9104585261,508.462296651429));
#268630=CARTESIAN_POINT('Ctrl Pts',(-87.5429283387237,134.586314540048,
506.462296651428));
#268631=CARTESIAN_POINT('Ctrl Pts',(-76.4770599218141,140.605189688823,
504.462296651429));
#268632=CARTESIAN_POINT('Ctrl Pts',(-65.4111915049045,146.624064837598,
502.462296651429));
#268633=CARTESIAN_POINT('Ctrl Pts',(-53.5400027769202,150.837754439537,
500.462296651429));
#268634=CARTESIAN_POINT('Ctrl Pts',(-41.668814048936,155.051444041475,498.462296651429));
#268635=CARTESIAN_POINT('Ctrl Pts',(-29.2846130745767,157.356193074143,
496.462296651429));
#268636=CARTESIAN_POINT('Ctrl Pts',(-16.9004121002175,159.660942106811,
494.462296651429));
#268637=CARTESIAN_POINT('Ctrl Pts',(-4.30813900827852,160.,492.462296651428));
#268638=CARTESIAN_POINT('Ctrl Pts',(8.28413408366043,160.339057893189,490.462296651429));
#268639=CARTESIAN_POINT('Ctrl Pts',(20.7744157382972,158.704075916301,488.462296651429));
#268640=CARTESIAN_POINT('Ctrl Pts',(33.2646973929339,157.069093939413,486.462296651429));
#268641=CARTESIAN_POINT('Ctrl Pts',(45.345435423063,153.500330774912,484.462296651429));
#268642=CARTESIAN_POINT('Ctrl Pts',(57.4261734531921,149.931567610412,482.462296651429));
#268643=CARTESIAN_POINT('Ctrl Pts',(68.7998999948409,144.516898051455,480.462296651428));
#268644=CARTESIAN_POINT('Ctrl Pts',(80.1736265364898,139.102228492498,478.462296651429));
#268645=CARTESIAN_POINT('Ctrl Pts',(90.5602826949688,131.974979673884,476.462296651428));
#268646=CARTESIAN_POINT('Ctrl Pts',(100.946938853448,124.84773085527,474.462296651429));
#268647=CARTESIAN_POINT('Ctrl Pts',(110.0907706828,116.183399296896,472.462296651429));
#268648=CARTESIAN_POINT('Ctrl Pts',(119.234602512151,107.519067738522,470.462296651429));
#268649=CARTESIAN_POINT('Ctrl Pts',(126.9104585261,97.5309980386227,468.462296651429));
#268650=CARTESIAN_POINT('Ctrl Pts',(134.586314540048,87.5429283387237,466.462296651429));
#268651=CARTESIAN_POINT('Ctrl Pts',(140.605189688823,76.4770599218141,464.462296651429));
#268652=CARTESIAN_POINT('Ctrl Pts',(146.624064837598,65.4111915049045,462.462296651429));
#268653=CARTESIAN_POINT('Ctrl Pts',(150.837754439537,53.5400027769202,460.462296651429));
#268654=CARTESIAN_POINT('Ctrl Pts',(155.051444041475,41.668814048936,458.462296651429));
#268655=CARTESIAN_POINT('Ctrl Pts',(157.356193074143,29.2846130745767,456.462296651429));
#268656=CARTESIAN_POINT('Ctrl Pts',(159.660942106811,16.9004121002175,454.462296651429));
#268657=CARTESIAN_POINT('Ctrl Pts',(160.,4.30813900827853,452.462296651429));
#268658=CARTESIAN_POINT('Ctrl Pts',(160.339057893189,-8.28413408366043,
450.462296651429));
#268659=CARTESIAN_POINT('Ctrl Pts',(158.704075916301,-20.7744157382971,
448.462296651429));
#268660=CARTESIAN_POINT('Ctrl Pts',(157.069093939413,-33.2646973929339,
446.462296651429));
#268661=CARTESIAN_POINT('Ctrl Pts',(153.500330774912,-45.345435423063,444.462296651429));
#268662=CARTESIAN_POINT('Ctrl Pts',(149.931567610412,-57.4261734531921,
442.462296651429));
#268663=CARTESIAN_POINT('Ctrl Pts',(144.516898051455,-68.7998999948409,
440.462296651429));
#268664=CARTESIAN_POINT('Ctrl Pts',(139.102228492498,-80.1736265364898,
438.462296651429));
#268665=CARTESIAN_POINT('Ctrl Pts',(131.974979673884,-90.5602826949688,
436.462296651429));
#268666=CARTESIAN_POINT('Ctrl Pts',(124.84773085527,-100.946938853448,434.462296651429));
#268667=CARTESIAN_POINT('Ctrl Pts',(116.183399296896,-110.0907706828,432.462296651429));
#268668=CARTESIAN_POINT('Ctrl Pts',(107.519067738522,-119.234602512151,
430.462296651429));
#268669=CARTESIAN_POINT('Ctrl Pts',(97.5309980386227,-126.9104585261,428.462296651429));
#268670=CARTESIAN_POINT('Ctrl Pts',(87.5429283387236,-134.586314540048,
426.462296651429));
#268671=CARTESIAN_POINT('Ctrl Pts',(76.4770599218141,-140.605189688823,
424.462296651429));
#268672=CARTESIAN_POINT('Ctrl Pts',(65.4111915049046,-146.624064837598,
422.462296651429));
#268673=CARTESIAN_POINT('Ctrl Pts',(53.5400027769202,-150.837754439537,
420.462296651429));
#268674=CARTESIAN_POINT('Ctrl Pts',(41.6688140489359,-155.051444041475,
418.462296651429));
#268675=CARTESIAN_POINT('Ctrl Pts',(29.2846130745768,-157.356193074143,
416.462296651429));
#268676=CARTESIAN_POINT('Ctrl Pts',(16.9004121002176,-159.660942106811,
414.462296651429));
#268677=CARTESIAN_POINT('Ctrl Pts',(4.30813900827854,-160.,412.462296651429));
#268678=CARTESIAN_POINT('Ctrl Pts',(-8.28413408366049,-160.339057893189,
410.462296651429));
#268679=CARTESIAN_POINT('Ctrl Pts',(-20.7744157382971,-158.704075916301,
408.462296651429));
#268680=CARTESIAN_POINT('Ctrl Pts',(-33.2646973929338,-157.069093939413,
406.462296651429));
#268681=CARTESIAN_POINT('Ctrl Pts',(-45.345435423063,-153.500330774912,
404.462296651429));
#268682=CARTESIAN_POINT('Ctrl Pts',(-57.4261734531921,-149.931567610412,
402.462296651429));
#268683=CARTESIAN_POINT('Ctrl Pts',(-68.7998999948409,-144.516898051455,
400.462296651429));
#268684=CARTESIAN_POINT('Ctrl Pts',(-80.1736265364897,-139.102228492498,
398.462296651429));
#268685=CARTESIAN_POINT('Ctrl Pts',(-90.5602826949688,-131.974979673884,
396.462296651429));
#268686=CARTESIAN_POINT('Ctrl Pts',(-100.946938853448,-124.84773085527,
394.462296651429));
#268687=CARTESIAN_POINT('Ctrl Pts',(-110.0907706828,-116.183399296896,392.462296651429));
#268688=CARTESIAN_POINT('Ctrl Pts',(-119.234602512151,-107.519067738522,
390.462296651429));
#268689=CARTESIAN_POINT('Ctrl Pts',(-126.9104585261,-97.5309980386227,388.462296651429));
#268690=CARTESIAN_POINT('Ctrl Pts',(-134.586314540048,-87.5429283387236,
386.462296651429));
#268691=CARTESIAN_POINT('Ctrl Pts',(-140.605189688823,-76.4770599218141,
384.462296651429));
#268692=CARTESIAN_POINT('Ctrl Pts',(-146.624064837598,-65.4111915049046,
382.462296651429));
#268693=CARTESIAN_POINT('Ctrl Pts',(-150.837754439537,-53.5400027769203,
380.462296651429));
#268694=CARTESIAN_POINT('Ctrl Pts',(-155.051444041475,-41.668814048936,
378.462296651429));
#268695=CARTESIAN_POINT('Ctrl Pts',(-157.356193074143,-29.2846130745768,
376.462296651429));
#268696=CARTESIAN_POINT('Ctrl Pts',(-159.660942106811,-16.9004121002176,
374.462296651429));
#268697=CARTESIAN_POINT('Ctrl Pts',(-160.,-4.30813900827851,372.462296651429));
#268698=CARTESIAN_POINT('Ctrl Pts',(-160.,4.30813900827767,537.537703348572));
#268699=CARTESIAN_POINT('Ctrl Pts',(-159.660942106811,16.9004121002166,
535.537703348572));
#268700=CARTESIAN_POINT('Ctrl Pts',(-157.356193074143,29.2846130745759,
533.537703348572));
#268701=CARTESIAN_POINT('Ctrl Pts',(-155.051444041476,41.6688140489352,
531.537703348572));
#268702=CARTESIAN_POINT('Ctrl Pts',(-150.837754439537,53.5400027769194,
529.537703348572));
#268703=CARTESIAN_POINT('Ctrl Pts',(-146.624064837599,65.4111915049037,
527.537703348572));
#268704=CARTESIAN_POINT('Ctrl Pts',(-140.605189688823,76.4770599218133,
525.537703348572));
#268705=CARTESIAN_POINT('Ctrl Pts',(-134.586314540048,87.542928338723,523.537703348572));
#268706=CARTESIAN_POINT('Ctrl Pts',(-126.9104585261,97.530998038622,521.537703348572));
#268707=CARTESIAN_POINT('Ctrl Pts',(-119.234602512152,107.519067738521,
519.537703348572));
#268708=CARTESIAN_POINT('Ctrl Pts',(-110.0907706828,116.183399296895,517.537703348572));
#268709=CARTESIAN_POINT('Ctrl Pts',(-100.946938853448,124.847730855269,
515.537703348572));
#268710=CARTESIAN_POINT('Ctrl Pts',(-90.5602826949695,131.974979673883,
513.537703348572));
#268711=CARTESIAN_POINT('Ctrl Pts',(-80.1736265364906,139.102228492497,
511.537703348572));
#268712=CARTESIAN_POINT('Ctrl Pts',(-68.7998999948417,144.516898051454,
509.537703348572));
#268713=CARTESIAN_POINT('Ctrl Pts',(-57.4261734531929,149.931567610411,
507.537703348572));
#268714=CARTESIAN_POINT('Ctrl Pts',(-45.3454354230638,153.500330774912,
505.537703348572));
#268715=CARTESIAN_POINT('Ctrl Pts',(-33.2646973929347,157.069093939413,
503.537703348572));
#268716=CARTESIAN_POINT('Ctrl Pts',(-20.774415738298,158.704075916301,501.537703348572));
#268717=CARTESIAN_POINT('Ctrl Pts',(-8.28413408366129,160.339057893189,
499.537703348572));
#268718=CARTESIAN_POINT('Ctrl Pts',(4.30813900827766,160.,497.537703348572));
#268719=CARTESIAN_POINT('Ctrl Pts',(16.9004121002166,159.660942106811,495.537703348572));
#268720=CARTESIAN_POINT('Ctrl Pts',(29.2846130745759,157.356193074143,493.537703348572));
#268721=CARTESIAN_POINT('Ctrl Pts',(41.6688140489352,155.051444041476,491.537703348572));
#268722=CARTESIAN_POINT('Ctrl Pts',(53.5400027769194,150.837754439537,489.537703348572));
#268723=CARTESIAN_POINT('Ctrl Pts',(65.4111915049037,146.624064837599,487.537703348572));
#268724=CARTESIAN_POINT('Ctrl Pts',(76.4770599218133,140.605189688823,485.537703348572));
#268725=CARTESIAN_POINT('Ctrl Pts',(87.542928338723,134.586314540048,483.537703348572));
#268726=CARTESIAN_POINT('Ctrl Pts',(97.530998038622,126.9104585261,481.537703348572));
#268727=CARTESIAN_POINT('Ctrl Pts',(107.519067738521,119.234602512152,479.537703348572));
#268728=CARTESIAN_POINT('Ctrl Pts',(116.183399296895,110.0907706828,477.537703348572));
#268729=CARTESIAN_POINT('Ctrl Pts',(124.847730855269,100.946938853448,475.537703348572));
#268730=CARTESIAN_POINT('Ctrl Pts',(131.974979673883,90.5602826949695,473.537703348572));
#268731=CARTESIAN_POINT('Ctrl Pts',(139.102228492497,80.1736265364906,471.537703348572));
#268732=CARTESIAN_POINT('Ctrl Pts',(144.516898051454,68.7998999948417,469.537703348572));
#268733=CARTESIAN_POINT('Ctrl Pts',(149.931567610411,57.4261734531929,467.537703348572));
#268734=CARTESIAN_POINT('Ctrl Pts',(153.500330774912,45.3454354230638,465.537703348572));
#268735=CARTESIAN_POINT('Ctrl Pts',(157.069093939413,33.2646973929347,463.537703348572));
#268736=CARTESIAN_POINT('Ctrl Pts',(158.704075916301,20.774415738298,461.537703348572));
#268737=CARTESIAN_POINT('Ctrl Pts',(160.339057893189,8.28413408366131,459.537703348572));
#268738=CARTESIAN_POINT('Ctrl Pts',(160.,-4.30813900827765,457.537703348572));
#268739=CARTESIAN_POINT('Ctrl Pts',(159.660942106811,-16.9004121002166,
455.537703348572));
#268740=CARTESIAN_POINT('Ctrl Pts',(157.356193074143,-29.2846130745759,
453.537703348572));
#268741=CARTESIAN_POINT('Ctrl Pts',(155.051444041476,-41.6688140489352,
451.537703348572));
#268742=CARTESIAN_POINT('Ctrl Pts',(150.837754439537,-53.5400027769194,
449.537703348572));
#268743=CARTESIAN_POINT('Ctrl Pts',(146.624064837599,-65.4111915049036,
447.537703348572));
#268744=CARTESIAN_POINT('Ctrl Pts',(140.605189688823,-76.4770599218133,
445.537703348572));
#268745=CARTESIAN_POINT('Ctrl Pts',(134.586314540048,-87.5429283387229,
443.537703348572));
#268746=CARTESIAN_POINT('Ctrl Pts',(126.9104585261,-97.530998038622,441.537703348572));
#268747=CARTESIAN_POINT('Ctrl Pts',(119.234602512152,-107.519067738521,
439.537703348572));
#268748=CARTESIAN_POINT('Ctrl Pts',(110.0907706828,-116.183399296895,437.537703348572));
#268749=CARTESIAN_POINT('Ctrl Pts',(100.946938853448,-124.847730855269,
435.537703348572));
#268750=CARTESIAN_POINT('Ctrl Pts',(90.5602826949695,-131.974979673883,
433.537703348572));
#268751=CARTESIAN_POINT('Ctrl Pts',(80.1736265364905,-139.102228492497,
431.537703348572));
#268752=CARTESIAN_POINT('Ctrl Pts',(68.7998999948417,-144.516898051454,
429.537703348572));
#268753=CARTESIAN_POINT('Ctrl Pts',(57.426173453193,-149.931567610411,427.537703348572));
#268754=CARTESIAN_POINT('Ctrl Pts',(45.3454354230638,-153.500330774912,
425.537703348572));
#268755=CARTESIAN_POINT('Ctrl Pts',(33.2646973929347,-157.069093939413,
423.537703348572));
#268756=CARTESIAN_POINT('Ctrl Pts',(20.774415738298,-158.704075916301,421.537703348572));
#268757=CARTESIAN_POINT('Ctrl Pts',(8.28413408366139,-160.339057893189,
419.537703348572));
#268758=CARTESIAN_POINT('Ctrl Pts',(-4.30813900827764,-160.,417.537703348572));
#268759=CARTESIAN_POINT('Ctrl Pts',(-16.9004121002167,-159.660942106811,
415.537703348572));
#268760=CARTESIAN_POINT('Ctrl Pts',(-29.2846130745759,-157.356193074143,
413.537703348572));
#268761=CARTESIAN_POINT('Ctrl Pts',(-41.6688140489351,-155.051444041476,
411.537703348572));
#268762=CARTESIAN_POINT('Ctrl Pts',(-53.5400027769194,-150.837754439537,
409.537703348572));
#268763=CARTESIAN_POINT('Ctrl Pts',(-65.4111915049037,-146.624064837599,
407.537703348572));
#268764=CARTESIAN_POINT('Ctrl Pts',(-76.4770599218133,-140.605189688823,
405.537703348572));
#268765=CARTESIAN_POINT('Ctrl Pts',(-87.5429283387229,-134.586314540048,
403.537703348572));
#268766=CARTESIAN_POINT('Ctrl Pts',(-97.530998038622,-126.9104585261,401.537703348572));
#268767=CARTESIAN_POINT('Ctrl Pts',(-107.519067738521,-119.234602512152,
399.537703348572));
#268768=CARTESIAN_POINT('Ctrl Pts',(-116.183399296895,-110.0907706828,397.537703348572));
#268769=CARTESIAN_POINT('Ctrl Pts',(-124.847730855269,-100.946938853448,
395.537703348572));
#268770=CARTESIAN_POINT('Ctrl Pts',(-131.974979673883,-90.5602826949695,
393.537703348572));
#268771=CARTESIAN_POINT('Ctrl Pts',(-139.102228492497,-80.1736265364905,
391.537703348572));
#268772=CARTESIAN_POINT('Ctrl Pts',(-144.516898051454,-68.7998999948417,
389.537703348572));
#268773=CARTESIAN_POINT('Ctrl Pts',(-149.931567610411,-57.426173453193,
387.537703348572));
#268774=CARTESIAN_POINT('Ctrl Pts',(-153.500330774912,-45.3454354230638,
385.537703348572));
#268775=CARTESIAN_POINT('Ctrl Pts',(-157.069093939413,-33.2646973929347,
383.537703348572));
#268776=CARTESIAN_POINT('Ctrl Pts',(-158.704075916301,-20.774415738298,
381.537703348572));
#268777=CARTESIAN_POINT('Ctrl Pts',(-160.339057893189,-8.2841340836614,
379.537703348572));
#268778=CARTESIAN_POINT('Ctrl Pts',(-160.,4.30813900827767,377.537703348572));
#268779=CARTESIAN_POINT('Ctrl Pts',(-130.,4.30813900827773,537.537703348572));
#268780=CARTESIAN_POINT('Ctrl Pts',(-129.660942106811,14.5393608954781,
535.537703348572));
#268781=CARTESIAN_POINT('Ctrl Pts',(-127.725542856289,24.591579123369,533.537703348572));
#268782=CARTESIAN_POINT('Ctrl Pts',(-125.790143605767,34.6437973512599,
531.537703348572));
#268783=CARTESIAN_POINT('Ctrl Pts',(-122.306058950683,44.269492945671,529.537703348572));
#268784=CARTESIAN_POINT('Ctrl Pts',(-118.821974295598,53.8951885400822,
527.537703348572));
#268785=CARTESIAN_POINT('Ctrl Pts',(-113.874993963172,62.8573449296269,
525.537703348572));
#268786=CARTESIAN_POINT('Ctrl Pts',(-108.928013630747,71.8195013191717,
523.537703348572));
#268787=CARTESIAN_POINT('Ctrl Pts',(-102.639948694852,79.8974404698478,
521.537703348572));
#268788=CARTESIAN_POINT('Ctrl Pts',(-96.3518837589562,87.9753796205239,
519.537703348572));
#268789=CARTESIAN_POINT('Ctrl Pts',(-88.8775672472037,94.9701958612987,
517.537703348572));
#268790=CARTESIAN_POINT('Ctrl Pts',(-81.4032507354512,101.965012102073,
515.537703348572));
#268791=CARTESIAN_POINT('Ctrl Pts',(-72.9267251261952,107.704469842635,
513.537703348572));
#268792=CARTESIAN_POINT('Ctrl Pts',(-64.4501995169392,113.443927583196,
511.537703348572));
#268793=CARTESIAN_POINT('Ctrl Pts',(-55.1801850026552,117.786702325803,
509.537703348572));
#268794=CARTESIAN_POINT('Ctrl Pts',(-45.9101704883713,122.12947706841,507.537703348572));
#268795=CARTESIAN_POINT('Ctrl Pts',(-36.0749255918153,124.968635286057,
505.537703348572));
#268796=CARTESIAN_POINT('Ctrl Pts',(-26.2396806952593,127.807793503704,
503.537703348572));
#268797=CARTESIAN_POINT('Ctrl Pts',(-16.081381787091,129.073425698447,501.537703348572));
#268798=CARTESIAN_POINT('Ctrl Pts',(-5.92308287892268,130.339057893189,
499.537703348572));
#268799=CARTESIAN_POINT('Ctrl Pts',(4.30813900827772,130.,497.537703348572));
#268800=CARTESIAN_POINT('Ctrl Pts',(14.5393608954781,129.660942106811,495.537703348572));
#268801=CARTESIAN_POINT('Ctrl Pts',(24.591579123369,127.725542856289,493.537703348572));
#268802=CARTESIAN_POINT('Ctrl Pts',(34.6437973512599,125.790143605767,491.537703348572));
#268803=CARTESIAN_POINT('Ctrl Pts',(44.269492945671,122.306058950683,489.537703348572));
#268804=CARTESIAN_POINT('Ctrl Pts',(53.8951885400822,118.821974295598,487.537703348572));
#268805=CARTESIAN_POINT('Ctrl Pts',(62.8573449296269,113.874993963172,485.537703348572));
#268806=CARTESIAN_POINT('Ctrl Pts',(71.8195013191717,108.928013630747,483.537703348572));
#268807=CARTESIAN_POINT('Ctrl Pts',(79.8974404698478,102.639948694852,481.537703348572));
#268808=CARTESIAN_POINT('Ctrl Pts',(87.9753796205239,96.3518837589562,479.537703348572));
#268809=CARTESIAN_POINT('Ctrl Pts',(94.9701958612986,88.8775672472037,477.537703348572));
#268810=CARTESIAN_POINT('Ctrl Pts',(101.965012102073,81.4032507354512,475.537703348572));
#268811=CARTESIAN_POINT('Ctrl Pts',(107.704469842635,72.9267251261952,473.537703348572));
#268812=CARTESIAN_POINT('Ctrl Pts',(113.443927583196,64.4501995169392,471.537703348572));
#268813=CARTESIAN_POINT('Ctrl Pts',(117.786702325803,55.1801850026552,469.537703348572));
#268814=CARTESIAN_POINT('Ctrl Pts',(122.12947706841,45.9101704883713,467.537703348572));
#268815=CARTESIAN_POINT('Ctrl Pts',(124.968635286057,36.0749255918153,465.537703348572));
#268816=CARTESIAN_POINT('Ctrl Pts',(127.807793503704,26.2396806952593,463.537703348572));
#268817=CARTESIAN_POINT('Ctrl Pts',(129.073425698447,16.081381787091,461.537703348572));
#268818=CARTESIAN_POINT('Ctrl Pts',(130.339057893189,5.92308287892268,459.537703348572));
#268819=CARTESIAN_POINT('Ctrl Pts',(130.,-4.30813900827772,457.537703348572));
#268820=CARTESIAN_POINT('Ctrl Pts',(129.660942106811,-14.5393608954781,
455.537703348572));
#268821=CARTESIAN_POINT('Ctrl Pts',(127.725542856289,-24.591579123369,453.537703348572));
#268822=CARTESIAN_POINT('Ctrl Pts',(125.790143605767,-34.6437973512599,
451.537703348572));
#268823=CARTESIAN_POINT('Ctrl Pts',(122.306058950683,-44.269492945671,449.537703348572));
#268824=CARTESIAN_POINT('Ctrl Pts',(118.821974295598,-53.8951885400822,
447.537703348572));
#268825=CARTESIAN_POINT('Ctrl Pts',(113.874993963172,-62.8573449296269,
445.537703348572));
#268826=CARTESIAN_POINT('Ctrl Pts',(108.928013630747,-71.8195013191717,
443.537703348572));
#268827=CARTESIAN_POINT('Ctrl Pts',(102.639948694852,-79.8974404698478,
441.537703348572));
#268828=CARTESIAN_POINT('Ctrl Pts',(96.3518837589563,-87.9753796205239,
439.537703348572));
#268829=CARTESIAN_POINT('Ctrl Pts',(88.8775672472037,-94.9701958612986,
437.537703348572));
#268830=CARTESIAN_POINT('Ctrl Pts',(81.4032507354513,-101.965012102073,
435.537703348572));
#268831=CARTESIAN_POINT('Ctrl Pts',(72.9267251261952,-107.704469842635,
433.537703348572));
#268832=CARTESIAN_POINT('Ctrl Pts',(64.4501995169392,-113.443927583196,
431.537703348572));
#268833=CARTESIAN_POINT('Ctrl Pts',(55.1801850026552,-117.786702325803,
429.537703348572));
#268834=CARTESIAN_POINT('Ctrl Pts',(45.9101704883713,-122.12947706841,427.537703348572));
#268835=CARTESIAN_POINT('Ctrl Pts',(36.0749255918153,-124.968635286057,
425.537703348572));
#268836=CARTESIAN_POINT('Ctrl Pts',(26.2396806952593,-127.807793503704,
423.537703348572));
#268837=CARTESIAN_POINT('Ctrl Pts',(16.081381787091,-129.073425698447,421.537703348572));
#268838=CARTESIAN_POINT('Ctrl Pts',(5.92308287892275,-130.339057893189,
419.537703348572));
#268839=CARTESIAN_POINT('Ctrl Pts',(-4.30813900827771,-130.,417.537703348572));
#268840=CARTESIAN_POINT('Ctrl Pts',(-14.5393608954782,-129.660942106811,
415.537703348572));
#268841=CARTESIAN_POINT('Ctrl Pts',(-24.591579123369,-127.725542856289,
413.537703348572));
#268842=CARTESIAN_POINT('Ctrl Pts',(-34.6437973512598,-125.790143605767,
411.537703348572));
#268843=CARTESIAN_POINT('Ctrl Pts',(-44.269492945671,-122.306058950683,
409.537703348572));
#268844=CARTESIAN_POINT('Ctrl Pts',(-53.8951885400822,-118.821974295598,
407.537703348572));
#268845=CARTESIAN_POINT('Ctrl Pts',(-62.8573449296269,-113.874993963172,
405.537703348572));
#268846=CARTESIAN_POINT('Ctrl Pts',(-71.8195013191717,-108.928013630747,
403.537703348572));
#268847=CARTESIAN_POINT('Ctrl Pts',(-79.8974404698478,-102.639948694852,
401.537703348572));
#268848=CARTESIAN_POINT('Ctrl Pts',(-87.975379620524,-96.3518837589562,
399.537703348572));
#268849=CARTESIAN_POINT('Ctrl Pts',(-94.9701958612986,-88.8775672472037,
397.537703348572));
#268850=CARTESIAN_POINT('Ctrl Pts',(-101.965012102073,-81.4032507354513,
395.537703348572));
#268851=CARTESIAN_POINT('Ctrl Pts',(-107.704469842635,-72.9267251261952,
393.537703348572));
#268852=CARTESIAN_POINT('Ctrl Pts',(-113.443927583196,-64.4501995169392,
391.537703348572));
#268853=CARTESIAN_POINT('Ctrl Pts',(-117.786702325803,-55.1801850026553,
389.537703348572));
#268854=CARTESIAN_POINT('Ctrl Pts',(-122.12947706841,-45.9101704883713,
387.537703348572));
#268855=CARTESIAN_POINT('Ctrl Pts',(-124.968635286057,-36.0749255918153,
385.537703348572));
#268856=CARTESIAN_POINT('Ctrl Pts',(-127.807793503704,-26.2396806952593,
383.537703348572));
#268857=CARTESIAN_POINT('Ctrl Pts',(-129.073425698447,-16.081381787091,
381.537703348572));
#268858=CARTESIAN_POINT('Ctrl Pts',(-130.339057893189,-5.92308287892275,
379.537703348572));
#268859=CARTESIAN_POINT('Ctrl Pts',(-130.,4.30813900827773,377.537703348572));
#268860=CARTESIAN_POINT('Ctrl Pts',(-130.,-4.30813900827845,532.462296651428));
#268861=CARTESIAN_POINT('Ctrl Pts',(-130.339057893189,5.92308287892195,
530.462296651429));
#268862=CARTESIAN_POINT('Ctrl Pts',(-129.073425698447,16.0813817870903,
528.462296651428));
#268863=CARTESIAN_POINT('Ctrl Pts',(-127.807793503705,26.2396806952586,
526.462296651429));
#268864=CARTESIAN_POINT('Ctrl Pts',(-124.968635286058,36.0749255918146,
524.462296651428));
#268865=CARTESIAN_POINT('Ctrl Pts',(-122.129477068411,45.9101704883706,
522.462296651428));
#268866=CARTESIAN_POINT('Ctrl Pts',(-117.786702325804,55.1801850026546,
520.462296651428));
#268867=CARTESIAN_POINT('Ctrl Pts',(-113.443927583196,64.4501995169386,
518.462296651428));
#268868=CARTESIAN_POINT('Ctrl Pts',(-107.704469842635,72.9267251261946,
516.462296651428));
#268869=CARTESIAN_POINT('Ctrl Pts',(-101.965012102074,81.4032507354507,
514.462296651428));
#268870=CARTESIAN_POINT('Ctrl Pts',(-94.9701958612992,88.8775672472032,
512.462296651428));
#268871=CARTESIAN_POINT('Ctrl Pts',(-87.9753796205245,96.3518837589558,
510.462296651429));
#268872=CARTESIAN_POINT('Ctrl Pts',(-79.8974404698484,102.639948694851,
508.462296651428));
#268873=CARTESIAN_POINT('Ctrl Pts',(-71.8195013191724,108.928013630747,
506.462296651428));
#268874=CARTESIAN_POINT('Ctrl Pts',(-62.8573449296276,113.874993963172,
504.462296651428));
#268875=CARTESIAN_POINT('Ctrl Pts',(-53.8951885400828,118.821974295598,
502.462296651428));
#268876=CARTESIAN_POINT('Ctrl Pts',(-44.2694929456717,122.306058950682,
500.462296651428));
#268877=CARTESIAN_POINT('Ctrl Pts',(-34.6437973512606,125.790143605767,
498.462296651429));
#268878=CARTESIAN_POINT('Ctrl Pts',(-24.5915791233697,127.725542856289,
496.462296651428));
#268879=CARTESIAN_POINT('Ctrl Pts',(-14.5393608954789,129.660942106811,
494.462296651428));
#268880=CARTESIAN_POINT('Ctrl Pts',(-4.30813900827846,130.,492.462296651428));
#268881=CARTESIAN_POINT('Ctrl Pts',(5.92308287892194,130.339057893189,490.462296651429));
#268882=CARTESIAN_POINT('Ctrl Pts',(16.0813817870903,129.073425698447,488.462296651428));
#268883=CARTESIAN_POINT('Ctrl Pts',(26.2396806952586,127.807793503705,486.462296651428));
#268884=CARTESIAN_POINT('Ctrl Pts',(36.0749255918146,124.968635286058,484.462296651428));
#268885=CARTESIAN_POINT('Ctrl Pts',(45.9101704883706,122.129477068411,482.462296651428));
#268886=CARTESIAN_POINT('Ctrl Pts',(55.1801850026546,117.786702325804,480.462296651428));
#268887=CARTESIAN_POINT('Ctrl Pts',(64.4501995169386,113.443927583196,478.462296651429));
#268888=CARTESIAN_POINT('Ctrl Pts',(72.9267251261946,107.704469842635,476.462296651428));
#268889=CARTESIAN_POINT('Ctrl Pts',(81.4032507354506,101.965012102074,474.462296651428));
#268890=CARTESIAN_POINT('Ctrl Pts',(88.8775672472032,94.9701958612992,472.462296651428));
#268891=CARTESIAN_POINT('Ctrl Pts',(96.3518837589558,87.9753796205245,470.462296651428));
#268892=CARTESIAN_POINT('Ctrl Pts',(102.639948694851,79.8974404698484,468.462296651428));
#268893=CARTESIAN_POINT('Ctrl Pts',(108.928013630747,71.8195013191724,466.462296651428));
#268894=CARTESIAN_POINT('Ctrl Pts',(113.874993963172,62.8573449296276,464.462296651428));
#268895=CARTESIAN_POINT('Ctrl Pts',(118.821974295598,53.8951885400829,462.462296651428));
#268896=CARTESIAN_POINT('Ctrl Pts',(122.306058950682,44.2694929456717,460.462296651428));
#268897=CARTESIAN_POINT('Ctrl Pts',(125.790143605767,34.6437973512606,458.462296651429));
#268898=CARTESIAN_POINT('Ctrl Pts',(127.725542856289,24.5915791233698,456.462296651428));
#268899=CARTESIAN_POINT('Ctrl Pts',(129.660942106811,14.5393608954789,454.462296651429));
#268900=CARTESIAN_POINT('Ctrl Pts',(130.,4.30813900827846,452.462296651428));
#268901=CARTESIAN_POINT('Ctrl Pts',(130.339057893189,-5.92308287892194,
450.462296651428));
#268902=CARTESIAN_POINT('Ctrl Pts',(129.073425698447,-16.0813817870903,
448.462296651429));
#268903=CARTESIAN_POINT('Ctrl Pts',(127.807793503705,-26.2396806952586,
446.462296651429));
#268904=CARTESIAN_POINT('Ctrl Pts',(124.968635286058,-36.0749255918146,
444.462296651429));
#268905=CARTESIAN_POINT('Ctrl Pts',(122.129477068411,-45.9101704883706,
442.462296651429));
#268906=CARTESIAN_POINT('Ctrl Pts',(117.786702325804,-55.1801850026546,
440.462296651428));
#268907=CARTESIAN_POINT('Ctrl Pts',(113.443927583196,-64.4501995169386,
438.462296651429));
#268908=CARTESIAN_POINT('Ctrl Pts',(107.704469842635,-72.9267251261946,
436.462296651428));
#268909=CARTESIAN_POINT('Ctrl Pts',(101.965012102074,-81.4032507354506,
434.462296651429));
#268910=CARTESIAN_POINT('Ctrl Pts',(94.9701958612992,-88.8775672472032,
432.462296651428));
#268911=CARTESIAN_POINT('Ctrl Pts',(87.9753796205246,-96.3518837589557,
430.462296651429));
#268912=CARTESIAN_POINT('Ctrl Pts',(79.8974404698484,-102.639948694851,
428.462296651429));
#268913=CARTESIAN_POINT('Ctrl Pts',(71.8195013191723,-108.928013630747,
426.462296651428));
#268914=CARTESIAN_POINT('Ctrl Pts',(62.8573449296276,-113.874993963172,
424.462296651428));
#268915=CARTESIAN_POINT('Ctrl Pts',(53.8951885400829,-118.821974295598,
422.462296651428));
#268916=CARTESIAN_POINT('Ctrl Pts',(44.2694929456717,-122.306058950682,
420.462296651428));
#268917=CARTESIAN_POINT('Ctrl Pts',(34.6437973512606,-125.790143605767,
418.462296651429));
#268918=CARTESIAN_POINT('Ctrl Pts',(24.5915791233698,-127.725542856289,
416.462296651428));
#268919=CARTESIAN_POINT('Ctrl Pts',(14.5393608954789,-129.660942106811,
414.462296651429));
#268920=CARTESIAN_POINT('Ctrl Pts',(4.30813900827847,-130.,412.462296651428));
#268921=CARTESIAN_POINT('Ctrl Pts',(-5.92308287892199,-130.339057893189,
410.462296651428));
#268922=CARTESIAN_POINT('Ctrl Pts',(-16.0813817870903,-129.073425698447,
408.462296651428));
#268923=CARTESIAN_POINT('Ctrl Pts',(-26.2396806952585,-127.807793503705,
406.462296651429));
#268924=CARTESIAN_POINT('Ctrl Pts',(-36.0749255918146,-124.968635286058,
404.462296651428));
#268925=CARTESIAN_POINT('Ctrl Pts',(-45.9101704883706,-122.129477068411,
402.462296651429));
#268926=CARTESIAN_POINT('Ctrl Pts',(-55.1801850026546,-117.786702325804,
400.462296651428));
#268927=CARTESIAN_POINT('Ctrl Pts',(-64.4501995169385,-113.443927583197,
398.462296651429));
#268928=CARTESIAN_POINT('Ctrl Pts',(-72.9267251261946,-107.704469842635,
396.462296651428));
#268929=CARTESIAN_POINT('Ctrl Pts',(-81.4032507354507,-101.965012102074,
394.462296651429));
#268930=CARTESIAN_POINT('Ctrl Pts',(-88.8775672472032,-94.9701958612992,
392.462296651428));
#268931=CARTESIAN_POINT('Ctrl Pts',(-96.3518837589557,-87.9753796205246,
390.462296651428));
#268932=CARTESIAN_POINT('Ctrl Pts',(-102.639948694851,-79.8974404698484,
388.462296651428));
#268933=CARTESIAN_POINT('Ctrl Pts',(-108.928013630747,-71.8195013191723,
386.462296651428));
#268934=CARTESIAN_POINT('Ctrl Pts',(-113.874993963172,-62.8573449296276,
384.462296651428));
#268935=CARTESIAN_POINT('Ctrl Pts',(-118.821974295598,-53.8951885400829,
382.462296651429));
#268936=CARTESIAN_POINT('Ctrl Pts',(-122.306058950682,-44.2694929456718,
380.462296651428));
#268937=CARTESIAN_POINT('Ctrl Pts',(-125.790143605767,-34.6437973512606,
378.462296651429));
#268938=CARTESIAN_POINT('Ctrl Pts',(-127.725542856289,-24.5915791233698,
376.462296651428));
#268939=CARTESIAN_POINT('Ctrl Pts',(-129.660942106811,-14.5393608954789,
374.462296651428));
#268940=CARTESIAN_POINT('Ctrl Pts',(-130.,-4.30813900827845,372.462296651428));
#268941=CARTESIAN_POINT('Ctrl Pts',(-129.869812400585,7.23822414350004,
536.964207537012));
#268942=CARTESIAN_POINT('Ctrl Pts',(-129.382196958681,15.9871278397991,
535.249654101829));
#268943=CARTESIAN_POINT('Ctrl Pts',(-127.725542856289,24.591579123369,533.537703348572));
#268944=CARTESIAN_POINT('Ctrl Pts',(-125.790143605767,34.6437973512599,
531.537703348572));
#268945=CARTESIAN_POINT('Ctrl Pts',(-122.306058950683,44.269492945671,529.537703348572));
#268946=CARTESIAN_POINT('Ctrl Pts',(-118.821974295598,53.8951885400822,
527.537703348572));
#268947=CARTESIAN_POINT('Ctrl Pts',(-113.874993963172,62.8573449296269,
525.537703348572));
#268948=CARTESIAN_POINT('Ctrl Pts',(-108.928013630747,71.8195013191717,
523.537703348572));
#268949=CARTESIAN_POINT('Ctrl Pts',(-102.639948694852,79.8974404698478,
521.537703348572));
#268950=CARTESIAN_POINT('Ctrl Pts',(-96.3518837589562,87.9753796205239,
519.537703348572));
#268951=CARTESIAN_POINT('Ctrl Pts',(-88.8775672472037,94.9701958612987,
517.537703348572));
#268952=CARTESIAN_POINT('Ctrl Pts',(-81.4032507354512,101.965012102073,
515.537703348572));
#268953=CARTESIAN_POINT('Ctrl Pts',(-72.9267251261952,107.704469842635,
513.537703348572));
#268954=CARTESIAN_POINT('Ctrl Pts',(-64.4501995169392,113.443927583196,
511.537703348572));
#268955=CARTESIAN_POINT('Ctrl Pts',(-55.1801850026552,117.786702325803,
509.537703348572));
#268956=CARTESIAN_POINT('Ctrl Pts',(-45.9101704883713,122.12947706841,507.537703348572));
#268957=CARTESIAN_POINT('Ctrl Pts',(-36.0749255918153,124.968635286057,
505.537703348572));
#268958=CARTESIAN_POINT('Ctrl Pts',(-26.2396806952593,127.807793503704,
503.537703348572));
#268959=CARTESIAN_POINT('Ctrl Pts',(-16.081381787091,129.073425698447,501.537703348572));
#268960=CARTESIAN_POINT('Ctrl Pts',(-5.92308287892268,130.339057893189,
499.537703348572));
#268961=CARTESIAN_POINT('Ctrl Pts',(4.30813900827772,130.,497.537703348572));
#268962=CARTESIAN_POINT('Ctrl Pts',(14.5393608954781,129.660942106811,495.537703348572));
#268963=CARTESIAN_POINT('Ctrl Pts',(24.591579123369,127.725542856289,493.537703348572));
#268964=CARTESIAN_POINT('Ctrl Pts',(34.6437973512599,125.790143605767,491.537703348572));
#268965=CARTESIAN_POINT('Ctrl Pts',(44.269492945671,122.306058950683,489.537703348572));
#268966=CARTESIAN_POINT('Ctrl Pts',(53.8951885400822,118.821974295598,487.537703348572));
#268967=CARTESIAN_POINT('Ctrl Pts',(62.8573449296269,113.874993963172,485.537703348572));
#268968=CARTESIAN_POINT('Ctrl Pts',(71.8195013191717,108.928013630747,483.537703348572));
#268969=CARTESIAN_POINT('Ctrl Pts',(79.8974404698478,102.639948694852,481.537703348572));
#268970=CARTESIAN_POINT('Ctrl Pts',(87.9753796205239,96.3518837589562,479.537703348572));
#268971=CARTESIAN_POINT('Ctrl Pts',(94.9701958612986,88.8775672472037,477.537703348572));
#268972=CARTESIAN_POINT('Ctrl Pts',(101.965012102073,81.4032507354512,475.537703348572));
#268973=CARTESIAN_POINT('Ctrl Pts',(107.704469842635,72.9267251261952,473.537703348572));
#268974=CARTESIAN_POINT('Ctrl Pts',(113.443927583196,64.4501995169392,471.537703348572));
#268975=CARTESIAN_POINT('Ctrl Pts',(117.786702325803,55.1801850026552,469.537703348572));
#268976=CARTESIAN_POINT('Ctrl Pts',(122.12947706841,45.9101704883713,467.537703348572));
#268977=CARTESIAN_POINT('Ctrl Pts',(124.968635286057,36.0749255918153,465.537703348572));
#268978=CARTESIAN_POINT('Ctrl Pts',(127.807793503704,26.2396806952593,463.537703348572));
#268979=CARTESIAN_POINT('Ctrl Pts',(129.073425698447,16.081381787091,461.537703348572));
#268980=CARTESIAN_POINT('Ctrl Pts',(130.339057893189,5.92308287892268,459.537703348572));
#268981=CARTESIAN_POINT('Ctrl Pts',(130.,-4.30813900827772,457.537703348572));
#268982=CARTESIAN_POINT('Ctrl Pts',(129.660942106811,-14.5393608954781,
455.537703348572));
#268983=CARTESIAN_POINT('Ctrl Pts',(127.725542856289,-24.591579123369,453.537703348572));
#268984=CARTESIAN_POINT('Ctrl Pts',(125.790143605767,-34.6437973512599,
451.537703348572));
#268985=CARTESIAN_POINT('Ctrl Pts',(122.306058950683,-44.269492945671,449.537703348572));
#268986=CARTESIAN_POINT('Ctrl Pts',(118.821974295598,-53.8951885400822,
447.537703348572));
#268987=CARTESIAN_POINT('Ctrl Pts',(113.874993963172,-62.8573449296269,
445.537703348572));
#268988=CARTESIAN_POINT('Ctrl Pts',(108.928013630747,-71.8195013191717,
443.537703348572));
#268989=CARTESIAN_POINT('Ctrl Pts',(102.639948694852,-79.8974404698478,
441.537703348572));
#268990=CARTESIAN_POINT('Ctrl Pts',(96.3518837589563,-87.9753796205239,
439.537703348572));
#268991=CARTESIAN_POINT('Ctrl Pts',(88.8775672472037,-94.9701958612986,
437.537703348572));
#268992=CARTESIAN_POINT('Ctrl Pts',(81.4032507354513,-101.965012102073,
435.537703348572));
#268993=CARTESIAN_POINT('Ctrl Pts',(72.9267251261952,-107.704469842635,
433.537703348572));
#268994=CARTESIAN_POINT('Ctrl Pts',(64.4501995169392,-113.443927583196,
431.537703348572));
#268995=CARTESIAN_POINT('Ctrl Pts',(55.1801850026552,-117.786702325803,
429.537703348572));
#268996=CARTESIAN_POINT('Ctrl Pts',(45.9101704883713,-122.12947706841,427.537703348572));
#268997=CARTESIAN_POINT('Ctrl Pts',(36.0749255918153,-124.968635286057,
425.537703348572));
#268998=CARTESIAN_POINT('Ctrl Pts',(26.2396806952593,-127.807793503704,
423.537703348572));
#268999=CARTESIAN_POINT('Ctrl Pts',(16.081381787091,-129.073425698447,421.537703348572));
#269000=CARTESIAN_POINT('Ctrl Pts',(5.92308287892275,-130.339057893189,
419.537703348572));
#269001=CARTESIAN_POINT('Ctrl Pts',(-4.30813900827771,-130.,417.537703348572));
#269002=CARTESIAN_POINT('Ctrl Pts',(-14.5393608954782,-129.660942106811,
415.537703348572));
#269003=CARTESIAN_POINT('Ctrl Pts',(-24.591579123369,-127.725542856289,
413.537703348572));
#269004=CARTESIAN_POINT('Ctrl Pts',(-34.6437973512598,-125.790143605767,
411.537703348572));
#269005=CARTESIAN_POINT('Ctrl Pts',(-44.269492945671,-122.306058950683,
409.537703348572));
#269006=CARTESIAN_POINT('Ctrl Pts',(-53.8951885400822,-118.821974295598,
407.537703348572));
#269007=CARTESIAN_POINT('Ctrl Pts',(-62.8573449296269,-113.874993963172,
405.537703348572));
#269008=CARTESIAN_POINT('Ctrl Pts',(-71.8195013191717,-108.928013630747,
403.537703348572));
#269009=CARTESIAN_POINT('Ctrl Pts',(-79.8974404698478,-102.639948694852,
401.537703348572));
#269010=CARTESIAN_POINT('Ctrl Pts',(-87.975379620524,-96.3518837589562,
399.537703348572));
#269011=CARTESIAN_POINT('Ctrl Pts',(-94.9701958612986,-88.8775672472037,
397.537703348572));
#269012=CARTESIAN_POINT('Ctrl Pts',(-101.965012102073,-81.4032507354513,
395.537703348572));
#269013=CARTESIAN_POINT('Ctrl Pts',(-107.704469842635,-72.9267251261952,
393.537703348572));
#269014=CARTESIAN_POINT('Ctrl Pts',(-113.443927583196,-64.4501995169392,
391.537703348572));
#269015=CARTESIAN_POINT('Ctrl Pts',(-117.786702325803,-55.1801850026553,
389.537703348572));
#269016=CARTESIAN_POINT('Ctrl Pts',(-122.12947706841,-45.9101704883713,
387.537703348572));
#269017=CARTESIAN_POINT('Ctrl Pts',(-124.968635286057,-36.0749255918153,
385.537703348572));
#269018=CARTESIAN_POINT('Ctrl Pts',(-127.807793503704,-26.2396806952593,
383.537703348572));
#269019=CARTESIAN_POINT('Ctrl Pts',(-129.073425698447,-16.081381787091,
381.537703348572));
#269020=CARTESIAN_POINT('Ctrl Pts',(-129.701667605591,-11.038945994199,
380.54493165747));
#269021=CARTESIAN_POINT('Ctrl Pts',(-129.934615416877,-5.962866607847,379.549090218607));
#269022=CARTESIAN_POINT('Ctrl Pts',(-129.934615416877,5.96286660784693,
530.450909781394));
#269023=CARTESIAN_POINT('Ctrl Pts',(-129.701667605591,11.0389459941986,
529.455068342531));
#269024=CARTESIAN_POINT('Ctrl Pts',(-129.073425698447,16.0813817870903,
528.462296651428));
#269025=CARTESIAN_POINT('Ctrl Pts',(-127.807793503705,26.2396806952586,
526.462296651429));
#269026=CARTESIAN_POINT('Ctrl Pts',(-124.968635286058,36.0749255918146,
524.462296651428));
#269027=CARTESIAN_POINT('Ctrl Pts',(-122.129477068411,45.9101704883706,
522.462296651428));
#269028=CARTESIAN_POINT('Ctrl Pts',(-117.786702325804,55.1801850026546,
520.462296651428));
#269029=CARTESIAN_POINT('Ctrl Pts',(-113.443927583196,64.4501995169386,
518.462296651428));
#269030=CARTESIAN_POINT('Ctrl Pts',(-107.704469842635,72.9267251261946,
516.462296651428));
#269031=CARTESIAN_POINT('Ctrl Pts',(-101.965012102074,81.4032507354507,
514.462296651428));
#269032=CARTESIAN_POINT('Ctrl Pts',(-94.9701958612992,88.8775672472032,
512.462296651428));
#269033=CARTESIAN_POINT('Ctrl Pts',(-87.9753796205245,96.3518837589558,
510.462296651429));
#269034=CARTESIAN_POINT('Ctrl Pts',(-79.8974404698484,102.639948694851,
508.462296651428));
#269035=CARTESIAN_POINT('Ctrl Pts',(-71.8195013191724,108.928013630747,
506.462296651428));
#269036=CARTESIAN_POINT('Ctrl Pts',(-62.8573449296276,113.874993963172,
504.462296651428));
#269037=CARTESIAN_POINT('Ctrl Pts',(-53.8951885400828,118.821974295598,
502.462296651429));
#269038=CARTESIAN_POINT('Ctrl Pts',(-44.2694929456717,122.306058950682,
500.462296651428));
#269039=CARTESIAN_POINT('Ctrl Pts',(-34.6437973512606,125.790143605767,
498.462296651429));
#269040=CARTESIAN_POINT('Ctrl Pts',(-24.5915791233697,127.725542856289,
496.462296651428));
#269041=CARTESIAN_POINT('Ctrl Pts',(-14.5393608954789,129.660942106811,
494.462296651429));
#269042=CARTESIAN_POINT('Ctrl Pts',(-4.30813900827846,130.,492.462296651428));
#269043=CARTESIAN_POINT('Ctrl Pts',(5.92308287892194,130.339057893189,490.462296651428));
#269044=CARTESIAN_POINT('Ctrl Pts',(16.0813817870903,129.073425698447,488.462296651428));
#269045=CARTESIAN_POINT('Ctrl Pts',(26.2396806952586,127.807793503705,486.462296651428));
#269046=CARTESIAN_POINT('Ctrl Pts',(36.0749255918146,124.968635286058,484.462296651428));
#269047=CARTESIAN_POINT('Ctrl Pts',(45.9101704883706,122.129477068411,482.462296651428));
#269048=CARTESIAN_POINT('Ctrl Pts',(55.1801850026546,117.786702325804,480.462296651428));
#269049=CARTESIAN_POINT('Ctrl Pts',(64.4501995169386,113.443927583196,478.462296651429));
#269050=CARTESIAN_POINT('Ctrl Pts',(72.9267251261946,107.704469842635,476.462296651428));
#269051=CARTESIAN_POINT('Ctrl Pts',(81.4032507354506,101.965012102074,474.462296651428));
#269052=CARTESIAN_POINT('Ctrl Pts',(88.8775672472032,94.9701958612992,472.462296651428));
#269053=CARTESIAN_POINT('Ctrl Pts',(96.3518837589558,87.9753796205245,470.462296651428));
#269054=CARTESIAN_POINT('Ctrl Pts',(102.639948694851,79.8974404698484,468.462296651428));
#269055=CARTESIAN_POINT('Ctrl Pts',(108.928013630747,71.8195013191724,466.462296651428));
#269056=CARTESIAN_POINT('Ctrl Pts',(113.874993963172,62.8573449296276,464.462296651428));
#269057=CARTESIAN_POINT('Ctrl Pts',(118.821974295598,53.8951885400829,462.462296651428));
#269058=CARTESIAN_POINT('Ctrl Pts',(122.306058950682,44.2694929456717,460.462296651428));
#269059=CARTESIAN_POINT('Ctrl Pts',(125.790143605767,34.6437973512606,458.462296651429));
#269060=CARTESIAN_POINT('Ctrl Pts',(127.725542856289,24.5915791233698,456.462296651428));
#269061=CARTESIAN_POINT('Ctrl Pts',(129.660942106811,14.5393608954789,454.462296651429));
#269062=CARTESIAN_POINT('Ctrl Pts',(130.,4.30813900827846,452.462296651428));
#269063=CARTESIAN_POINT('Ctrl Pts',(130.339057893189,-5.92308287892194,
450.462296651429));
#269064=CARTESIAN_POINT('Ctrl Pts',(129.073425698447,-16.0813817870903,
448.462296651429));
#269065=CARTESIAN_POINT('Ctrl Pts',(127.807793503705,-26.2396806952586,
446.462296651429));
#269066=CARTESIAN_POINT('Ctrl Pts',(124.968635286058,-36.0749255918146,
444.462296651429));
#269067=CARTESIAN_POINT('Ctrl Pts',(122.129477068411,-45.9101704883706,
442.462296651429));
#269068=CARTESIAN_POINT('Ctrl Pts',(117.786702325804,-55.1801850026546,
440.462296651428));
#269069=CARTESIAN_POINT('Ctrl Pts',(113.443927583196,-64.4501995169386,
438.462296651429));
#269070=CARTESIAN_POINT('Ctrl Pts',(107.704469842635,-72.9267251261946,
436.462296651428));
#269071=CARTESIAN_POINT('Ctrl Pts',(101.965012102074,-81.4032507354506,
434.462296651429));
#269072=CARTESIAN_POINT('Ctrl Pts',(94.9701958612992,-88.8775672472032,
432.462296651428));
#269073=CARTESIAN_POINT('Ctrl Pts',(87.9753796205245,-96.3518837589557,
430.462296651429));
#269074=CARTESIAN_POINT('Ctrl Pts',(79.8974404698484,-102.639948694851,
428.462296651429));
#269075=CARTESIAN_POINT('Ctrl Pts',(71.8195013191723,-108.928013630747,
426.462296651428));
#269076=CARTESIAN_POINT('Ctrl Pts',(62.8573449296276,-113.874993963172,
424.462296651428));
#269077=CARTESIAN_POINT('Ctrl Pts',(53.8951885400829,-118.821974295598,
422.462296651428));
#269078=CARTESIAN_POINT('Ctrl Pts',(44.2694929456717,-122.306058950682,
420.462296651428));
#269079=CARTESIAN_POINT('Ctrl Pts',(34.6437973512606,-125.790143605767,
418.462296651429));
#269080=CARTESIAN_POINT('Ctrl Pts',(24.5915791233698,-127.725542856289,
416.462296651428));
#269081=CARTESIAN_POINT('Ctrl Pts',(14.5393608954789,-129.660942106811,
414.462296651429));
#269082=CARTESIAN_POINT('Ctrl Pts',(4.30813900827847,-130.,412.462296651428));
#269083=CARTESIAN_POINT('Ctrl Pts',(-5.92308287892199,-130.339057893189,
410.462296651428));
#269084=CARTESIAN_POINT('Ctrl Pts',(-16.0813817870903,-129.073425698447,
408.462296651428));
#269085=CARTESIAN_POINT('Ctrl Pts',(-26.2396806952585,-127.807793503705,
406.462296651429));
#269086=CARTESIAN_POINT('Ctrl Pts',(-36.0749255918146,-124.968635286058,
404.462296651428));
#269087=CARTESIAN_POINT('Ctrl Pts',(-45.9101704883706,-122.129477068411,
402.462296651428));
#269088=CARTESIAN_POINT('Ctrl Pts',(-55.1801850026546,-117.786702325804,
400.462296651428));
#269089=CARTESIAN_POINT('Ctrl Pts',(-64.4501995169385,-113.443927583197,
398.462296651429));
#269090=CARTESIAN_POINT('Ctrl Pts',(-72.9267251261946,-107.704469842635,
396.462296651428));
#269091=CARTESIAN_POINT('Ctrl Pts',(-81.4032507354507,-101.965012102074,
394.462296651429));
#269092=CARTESIAN_POINT('Ctrl Pts',(-88.8775672472032,-94.9701958612992,
392.462296651428));
#269093=CARTESIAN_POINT('Ctrl Pts',(-96.3518837589557,-87.9753796205245,
390.462296651428));
#269094=CARTESIAN_POINT('Ctrl Pts',(-102.639948694851,-79.8974404698484,
388.462296651428));
#269095=CARTESIAN_POINT('Ctrl Pts',(-108.928013630747,-71.8195013191723,
386.462296651429));
#269096=CARTESIAN_POINT('Ctrl Pts',(-113.874993963172,-62.8573449296276,
384.462296651428));
#269097=CARTESIAN_POINT('Ctrl Pts',(-118.821974295598,-53.8951885400829,
382.462296651429));
#269098=CARTESIAN_POINT('Ctrl Pts',(-122.306058950682,-44.2694929456718,
380.462296651428));
#269099=CARTESIAN_POINT('Ctrl Pts',(-125.790143605767,-34.6437973512606,
378.462296651429));
#269100=CARTESIAN_POINT('Ctrl Pts',(-127.725542856289,-24.5915791233698,
376.462296651428));
#269101=CARTESIAN_POINT('Ctrl Pts',(-129.382196958681,-15.9871278397995,
374.750345898172));
#269102=CARTESIAN_POINT('Ctrl Pts',(-129.869812400585,-7.23822414349998,
373.035792462989));
#269103=CARTESIAN_POINT('Ctrl Pts',(-160.,4.30813900827767,537.537703348572));
#269104=CARTESIAN_POINT('Ctrl Pts',(-159.660942106811,16.9004121002166,
535.537703348572));
#269105=CARTESIAN_POINT('Ctrl Pts',(-157.356193074143,29.2846130745759,
533.537703348572));
#269106=CARTESIAN_POINT('Ctrl Pts',(-155.051444041476,41.6688140489352,
531.537703348572));
#269107=CARTESIAN_POINT('Ctrl Pts',(-150.837754439537,53.5400027769194,
529.537703348572));
#269108=CARTESIAN_POINT('Ctrl Pts',(-146.624064837599,65.4111915049037,
527.537703348572));
#269109=CARTESIAN_POINT('Ctrl Pts',(-140.605189688823,76.4770599218133,
525.537703348572));
#269110=CARTESIAN_POINT('Ctrl Pts',(-134.586314540048,87.542928338723,523.537703348572));
#269111=CARTESIAN_POINT('Ctrl Pts',(-126.9104585261,97.530998038622,521.537703348572));
#269112=CARTESIAN_POINT('Ctrl Pts',(-119.234602512152,107.519067738521,
519.537703348572));
#269113=CARTESIAN_POINT('Ctrl Pts',(-110.0907706828,116.183399296895,517.537703348572));
#269114=CARTESIAN_POINT('Ctrl Pts',(-100.946938853448,124.847730855269,
515.537703348572));
#269115=CARTESIAN_POINT('Ctrl Pts',(-90.5602826949695,131.974979673883,
513.537703348572));
#269116=CARTESIAN_POINT('Ctrl Pts',(-80.1736265364906,139.102228492497,
511.537703348572));
#269117=CARTESIAN_POINT('Ctrl Pts',(-68.7998999948417,144.516898051454,
509.537703348572));
#269118=CARTESIAN_POINT('Ctrl Pts',(-57.4261734531929,149.931567610411,
507.537703348572));
#269119=CARTESIAN_POINT('Ctrl Pts',(-45.3454354230638,153.500330774912,
505.537703348572));
#269120=CARTESIAN_POINT('Ctrl Pts',(-33.2646973929347,157.069093939413,
503.537703348572));
#269121=CARTESIAN_POINT('Ctrl Pts',(-20.774415738298,158.704075916301,501.537703348572));
#269122=CARTESIAN_POINT('Ctrl Pts',(-8.28413408366129,160.339057893189,
499.537703348572));
#269123=CARTESIAN_POINT('Ctrl Pts',(4.30813900827766,160.,497.537703348572));
#269124=CARTESIAN_POINT('Ctrl Pts',(16.9004121002166,159.660942106811,495.537703348572));
#269125=CARTESIAN_POINT('Ctrl Pts',(29.2846130745759,157.356193074143,493.537703348572));
#269126=CARTESIAN_POINT('Ctrl Pts',(41.6688140489352,155.051444041476,491.537703348572));
#269127=CARTESIAN_POINT('Ctrl Pts',(53.5400027769194,150.837754439537,489.537703348572));
#269128=CARTESIAN_POINT('Ctrl Pts',(65.4111915049037,146.624064837599,487.537703348572));
#269129=CARTESIAN_POINT('Ctrl Pts',(76.4770599218133,140.605189688823,485.537703348572));
#269130=CARTESIAN_POINT('Ctrl Pts',(87.542928338723,134.586314540048,483.537703348572));
#269131=CARTESIAN_POINT('Ctrl Pts',(97.530998038622,126.9104585261,481.537703348572));
#269132=CARTESIAN_POINT('Ctrl Pts',(107.519067738521,119.234602512152,479.537703348572));
#269133=CARTESIAN_POINT('Ctrl Pts',(116.183399296895,110.0907706828,477.537703348572));
#269134=CARTESIAN_POINT('Ctrl Pts',(124.847730855269,100.946938853448,475.537703348572));
#269135=CARTESIAN_POINT('Ctrl Pts',(131.974979673883,90.5602826949695,473.537703348572));
#269136=CARTESIAN_POINT('Ctrl Pts',(139.102228492497,80.1736265364906,471.537703348572));
#269137=CARTESIAN_POINT('Ctrl Pts',(144.516898051454,68.7998999948417,469.537703348572));
#269138=CARTESIAN_POINT('Ctrl Pts',(149.931567610411,57.4261734531929,467.537703348572));
#269139=CARTESIAN_POINT('Ctrl Pts',(153.500330774912,45.3454354230638,465.537703348572));
#269140=CARTESIAN_POINT('Ctrl Pts',(157.069093939413,33.2646973929347,463.537703348572));
#269141=CARTESIAN_POINT('Ctrl Pts',(158.704075916301,20.774415738298,461.537703348572));
#269142=CARTESIAN_POINT('Ctrl Pts',(160.339057893189,8.28413408366131,459.537703348572));
#269143=CARTESIAN_POINT('Ctrl Pts',(160.,-4.30813900827765,457.537703348572));
#269144=CARTESIAN_POINT('Ctrl Pts',(159.660942106811,-16.9004121002166,
455.537703348572));
#269145=CARTESIAN_POINT('Ctrl Pts',(157.356193074143,-29.2846130745759,
453.537703348572));
#269146=CARTESIAN_POINT('Ctrl Pts',(155.051444041476,-41.6688140489352,
451.537703348572));
#269147=CARTESIAN_POINT('Ctrl Pts',(150.837754439537,-53.5400027769194,
449.537703348572));
#269148=CARTESIAN_POINT('Ctrl Pts',(146.624064837599,-65.4111915049036,
447.537703348572));
#269149=CARTESIAN_POINT('Ctrl Pts',(140.605189688823,-76.4770599218133,
445.537703348572));
#269150=CARTESIAN_POINT('Ctrl Pts',(134.586314540048,-87.5429283387229,
443.537703348572));
#269151=CARTESIAN_POINT('Ctrl Pts',(126.9104585261,-97.530998038622,441.537703348572));
#269152=CARTESIAN_POINT('Ctrl Pts',(119.234602512152,-107.519067738521,
439.537703348572));
#269153=CARTESIAN_POINT('Ctrl Pts',(110.0907706828,-116.183399296895,437.537703348572));
#269154=CARTESIAN_POINT('Ctrl Pts',(100.946938853448,-124.847730855269,
435.537703348572));
#269155=CARTESIAN_POINT('Ctrl Pts',(90.5602826949695,-131.974979673883,
433.537703348572));
#269156=CARTESIAN_POINT('Ctrl Pts',(80.1736265364905,-139.102228492497,
431.537703348572));
#269157=CARTESIAN_POINT('Ctrl Pts',(68.7998999948417,-144.516898051454,
429.537703348572));
#269158=CARTESIAN_POINT('Ctrl Pts',(57.426173453193,-149.931567610411,427.537703348572));
#269159=CARTESIAN_POINT('Ctrl Pts',(45.3454354230638,-153.500330774912,
425.537703348572));
#269160=CARTESIAN_POINT('Ctrl Pts',(33.2646973929347,-157.069093939413,
423.537703348572));
#269161=CARTESIAN_POINT('Ctrl Pts',(20.774415738298,-158.704075916301,421.537703348572));
#269162=CARTESIAN_POINT('Ctrl Pts',(8.28413408366139,-160.339057893189,
419.537703348572));
#269163=CARTESIAN_POINT('Ctrl Pts',(-4.30813900827764,-160.,417.537703348572));
#269164=CARTESIAN_POINT('Ctrl Pts',(-16.9004121002167,-159.660942106811,
415.537703348572));
#269165=CARTESIAN_POINT('Ctrl Pts',(-29.2846130745759,-157.356193074143,
413.537703348572));
#269166=CARTESIAN_POINT('Ctrl Pts',(-41.6688140489351,-155.051444041476,
411.537703348572));
#269167=CARTESIAN_POINT('Ctrl Pts',(-53.5400027769194,-150.837754439537,
409.537703348572));
#269168=CARTESIAN_POINT('Ctrl Pts',(-65.4111915049037,-146.624064837599,
407.537703348572));
#269169=CARTESIAN_POINT('Ctrl Pts',(-76.4770599218133,-140.605189688823,
405.537703348572));
#269170=CARTESIAN_POINT('Ctrl Pts',(-87.5429283387229,-134.586314540048,
403.537703348572));
#269171=CARTESIAN_POINT('Ctrl Pts',(-97.530998038622,-126.9104585261,401.537703348572));
#269172=CARTESIAN_POINT('Ctrl Pts',(-107.519067738521,-119.234602512152,
399.537703348572));
#269173=CARTESIAN_POINT('Ctrl Pts',(-116.183399296895,-110.0907706828,397.537703348572));
#269174=CARTESIAN_POINT('Ctrl Pts',(-124.847730855269,-100.946938853448,
395.537703348572));
#269175=CARTESIAN_POINT('Ctrl Pts',(-131.974979673883,-90.5602826949695,
393.537703348572));
#269176=CARTESIAN_POINT('Ctrl Pts',(-139.102228492497,-80.1736265364905,
391.537703348572));
#269177=CARTESIAN_POINT('Ctrl Pts',(-144.516898051454,-68.7998999948417,
389.537703348572));
#269178=CARTESIAN_POINT('Ctrl Pts',(-149.931567610411,-57.426173453193,
387.537703348572));
#269179=CARTESIAN_POINT('Ctrl Pts',(-153.500330774912,-45.3454354230638,
385.537703348572));
#269180=CARTESIAN_POINT('Ctrl Pts',(-157.069093939413,-33.2646973929347,
383.537703348572));
#269181=CARTESIAN_POINT('Ctrl Pts',(-158.704075916301,-20.774415738298,
381.537703348572));
#269182=CARTESIAN_POINT('Ctrl Pts',(-160.339057893189,-8.2841340836614,
379.537703348572));
#269183=CARTESIAN_POINT('Ctrl Pts',(-160.,4.30813900827767,377.537703348572));
#269184=CARTESIAN_POINT('Ctrl Pts',(-130.,4.30813900827773,537.537703348572));
#269185=CARTESIAN_POINT('Ctrl Pts',(-129.660942106811,14.5393608954781,
535.537703348572));
#269186=CARTESIAN_POINT('Ctrl Pts',(-127.725542856289,24.591579123369,533.537703348572));
#269187=CARTESIAN_POINT('Ctrl Pts',(-125.790143605767,34.6437973512599,
531.537703348572));
#269188=CARTESIAN_POINT('Ctrl Pts',(-122.306058950683,44.269492945671,529.537703348572));
#269189=CARTESIAN_POINT('Ctrl Pts',(-118.821974295598,53.8951885400822,
527.537703348572));
#269190=CARTESIAN_POINT('Ctrl Pts',(-113.874993963172,62.8573449296269,
525.537703348572));
#269191=CARTESIAN_POINT('Ctrl Pts',(-108.928013630747,71.8195013191717,
523.537703348572));
#269192=CARTESIAN_POINT('Ctrl Pts',(-102.639948694852,79.8974404698478,
521.537703348572));
#269193=CARTESIAN_POINT('Ctrl Pts',(-96.3518837589562,87.9753796205239,
519.537703348572));
#269194=CARTESIAN_POINT('Ctrl Pts',(-88.8775672472037,94.9701958612987,
517.537703348572));
#269195=CARTESIAN_POINT('Ctrl Pts',(-81.4032507354512,101.965012102073,
515.537703348572));
#269196=CARTESIAN_POINT('Ctrl Pts',(-72.9267251261952,107.704469842635,
513.537703348572));
#269197=CARTESIAN_POINT('Ctrl Pts',(-64.4501995169392,113.443927583196,
511.537703348572));
#269198=CARTESIAN_POINT('Ctrl Pts',(-55.1801850026552,117.786702325803,
509.537703348572));
#269199=CARTESIAN_POINT('Ctrl Pts',(-45.9101704883713,122.12947706841,507.537703348572));
#269200=CARTESIAN_POINT('Ctrl Pts',(-36.0749255918153,124.968635286057,
505.537703348572));
#269201=CARTESIAN_POINT('Ctrl Pts',(-26.2396806952593,127.807793503704,
503.537703348572));
#269202=CARTESIAN_POINT('Ctrl Pts',(-16.081381787091,129.073425698447,501.537703348572));
#269203=CARTESIAN_POINT('Ctrl Pts',(-5.92308287892268,130.339057893189,
499.537703348572));
#269204=CARTESIAN_POINT('Ctrl Pts',(4.30813900827772,130.,497.537703348572));
#269205=CARTESIAN_POINT('Ctrl Pts',(14.5393608954781,129.660942106811,495.537703348572));
#269206=CARTESIAN_POINT('Ctrl Pts',(24.591579123369,127.725542856289,493.537703348572));
#269207=CARTESIAN_POINT('Ctrl Pts',(34.6437973512599,125.790143605767,491.537703348572));
#269208=CARTESIAN_POINT('Ctrl Pts',(44.269492945671,122.306058950683,489.537703348572));
#269209=CARTESIAN_POINT('Ctrl Pts',(53.8951885400822,118.821974295598,487.537703348572));
#269210=CARTESIAN_POINT('Ctrl Pts',(62.8573449296269,113.874993963172,485.537703348572));
#269211=CARTESIAN_POINT('Ctrl Pts',(71.8195013191717,108.928013630747,483.537703348572));
#269212=CARTESIAN_POINT('Ctrl Pts',(79.8974404698478,102.639948694852,481.537703348572));
#269213=CARTESIAN_POINT('Ctrl Pts',(87.9753796205239,96.3518837589562,479.537703348572));
#269214=CARTESIAN_POINT('Ctrl Pts',(94.9701958612986,88.8775672472037,477.537703348572));
#269215=CARTESIAN_POINT('Ctrl Pts',(101.965012102073,81.4032507354512,475.537703348572));
#269216=CARTESIAN_POINT('Ctrl Pts',(107.704469842635,72.9267251261952,473.537703348572));
#269217=CARTESIAN_POINT('Ctrl Pts',(113.443927583196,64.4501995169392,471.537703348572));
#269218=CARTESIAN_POINT('Ctrl Pts',(117.786702325803,55.1801850026552,469.537703348572));
#269219=CARTESIAN_POINT('Ctrl Pts',(122.12947706841,45.9101704883713,467.537703348572));
#269220=CARTESIAN_POINT('Ctrl Pts',(124.968635286057,36.0749255918153,465.537703348572));
#269221=CARTESIAN_POINT('Ctrl Pts',(127.807793503704,26.2396806952593,463.537703348572));
#269222=CARTESIAN_POINT('Ctrl Pts',(129.073425698447,16.081381787091,461.537703348572));
#269223=CARTESIAN_POINT('Ctrl Pts',(130.339057893189,5.92308287892268,459.537703348572));
#269224=CARTESIAN_POINT('Ctrl Pts',(130.,-4.30813900827772,457.537703348572));
#269225=CARTESIAN_POINT('Ctrl Pts',(129.660942106811,-14.5393608954781,
455.537703348572));
#269226=CARTESIAN_POINT('Ctrl Pts',(127.725542856289,-24.591579123369,453.537703348572));
#269227=CARTESIAN_POINT('Ctrl Pts',(125.790143605767,-34.6437973512599,
451.537703348572));
#269228=CARTESIAN_POINT('Ctrl Pts',(122.306058950683,-44.269492945671,449.537703348572));
#269229=CARTESIAN_POINT('Ctrl Pts',(118.821974295598,-53.8951885400822,
447.537703348572));
#269230=CARTESIAN_POINT('Ctrl Pts',(113.874993963172,-62.8573449296269,
445.537703348572));
#269231=CARTESIAN_POINT('Ctrl Pts',(108.928013630747,-71.8195013191717,
443.537703348572));
#269232=CARTESIAN_POINT('Ctrl Pts',(102.639948694852,-79.8974404698478,
441.537703348572));
#269233=CARTESIAN_POINT('Ctrl Pts',(96.3518837589563,-87.9753796205239,
439.537703348572));
#269234=CARTESIAN_POINT('Ctrl Pts',(88.8775672472037,-94.9701958612986,
437.537703348572));
#269235=CARTESIAN_POINT('Ctrl Pts',(81.4032507354513,-101.965012102073,
435.537703348572));
#269236=CARTESIAN_POINT('Ctrl Pts',(72.9267251261952,-107.704469842635,
433.537703348572));
#269237=CARTESIAN_POINT('Ctrl Pts',(64.4501995169392,-113.443927583196,
431.537703348572));
#269238=CARTESIAN_POINT('Ctrl Pts',(55.1801850026552,-117.786702325803,
429.537703348572));
#269239=CARTESIAN_POINT('Ctrl Pts',(45.9101704883713,-122.12947706841,427.537703348572));
#269240=CARTESIAN_POINT('Ctrl Pts',(36.0749255918153,-124.968635286057,
425.537703348572));
#269241=CARTESIAN_POINT('Ctrl Pts',(26.2396806952593,-127.807793503704,
423.537703348572));
#269242=CARTESIAN_POINT('Ctrl Pts',(16.081381787091,-129.073425698447,421.537703348572));
#269243=CARTESIAN_POINT('Ctrl Pts',(5.92308287892275,-130.339057893189,
419.537703348572));
#269244=CARTESIAN_POINT('Ctrl Pts',(-4.30813900827771,-130.,417.537703348572));
#269245=CARTESIAN_POINT('Ctrl Pts',(-14.5393608954782,-129.660942106811,
415.537703348572));
#269246=CARTESIAN_POINT('Ctrl Pts',(-24.591579123369,-127.725542856289,
413.537703348572));
#269247=CARTESIAN_POINT('Ctrl Pts',(-34.6437973512598,-125.790143605767,
411.537703348572));
#269248=CARTESIAN_POINT('Ctrl Pts',(-44.269492945671,-122.306058950683,
409.537703348572));
#269249=CARTESIAN_POINT('Ctrl Pts',(-53.8951885400822,-118.821974295598,
407.537703348572));
#269250=CARTESIAN_POINT('Ctrl Pts',(-62.8573449296269,-113.874993963172,
405.537703348572));
#269251=CARTESIAN_POINT('Ctrl Pts',(-71.8195013191717,-108.928013630747,
403.537703348572));
#269252=CARTESIAN_POINT('Ctrl Pts',(-79.8974404698478,-102.639948694852,
401.537703348572));
#269253=CARTESIAN_POINT('Ctrl Pts',(-87.975379620524,-96.3518837589562,
399.537703348572));
#269254=CARTESIAN_POINT('Ctrl Pts',(-94.9701958612986,-88.8775672472037,
397.537703348572));
#269255=CARTESIAN_POINT('Ctrl Pts',(-101.965012102073,-81.4032507354513,
395.537703348572));
#269256=CARTESIAN_POINT('Ctrl Pts',(-107.704469842635,-72.9267251261952,
393.537703348572));
#269257=CARTESIAN_POINT('Ctrl Pts',(-113.443927583196,-64.4501995169392,
391.537703348572));
#269258=CARTESIAN_POINT('Ctrl Pts',(-117.786702325803,-55.1801850026553,
389.537703348572));
#269259=CARTESIAN_POINT('Ctrl Pts',(-122.12947706841,-45.9101704883713,
387.537703348572));
#269260=CARTESIAN_POINT('Ctrl Pts',(-124.968635286057,-36.0749255918153,
385.537703348572));
#269261=CARTESIAN_POINT('Ctrl Pts',(-127.807793503704,-26.2396806952593,
383.537703348572));
#269262=CARTESIAN_POINT('Ctrl Pts',(-129.073425698447,-16.081381787091,
381.537703348572));
#269263=CARTESIAN_POINT('Ctrl Pts',(-130.339057893189,-5.92308287892275,
379.537703348572));
#269264=CARTESIAN_POINT('Ctrl Pts',(-130.,4.30813900827773,377.537703348572));
#269265=CARTESIAN_POINT('Ctrl Pts',(-159.895664541343,7.20669984090294,
537.076891283416));
#269266=CARTESIAN_POINT('Ctrl Pts',(-159.394142202012,18.3340187941078,
535.306181476978));
#269267=CARTESIAN_POINT('Ctrl Pts',(-157.356193074143,29.2846130745759,
533.537703348572));
#269268=CARTESIAN_POINT('Ctrl Pts',(-155.051444041476,41.6688140489352,
531.537703348572));
#269269=CARTESIAN_POINT('Ctrl Pts',(-150.837754439537,53.5400027769194,
529.537703348572));
#269270=CARTESIAN_POINT('Ctrl Pts',(-146.624064837599,65.4111915049037,
527.537703348572));
#269271=CARTESIAN_POINT('Ctrl Pts',(-140.605189688823,76.4770599218133,
525.537703348572));
#269272=CARTESIAN_POINT('Ctrl Pts',(-134.586314540048,87.542928338723,523.537703348572));
#269273=CARTESIAN_POINT('Ctrl Pts',(-126.9104585261,97.530998038622,521.537703348572));
#269274=CARTESIAN_POINT('Ctrl Pts',(-119.234602512152,107.519067738521,
519.537703348572));
#269275=CARTESIAN_POINT('Ctrl Pts',(-110.0907706828,116.183399296895,517.537703348572));
#269276=CARTESIAN_POINT('Ctrl Pts',(-100.946938853448,124.847730855269,
515.537703348572));
#269277=CARTESIAN_POINT('Ctrl Pts',(-90.5602826949695,131.974979673883,
513.537703348572));
#269278=CARTESIAN_POINT('Ctrl Pts',(-80.1736265364906,139.102228492497,
511.537703348572));
#269279=CARTESIAN_POINT('Ctrl Pts',(-68.7998999948417,144.516898051454,
509.537703348572));
#269280=CARTESIAN_POINT('Ctrl Pts',(-57.4261734531929,149.931567610411,
507.537703348572));
#269281=CARTESIAN_POINT('Ctrl Pts',(-45.3454354230638,153.500330774912,
505.537703348572));
#269282=CARTESIAN_POINT('Ctrl Pts',(-33.2646973929347,157.069093939413,
503.537703348572));
#269283=CARTESIAN_POINT('Ctrl Pts',(-20.774415738298,158.704075916301,501.537703348572));
#269284=CARTESIAN_POINT('Ctrl Pts',(-8.28413408366129,160.339057893189,
499.537703348572));
#269285=CARTESIAN_POINT('Ctrl Pts',(4.30813900827766,160.,497.537703348572));
#269286=CARTESIAN_POINT('Ctrl Pts',(16.9004121002166,159.660942106811,495.537703348572));
#269287=CARTESIAN_POINT('Ctrl Pts',(29.2846130745759,157.356193074143,493.537703348572));
#269288=CARTESIAN_POINT('Ctrl Pts',(41.6688140489352,155.051444041476,491.537703348572));
#269289=CARTESIAN_POINT('Ctrl Pts',(53.5400027769194,150.837754439537,489.537703348572));
#269290=CARTESIAN_POINT('Ctrl Pts',(65.4111915049037,146.624064837599,487.537703348572));
#269291=CARTESIAN_POINT('Ctrl Pts',(76.4770599218133,140.605189688823,485.537703348572));
#269292=CARTESIAN_POINT('Ctrl Pts',(87.542928338723,134.586314540048,483.537703348572));
#269293=CARTESIAN_POINT('Ctrl Pts',(97.530998038622,126.9104585261,481.537703348572));
#269294=CARTESIAN_POINT('Ctrl Pts',(107.519067738521,119.234602512152,479.537703348572));
#269295=CARTESIAN_POINT('Ctrl Pts',(116.183399296895,110.0907706828,477.537703348572));
#269296=CARTESIAN_POINT('Ctrl Pts',(124.847730855269,100.946938853448,475.537703348572));
#269297=CARTESIAN_POINT('Ctrl Pts',(131.974979673883,90.5602826949695,473.537703348572));
#269298=CARTESIAN_POINT('Ctrl Pts',(139.102228492497,80.1736265364906,471.537703348572));
#269299=CARTESIAN_POINT('Ctrl Pts',(144.516898051454,68.7998999948417,469.537703348572));
#269300=CARTESIAN_POINT('Ctrl Pts',(149.931567610411,57.4261734531929,467.537703348572));
#269301=CARTESIAN_POINT('Ctrl Pts',(153.500330774912,45.3454354230638,465.537703348572));
#269302=CARTESIAN_POINT('Ctrl Pts',(157.069093939413,33.2646973929347,463.537703348572));
#269303=CARTESIAN_POINT('Ctrl Pts',(158.704075916301,20.774415738298,461.537703348572));
#269304=CARTESIAN_POINT('Ctrl Pts',(160.339057893189,8.28413408366131,459.537703348572));
#269305=CARTESIAN_POINT('Ctrl Pts',(160.,-4.30813900827765,457.537703348572));
#269306=CARTESIAN_POINT('Ctrl Pts',(159.660942106811,-16.9004121002166,
455.537703348572));
#269307=CARTESIAN_POINT('Ctrl Pts',(157.356193074143,-29.2846130745759,
453.537703348572));
#269308=CARTESIAN_POINT('Ctrl Pts',(155.051444041476,-41.6688140489352,
451.537703348572));
#269309=CARTESIAN_POINT('Ctrl Pts',(150.837754439537,-53.5400027769194,
449.537703348572));
#269310=CARTESIAN_POINT('Ctrl Pts',(146.624064837599,-65.4111915049036,
447.537703348572));
#269311=CARTESIAN_POINT('Ctrl Pts',(140.605189688823,-76.4770599218133,
445.537703348572));
#269312=CARTESIAN_POINT('Ctrl Pts',(134.586314540048,-87.5429283387229,
443.537703348572));
#269313=CARTESIAN_POINT('Ctrl Pts',(126.9104585261,-97.530998038622,441.537703348572));
#269314=CARTESIAN_POINT('Ctrl Pts',(119.234602512152,-107.519067738521,
439.537703348572));
#269315=CARTESIAN_POINT('Ctrl Pts',(110.0907706828,-116.183399296895,437.537703348572));
#269316=CARTESIAN_POINT('Ctrl Pts',(100.946938853448,-124.847730855269,
435.537703348572));
#269317=CARTESIAN_POINT('Ctrl Pts',(90.5602826949695,-131.974979673883,
433.537703348572));
#269318=CARTESIAN_POINT('Ctrl Pts',(80.1736265364905,-139.102228492497,
431.537703348572));
#269319=CARTESIAN_POINT('Ctrl Pts',(68.7998999948417,-144.516898051454,
429.537703348572));
#269320=CARTESIAN_POINT('Ctrl Pts',(57.426173453193,-149.931567610411,427.537703348572));
#269321=CARTESIAN_POINT('Ctrl Pts',(45.3454354230638,-153.500330774912,
425.537703348572));
#269322=CARTESIAN_POINT('Ctrl Pts',(33.2646973929347,-157.069093939413,
423.537703348572));
#269323=CARTESIAN_POINT('Ctrl Pts',(20.774415738298,-158.704075916301,421.537703348572));
#269324=CARTESIAN_POINT('Ctrl Pts',(8.28413408366139,-160.339057893189,
419.537703348572));
#269325=CARTESIAN_POINT('Ctrl Pts',(-4.30813900827764,-160.,417.537703348572));
#269326=CARTESIAN_POINT('Ctrl Pts',(-16.9004121002167,-159.660942106811,
415.537703348572));
#269327=CARTESIAN_POINT('Ctrl Pts',(-29.2846130745759,-157.356193074143,
413.537703348572));
#269328=CARTESIAN_POINT('Ctrl Pts',(-41.6688140489351,-155.051444041476,
411.537703348572));
#269329=CARTESIAN_POINT('Ctrl Pts',(-53.5400027769194,-150.837754439537,
409.537703348572));
#269330=CARTESIAN_POINT('Ctrl Pts',(-65.4111915049037,-146.624064837599,
407.537703348572));
#269331=CARTESIAN_POINT('Ctrl Pts',(-76.4770599218133,-140.605189688823,
405.537703348572));
#269332=CARTESIAN_POINT('Ctrl Pts',(-87.5429283387229,-134.586314540048,
403.537703348572));
#269333=CARTESIAN_POINT('Ctrl Pts',(-97.530998038622,-126.9104585261,401.537703348572));
#269334=CARTESIAN_POINT('Ctrl Pts',(-107.519067738521,-119.234602512152,
399.537703348572));
#269335=CARTESIAN_POINT('Ctrl Pts',(-116.183399296895,-110.0907706828,397.537703348572));
#269336=CARTESIAN_POINT('Ctrl Pts',(-124.847730855269,-100.946938853448,
395.537703348572));
#269337=CARTESIAN_POINT('Ctrl Pts',(-131.974979673883,-90.5602826949695,
393.537703348572));
#269338=CARTESIAN_POINT('Ctrl Pts',(-139.102228492497,-80.1736265364905,
391.537703348572));
#269339=CARTESIAN_POINT('Ctrl Pts',(-144.516898051454,-68.7998999948417,
389.537703348572));
#269340=CARTESIAN_POINT('Ctrl Pts',(-149.931567610411,-57.426173453193,
387.537703348572));
#269341=CARTESIAN_POINT('Ctrl Pts',(-153.500330774912,-45.3454354230638,
385.537703348572));
#269342=CARTESIAN_POINT('Ctrl Pts',(-157.069093939413,-33.2646973929347,
383.537703348572));
#269343=CARTESIAN_POINT('Ctrl Pts',(-158.704075916301,-20.774415738298,
381.537703348572));
#269344=CARTESIAN_POINT('Ctrl Pts',(-159.653854600275,-13.5186762622036,
380.375881753716));
#269345=CARTESIAN_POINT('Ctrl Pts',(-159.937609420477,-6.20654127333065,
379.210563551645));
#269346=CARTESIAN_POINT('Ctrl Pts',(-160.,-4.30813900827851,532.462296651429));
#269347=CARTESIAN_POINT('Ctrl Pts',(-160.339057893189,8.28413408366045,
530.462296651429));
#269348=CARTESIAN_POINT('Ctrl Pts',(-158.704075916301,20.7744157382972,
528.462296651429));
#269349=CARTESIAN_POINT('Ctrl Pts',(-157.069093939413,33.2646973929339,
526.462296651429));
#269350=CARTESIAN_POINT('Ctrl Pts',(-153.500330774912,45.345435423063,524.462296651428));
#269351=CARTESIAN_POINT('Ctrl Pts',(-149.931567610412,57.4261734531921,
522.462296651429));
#269352=CARTESIAN_POINT('Ctrl Pts',(-144.516898051455,68.7998999948409,
520.462296651428));
#269353=CARTESIAN_POINT('Ctrl Pts',(-139.102228492498,80.1736265364898,
518.462296651428));
#269354=CARTESIAN_POINT('Ctrl Pts',(-131.974979673884,90.5602826949688,
516.462296651428));
#269355=CARTESIAN_POINT('Ctrl Pts',(-124.84773085527,100.946938853448,514.462296651429));
#269356=CARTESIAN_POINT('Ctrl Pts',(-116.183399296896,110.0907706828,512.462296651428));
#269357=CARTESIAN_POINT('Ctrl Pts',(-107.519067738522,119.234602512151,
510.462296651429));
#269358=CARTESIAN_POINT('Ctrl Pts',(-97.5309980386227,126.9104585261,508.462296651429));
#269359=CARTESIAN_POINT('Ctrl Pts',(-87.5429283387237,134.586314540048,
506.462296651428));
#269360=CARTESIAN_POINT('Ctrl Pts',(-76.4770599218141,140.605189688823,
504.462296651429));
#269361=CARTESIAN_POINT('Ctrl Pts',(-65.4111915049045,146.624064837598,
502.462296651429));
#269362=CARTESIAN_POINT('Ctrl Pts',(-53.5400027769202,150.837754439537,
500.462296651429));
#269363=CARTESIAN_POINT('Ctrl Pts',(-41.668814048936,155.051444041475,498.462296651429));
#269364=CARTESIAN_POINT('Ctrl Pts',(-29.2846130745767,157.356193074143,
496.462296651429));
#269365=CARTESIAN_POINT('Ctrl Pts',(-16.9004121002175,159.660942106811,
494.462296651429));
#269366=CARTESIAN_POINT('Ctrl Pts',(-4.30813900827852,160.,492.462296651428));
#269367=CARTESIAN_POINT('Ctrl Pts',(8.28413408366043,160.339057893189,490.462296651429));
#269368=CARTESIAN_POINT('Ctrl Pts',(20.7744157382972,158.704075916301,488.462296651429));
#269369=CARTESIAN_POINT('Ctrl Pts',(33.2646973929339,157.069093939413,486.462296651429));
#269370=CARTESIAN_POINT('Ctrl Pts',(45.345435423063,153.500330774912,484.462296651429));
#269371=CARTESIAN_POINT('Ctrl Pts',(57.4261734531921,149.931567610412,482.462296651429));
#269372=CARTESIAN_POINT('Ctrl Pts',(68.7998999948409,144.516898051455,480.462296651428));
#269373=CARTESIAN_POINT('Ctrl Pts',(80.1736265364898,139.102228492498,478.462296651429));
#269374=CARTESIAN_POINT('Ctrl Pts',(90.5602826949688,131.974979673884,476.462296651428));
#269375=CARTESIAN_POINT('Ctrl Pts',(100.946938853448,124.84773085527,474.462296651429));
#269376=CARTESIAN_POINT('Ctrl Pts',(110.0907706828,116.183399296896,472.462296651429));
#269377=CARTESIAN_POINT('Ctrl Pts',(119.234602512151,107.519067738522,470.462296651429));
#269378=CARTESIAN_POINT('Ctrl Pts',(126.9104585261,97.5309980386227,468.462296651429));
#269379=CARTESIAN_POINT('Ctrl Pts',(134.586314540048,87.5429283387237,466.462296651429));
#269380=CARTESIAN_POINT('Ctrl Pts',(140.605189688823,76.4770599218141,464.462296651429));
#269381=CARTESIAN_POINT('Ctrl Pts',(146.624064837598,65.4111915049045,462.462296651429));
#269382=CARTESIAN_POINT('Ctrl Pts',(150.837754439537,53.5400027769202,460.462296651429));
#269383=CARTESIAN_POINT('Ctrl Pts',(155.051444041475,41.668814048936,458.462296651429));
#269384=CARTESIAN_POINT('Ctrl Pts',(157.356193074143,29.2846130745767,456.462296651429));
#269385=CARTESIAN_POINT('Ctrl Pts',(159.660942106811,16.9004121002175,454.462296651429));
#269386=CARTESIAN_POINT('Ctrl Pts',(160.,4.30813900827853,452.462296651429));
#269387=CARTESIAN_POINT('Ctrl Pts',(160.339057893189,-8.28413408366043,
450.462296651429));
#269388=CARTESIAN_POINT('Ctrl Pts',(158.704075916301,-20.7744157382971,
448.462296651429));
#269389=CARTESIAN_POINT('Ctrl Pts',(157.069093939413,-33.2646973929339,
446.462296651429));
#269390=CARTESIAN_POINT('Ctrl Pts',(153.500330774912,-45.345435423063,444.462296651429));
#269391=CARTESIAN_POINT('Ctrl Pts',(149.931567610412,-57.4261734531921,
442.462296651429));
#269392=CARTESIAN_POINT('Ctrl Pts',(144.516898051455,-68.7998999948409,
440.462296651429));
#269393=CARTESIAN_POINT('Ctrl Pts',(139.102228492498,-80.1736265364898,
438.462296651429));
#269394=CARTESIAN_POINT('Ctrl Pts',(131.974979673884,-90.5602826949688,
436.462296651429));
#269395=CARTESIAN_POINT('Ctrl Pts',(124.84773085527,-100.946938853448,434.462296651429));
#269396=CARTESIAN_POINT('Ctrl Pts',(116.183399296896,-110.0907706828,432.462296651429));
#269397=CARTESIAN_POINT('Ctrl Pts',(107.519067738522,-119.234602512151,
430.462296651429));
#269398=CARTESIAN_POINT('Ctrl Pts',(97.5309980386227,-126.9104585261,428.462296651429));
#269399=CARTESIAN_POINT('Ctrl Pts',(87.5429283387236,-134.586314540048,
426.462296651429));
#269400=CARTESIAN_POINT('Ctrl Pts',(76.4770599218141,-140.605189688823,
424.462296651429));
#269401=CARTESIAN_POINT('Ctrl Pts',(65.4111915049046,-146.624064837598,
422.462296651429));
#269402=CARTESIAN_POINT('Ctrl Pts',(53.5400027769202,-150.837754439537,
420.462296651429));
#269403=CARTESIAN_POINT('Ctrl Pts',(41.6688140489359,-155.051444041475,
418.462296651429));
#269404=CARTESIAN_POINT('Ctrl Pts',(29.2846130745768,-157.356193074143,
416.462296651429));
#269405=CARTESIAN_POINT('Ctrl Pts',(16.9004121002176,-159.660942106811,
414.462296651429));
#269406=CARTESIAN_POINT('Ctrl Pts',(4.30813900827854,-160.,412.462296651429));
#269407=CARTESIAN_POINT('Ctrl Pts',(-8.28413408366049,-160.339057893189,
410.462296651429));
#269408=CARTESIAN_POINT('Ctrl Pts',(-20.7744157382971,-158.704075916301,
408.462296651429));
#269409=CARTESIAN_POINT('Ctrl Pts',(-33.2646973929338,-157.069093939413,
406.462296651429));
#269410=CARTESIAN_POINT('Ctrl Pts',(-45.345435423063,-153.500330774912,
404.462296651429));
#269411=CARTESIAN_POINT('Ctrl Pts',(-57.4261734531921,-149.931567610412,
402.462296651429));
#269412=CARTESIAN_POINT('Ctrl Pts',(-68.7998999948409,-144.516898051455,
400.462296651429));
#269413=CARTESIAN_POINT('Ctrl Pts',(-80.1736265364897,-139.102228492498,
398.462296651429));
#269414=CARTESIAN_POINT('Ctrl Pts',(-90.5602826949688,-131.974979673884,
396.462296651429));
#269415=CARTESIAN_POINT('Ctrl Pts',(-100.946938853448,-124.84773085527,
394.462296651429));
#269416=CARTESIAN_POINT('Ctrl Pts',(-110.0907706828,-116.183399296896,392.462296651429));
#269417=CARTESIAN_POINT('Ctrl Pts',(-119.234602512151,-107.519067738522,
390.462296651429));
#269418=CARTESIAN_POINT('Ctrl Pts',(-126.9104585261,-97.5309980386227,388.462296651429));
#269419=CARTESIAN_POINT('Ctrl Pts',(-134.586314540048,-87.5429283387236,
386.462296651429));
#269420=CARTESIAN_POINT('Ctrl Pts',(-140.605189688823,-76.4770599218141,
384.462296651429));
#269421=CARTESIAN_POINT('Ctrl Pts',(-146.624064837598,-65.4111915049046,
382.462296651429));
#269422=CARTESIAN_POINT('Ctrl Pts',(-150.837754439537,-53.5400027769203,
380.462296651429));
#269423=CARTESIAN_POINT('Ctrl Pts',(-155.051444041475,-41.668814048936,
378.462296651429));
#269424=CARTESIAN_POINT('Ctrl Pts',(-157.356193074143,-29.2846130745768,
376.462296651429));
#269425=CARTESIAN_POINT('Ctrl Pts',(-159.660942106811,-16.9004121002176,
374.462296651429));
#269426=CARTESIAN_POINT('Ctrl Pts',(-160.,-4.30813900827851,372.462296651429));
#269427=CARTESIAN_POINT('Ctrl Pts',(-160.,4.30813900827767,537.537703348572));
#269428=CARTESIAN_POINT('Ctrl Pts',(-159.660942106811,16.9004121002166,
535.537703348572));
#269429=CARTESIAN_POINT('Ctrl Pts',(-157.356193074143,29.2846130745759,
533.537703348572));
#269430=CARTESIAN_POINT('Ctrl Pts',(-155.051444041476,41.6688140489352,
531.537703348572));
#269431=CARTESIAN_POINT('Ctrl Pts',(-150.837754439537,53.5400027769194,
529.537703348572));
#269432=CARTESIAN_POINT('Ctrl Pts',(-146.624064837599,65.4111915049037,
527.537703348572));
#269433=CARTESIAN_POINT('Ctrl Pts',(-140.605189688823,76.4770599218133,
525.537703348572));
#269434=CARTESIAN_POINT('Ctrl Pts',(-134.586314540048,87.542928338723,523.537703348572));
#269435=CARTESIAN_POINT('Ctrl Pts',(-126.9104585261,97.530998038622,521.537703348572));
#269436=CARTESIAN_POINT('Ctrl Pts',(-119.234602512152,107.519067738521,
519.537703348572));
#269437=CARTESIAN_POINT('Ctrl Pts',(-110.0907706828,116.183399296895,517.537703348572));
#269438=CARTESIAN_POINT('Ctrl Pts',(-100.946938853448,124.847730855269,
515.537703348572));
#269439=CARTESIAN_POINT('Ctrl Pts',(-90.5602826949695,131.974979673883,
513.537703348572));
#269440=CARTESIAN_POINT('Ctrl Pts',(-80.1736265364906,139.102228492497,
511.537703348572));
#269441=CARTESIAN_POINT('Ctrl Pts',(-68.7998999948417,144.516898051454,
509.537703348572));
#269442=CARTESIAN_POINT('Ctrl Pts',(-57.4261734531929,149.931567610411,
507.537703348572));
#269443=CARTESIAN_POINT('Ctrl Pts',(-45.3454354230638,153.500330774912,
505.537703348572));
#269444=CARTESIAN_POINT('Ctrl Pts',(-33.2646973929347,157.069093939413,
503.537703348572));
#269445=CARTESIAN_POINT('Ctrl Pts',(-20.774415738298,158.704075916301,501.537703348572));
#269446=CARTESIAN_POINT('Ctrl Pts',(-8.28413408366129,160.339057893189,
499.537703348572));
#269447=CARTESIAN_POINT('Ctrl Pts',(4.30813900827766,160.,497.537703348572));
#269448=CARTESIAN_POINT('Ctrl Pts',(16.9004121002166,159.660942106811,495.537703348572));
#269449=CARTESIAN_POINT('Ctrl Pts',(29.2846130745759,157.356193074143,493.537703348572));
#269450=CARTESIAN_POINT('Ctrl Pts',(41.6688140489352,155.051444041476,491.537703348572));
#269451=CARTESIAN_POINT('Ctrl Pts',(53.5400027769194,150.837754439537,489.537703348572));
#269452=CARTESIAN_POINT('Ctrl Pts',(65.4111915049037,146.624064837599,487.537703348572));
#269453=CARTESIAN_POINT('Ctrl Pts',(76.4770599218133,140.605189688823,485.537703348572));
#269454=CARTESIAN_POINT('Ctrl Pts',(87.542928338723,134.586314540048,483.537703348572));
#269455=CARTESIAN_POINT('Ctrl Pts',(97.530998038622,126.9104585261,481.537703348572));
#269456=CARTESIAN_POINT('Ctrl Pts',(107.519067738521,119.234602512152,479.537703348572));
#269457=CARTESIAN_POINT('Ctrl Pts',(116.183399296895,110.0907706828,477.537703348572));
#269458=CARTESIAN_POINT('Ctrl Pts',(124.847730855269,100.946938853448,475.537703348572));
#269459=CARTESIAN_POINT('Ctrl Pts',(131.974979673883,90.5602826949695,473.537703348572));
#269460=CARTESIAN_POINT('Ctrl Pts',(139.102228492497,80.1736265364906,471.537703348572));
#269461=CARTESIAN_POINT('Ctrl Pts',(144.516898051454,68.7998999948417,469.537703348572));
#269462=CARTESIAN_POINT('Ctrl Pts',(149.931567610411,57.4261734531929,467.537703348572));
#269463=CARTESIAN_POINT('Ctrl Pts',(153.500330774912,45.3454354230638,465.537703348572));
#269464=CARTESIAN_POINT('Ctrl Pts',(157.069093939413,33.2646973929347,463.537703348572));
#269465=CARTESIAN_POINT('Ctrl Pts',(158.704075916301,20.774415738298,461.537703348572));
#269466=CARTESIAN_POINT('Ctrl Pts',(160.339057893189,8.28413408366131,459.537703348572));
#269467=CARTESIAN_POINT('Ctrl Pts',(160.,-4.30813900827765,457.537703348572));
#269468=CARTESIAN_POINT('Ctrl Pts',(159.660942106811,-16.9004121002166,
455.537703348572));
#269469=CARTESIAN_POINT('Ctrl Pts',(157.356193074143,-29.2846130745759,
453.537703348572));
#269470=CARTESIAN_POINT('Ctrl Pts',(155.051444041476,-41.6688140489352,
451.537703348572));
#269471=CARTESIAN_POINT('Ctrl Pts',(150.837754439537,-53.5400027769194,
449.537703348572));
#269472=CARTESIAN_POINT('Ctrl Pts',(146.624064837599,-65.4111915049036,
447.537703348572));
#269473=CARTESIAN_POINT('Ctrl Pts',(140.605189688823,-76.4770599218133,
445.537703348572));
#269474=CARTESIAN_POINT('Ctrl Pts',(134.586314540048,-87.5429283387229,
443.537703348572));
#269475=CARTESIAN_POINT('Ctrl Pts',(126.9104585261,-97.530998038622,441.537703348572));
#269476=CARTESIAN_POINT('Ctrl Pts',(119.234602512152,-107.519067738521,
439.537703348572));
#269477=CARTESIAN_POINT('Ctrl Pts',(110.0907706828,-116.183399296895,437.537703348572));
#269478=CARTESIAN_POINT('Ctrl Pts',(100.946938853448,-124.847730855269,
435.537703348572));
#269479=CARTESIAN_POINT('Ctrl Pts',(90.5602826949695,-131.974979673883,
433.537703348572));
#269480=CARTESIAN_POINT('Ctrl Pts',(80.1736265364905,-139.102228492497,
431.537703348572));
#269481=CARTESIAN_POINT('Ctrl Pts',(68.7998999948417,-144.516898051454,
429.537703348572));
#269482=CARTESIAN_POINT('Ctrl Pts',(57.426173453193,-149.931567610411,427.537703348572));
#269483=CARTESIAN_POINT('Ctrl Pts',(45.3454354230638,-153.500330774912,
425.537703348572));
#269484=CARTESIAN_POINT('Ctrl Pts',(33.2646973929347,-157.069093939413,
423.537703348572));
#269485=CARTESIAN_POINT('Ctrl Pts',(20.774415738298,-158.704075916301,421.537703348572));
#269486=CARTESIAN_POINT('Ctrl Pts',(8.28413408366139,-160.339057893189,
419.537703348572));
#269487=CARTESIAN_POINT('Ctrl Pts',(-4.30813900827764,-160.,417.537703348572));
#269488=CARTESIAN_POINT('Ctrl Pts',(-16.9004121002167,-159.660942106811,
415.537703348572));
#269489=CARTESIAN_POINT('Ctrl Pts',(-29.2846130745759,-157.356193074143,
413.537703348572));
#269490=CARTESIAN_POINT('Ctrl Pts',(-41.6688140489351,-155.051444041476,
411.537703348572));
#269491=CARTESIAN_POINT('Ctrl Pts',(-53.5400027769194,-150.837754439537,
409.537703348572));
#269492=CARTESIAN_POINT('Ctrl Pts',(-65.4111915049037,-146.624064837599,
407.537703348572));
#269493=CARTESIAN_POINT('Ctrl Pts',(-76.4770599218133,-140.605189688823,
405.537703348572));
#269494=CARTESIAN_POINT('Ctrl Pts',(-87.5429283387229,-134.586314540048,
403.537703348572));
#269495=CARTESIAN_POINT('Ctrl Pts',(-97.530998038622,-126.9104585261,401.537703348572));
#269496=CARTESIAN_POINT('Ctrl Pts',(-107.519067738521,-119.234602512152,
399.537703348572));
#269497=CARTESIAN_POINT('Ctrl Pts',(-116.183399296895,-110.0907706828,397.537703348572));
#269498=CARTESIAN_POINT('Ctrl Pts',(-124.847730855269,-100.946938853448,
395.537703348572));
#269499=CARTESIAN_POINT('Ctrl Pts',(-131.974979673883,-90.5602826949695,
393.537703348572));
#269500=CARTESIAN_POINT('Ctrl Pts',(-139.102228492497,-80.1736265364905,
391.537703348572));
#269501=CARTESIAN_POINT('Ctrl Pts',(-144.516898051454,-68.7998999948417,
389.537703348572));
#269502=CARTESIAN_POINT('Ctrl Pts',(-149.931567610411,-57.426173453193,
387.537703348572));
#269503=CARTESIAN_POINT('Ctrl Pts',(-153.500330774912,-45.3454354230638,
385.537703348572));
#269504=CARTESIAN_POINT('Ctrl Pts',(-157.069093939413,-33.2646973929347,
383.537703348572));
#269505=CARTESIAN_POINT('Ctrl Pts',(-158.704075916301,-20.774415738298,
381.537703348572));
#269506=CARTESIAN_POINT('Ctrl Pts',(-160.339057893189,-8.2841340836614,
379.537703348572));
#269507=CARTESIAN_POINT('Ctrl Pts',(-160.,4.30813900827767,377.537703348572));
#269508=CARTESIAN_POINT('Ctrl Pts',(-159.937609420477,6.2065412733309,530.789436448355));
#269509=CARTESIAN_POINT('Ctrl Pts',(-159.653854600275,13.5186762622033,
529.624118246284));
#269510=CARTESIAN_POINT('Ctrl Pts',(-158.704075916301,20.7744157382972,
528.462296651429));
#269511=CARTESIAN_POINT('Ctrl Pts',(-157.069093939413,33.2646973929339,
526.462296651429));
#269512=CARTESIAN_POINT('Ctrl Pts',(-153.500330774912,45.345435423063,524.462296651428));
#269513=CARTESIAN_POINT('Ctrl Pts',(-149.931567610412,57.4261734531921,
522.462296651429));
#269514=CARTESIAN_POINT('Ctrl Pts',(-144.516898051455,68.7998999948409,
520.462296651428));
#269515=CARTESIAN_POINT('Ctrl Pts',(-139.102228492498,80.1736265364898,
518.462296651428));
#269516=CARTESIAN_POINT('Ctrl Pts',(-131.974979673884,90.5602826949688,
516.462296651428));
#269517=CARTESIAN_POINT('Ctrl Pts',(-124.84773085527,100.946938853448,514.462296651429));
#269518=CARTESIAN_POINT('Ctrl Pts',(-116.183399296896,110.0907706828,512.462296651428));
#269519=CARTESIAN_POINT('Ctrl Pts',(-107.519067738522,119.234602512151,
510.462296651429));
#269520=CARTESIAN_POINT('Ctrl Pts',(-97.5309980386227,126.9104585261,508.462296651429));
#269521=CARTESIAN_POINT('Ctrl Pts',(-87.5429283387237,134.586314540048,
506.462296651429));
#269522=CARTESIAN_POINT('Ctrl Pts',(-76.4770599218141,140.605189688823,
504.462296651429));
#269523=CARTESIAN_POINT('Ctrl Pts',(-65.4111915049045,146.624064837598,
502.462296651429));
#269524=CARTESIAN_POINT('Ctrl Pts',(-53.5400027769202,150.837754439537,
500.462296651429));
#269525=CARTESIAN_POINT('Ctrl Pts',(-41.668814048936,155.051444041475,498.462296651429));
#269526=CARTESIAN_POINT('Ctrl Pts',(-29.2846130745767,157.356193074143,
496.462296651429));
#269527=CARTESIAN_POINT('Ctrl Pts',(-16.9004121002175,159.660942106811,
494.462296651429));
#269528=CARTESIAN_POINT('Ctrl Pts',(-4.30813900827852,160.,492.462296651428));
#269529=CARTESIAN_POINT('Ctrl Pts',(8.28413408366043,160.339057893189,490.462296651429));
#269530=CARTESIAN_POINT('Ctrl Pts',(20.7744157382972,158.704075916301,488.462296651429));
#269531=CARTESIAN_POINT('Ctrl Pts',(33.2646973929339,157.069093939413,486.462296651429));
#269532=CARTESIAN_POINT('Ctrl Pts',(45.345435423063,153.500330774912,484.462296651429));
#269533=CARTESIAN_POINT('Ctrl Pts',(57.4261734531921,149.931567610412,482.462296651429));
#269534=CARTESIAN_POINT('Ctrl Pts',(68.7998999948409,144.516898051455,480.462296651428));
#269535=CARTESIAN_POINT('Ctrl Pts',(80.1736265364898,139.102228492498,478.462296651429));
#269536=CARTESIAN_POINT('Ctrl Pts',(90.5602826949688,131.974979673884,476.462296651428));
#269537=CARTESIAN_POINT('Ctrl Pts',(100.946938853448,124.84773085527,474.462296651429));
#269538=CARTESIAN_POINT('Ctrl Pts',(110.0907706828,116.183399296896,472.462296651429));
#269539=CARTESIAN_POINT('Ctrl Pts',(119.234602512151,107.519067738522,470.462296651429));
#269540=CARTESIAN_POINT('Ctrl Pts',(126.9104585261,97.5309980386227,468.462296651429));
#269541=CARTESIAN_POINT('Ctrl Pts',(134.586314540048,87.5429283387237,466.462296651429));
#269542=CARTESIAN_POINT('Ctrl Pts',(140.605189688823,76.4770599218141,464.462296651429));
#269543=CARTESIAN_POINT('Ctrl Pts',(146.624064837598,65.4111915049045,462.462296651429));
#269544=CARTESIAN_POINT('Ctrl Pts',(150.837754439537,53.5400027769202,460.462296651429));
#269545=CARTESIAN_POINT('Ctrl Pts',(155.051444041475,41.668814048936,458.462296651429));
#269546=CARTESIAN_POINT('Ctrl Pts',(157.356193074143,29.2846130745767,456.462296651429));
#269547=CARTESIAN_POINT('Ctrl Pts',(159.660942106811,16.9004121002175,454.462296651429));
#269548=CARTESIAN_POINT('Ctrl Pts',(160.,4.30813900827853,452.462296651429));
#269549=CARTESIAN_POINT('Ctrl Pts',(160.339057893189,-8.28413408366043,
450.462296651429));
#269550=CARTESIAN_POINT('Ctrl Pts',(158.704075916301,-20.7744157382971,
448.462296651429));
#269551=CARTESIAN_POINT('Ctrl Pts',(157.069093939413,-33.2646973929339,
446.462296651429));
#269552=CARTESIAN_POINT('Ctrl Pts',(153.500330774912,-45.345435423063,444.462296651429));
#269553=CARTESIAN_POINT('Ctrl Pts',(149.931567610412,-57.4261734531921,
442.462296651429));
#269554=CARTESIAN_POINT('Ctrl Pts',(144.516898051455,-68.7998999948409,
440.462296651429));
#269555=CARTESIAN_POINT('Ctrl Pts',(139.102228492498,-80.1736265364898,
438.462296651429));
#269556=CARTESIAN_POINT('Ctrl Pts',(131.974979673884,-90.5602826949688,
436.462296651429));
#269557=CARTESIAN_POINT('Ctrl Pts',(124.84773085527,-100.946938853448,434.462296651429));
#269558=CARTESIAN_POINT('Ctrl Pts',(116.183399296896,-110.0907706828,432.462296651429));
#269559=CARTESIAN_POINT('Ctrl Pts',(107.519067738522,-119.234602512151,
430.462296651429));
#269560=CARTESIAN_POINT('Ctrl Pts',(97.5309980386227,-126.9104585261,428.462296651429));
#269561=CARTESIAN_POINT('Ctrl Pts',(87.5429283387236,-134.586314540048,
426.462296651429));
#269562=CARTESIAN_POINT('Ctrl Pts',(76.4770599218141,-140.605189688823,
424.462296651429));
#269563=CARTESIAN_POINT('Ctrl Pts',(65.4111915049045,-146.624064837598,
422.462296651429));
#269564=CARTESIAN_POINT('Ctrl Pts',(53.5400027769202,-150.837754439537,
420.462296651429));
#269565=CARTESIAN_POINT('Ctrl Pts',(41.6688140489359,-155.051444041475,
418.462296651429));
#269566=CARTESIAN_POINT('Ctrl Pts',(29.2846130745768,-157.356193074143,
416.462296651429));
#269567=CARTESIAN_POINT('Ctrl Pts',(16.9004121002176,-159.660942106811,
414.462296651429));
#269568=CARTESIAN_POINT('Ctrl Pts',(4.30813900827854,-160.,412.462296651429));
#269569=CARTESIAN_POINT('Ctrl Pts',(-8.28413408366049,-160.339057893189,
410.462296651429));
#269570=CARTESIAN_POINT('Ctrl Pts',(-20.7744157382971,-158.704075916301,
408.462296651429));
#269571=CARTESIAN_POINT('Ctrl Pts',(-33.2646973929338,-157.069093939413,
406.462296651429));
#269572=CARTESIAN_POINT('Ctrl Pts',(-45.345435423063,-153.500330774912,
404.462296651429));
#269573=CARTESIAN_POINT('Ctrl Pts',(-57.4261734531921,-149.931567610412,
402.462296651429));
#269574=CARTESIAN_POINT('Ctrl Pts',(-68.7998999948409,-144.516898051455,
400.462296651429));
#269575=CARTESIAN_POINT('Ctrl Pts',(-80.1736265364897,-139.102228492498,
398.462296651429));
#269576=CARTESIAN_POINT('Ctrl Pts',(-90.5602826949688,-131.974979673884,
396.462296651429));
#269577=CARTESIAN_POINT('Ctrl Pts',(-100.946938853448,-124.84773085527,
394.462296651429));
#269578=CARTESIAN_POINT('Ctrl Pts',(-110.0907706828,-116.183399296896,392.462296651429));
#269579=CARTESIAN_POINT('Ctrl Pts',(-119.234602512151,-107.519067738522,
390.462296651429));
#269580=CARTESIAN_POINT('Ctrl Pts',(-126.9104585261,-97.5309980386227,388.462296651429));
#269581=CARTESIAN_POINT('Ctrl Pts',(-134.586314540048,-87.5429283387237,
386.462296651429));
#269582=CARTESIAN_POINT('Ctrl Pts',(-140.605189688823,-76.4770599218141,
384.462296651429));
#269583=CARTESIAN_POINT('Ctrl Pts',(-146.624064837598,-65.4111915049046,
382.462296651429));
#269584=CARTESIAN_POINT('Ctrl Pts',(-150.837754439537,-53.5400027769203,
380.462296651429));
#269585=CARTESIAN_POINT('Ctrl Pts',(-155.051444041475,-41.668814048936,
378.462296651429));
#269586=CARTESIAN_POINT('Ctrl Pts',(-157.356193074143,-29.2846130745768,
376.462296651429));
#269587=CARTESIAN_POINT('Ctrl Pts',(-159.394142202012,-18.3340187941083,
374.693818523023));
#269588=CARTESIAN_POINT('Ctrl Pts',(-159.895664541343,-7.20669984090295,
372.923108716584));
#269589=CARTESIAN_POINT('Ctrl Pts',(-130.,-4.30813900827845,532.462296651428));
#269590=CARTESIAN_POINT('Ctrl Pts',(-130.339057893189,5.92308287892195,
530.462296651429));
#269591=CARTESIAN_POINT('Ctrl Pts',(-129.073425698447,16.0813817870903,
528.462296651428));
#269592=CARTESIAN_POINT('Ctrl Pts',(-127.807793503705,26.2396806952586,
526.462296651429));
#269593=CARTESIAN_POINT('Ctrl Pts',(-124.968635286058,36.0749255918146,
524.462296651428));
#269594=CARTESIAN_POINT('Ctrl Pts',(-122.129477068411,45.9101704883706,
522.462296651428));
#269595=CARTESIAN_POINT('Ctrl Pts',(-117.786702325804,55.1801850026546,
520.462296651428));
#269596=CARTESIAN_POINT('Ctrl Pts',(-113.443927583196,64.4501995169386,
518.462296651428));
#269597=CARTESIAN_POINT('Ctrl Pts',(-107.704469842635,72.9267251261946,
516.462296651428));
#269598=CARTESIAN_POINT('Ctrl Pts',(-101.965012102074,81.4032507354507,
514.462296651428));
#269599=CARTESIAN_POINT('Ctrl Pts',(-94.9701958612992,88.8775672472032,
512.462296651428));
#269600=CARTESIAN_POINT('Ctrl Pts',(-87.9753796205245,96.3518837589558,
510.462296651429));
#269601=CARTESIAN_POINT('Ctrl Pts',(-79.8974404698484,102.639948694851,
508.462296651428));
#269602=CARTESIAN_POINT('Ctrl Pts',(-71.8195013191724,108.928013630747,
506.462296651428));
#269603=CARTESIAN_POINT('Ctrl Pts',(-62.8573449296276,113.874993963172,
504.462296651428));
#269604=CARTESIAN_POINT('Ctrl Pts',(-53.8951885400828,118.821974295598,
502.462296651428));
#269605=CARTESIAN_POINT('Ctrl Pts',(-44.2694929456717,122.306058950682,
500.462296651428));
#269606=CARTESIAN_POINT('Ctrl Pts',(-34.6437973512606,125.790143605767,
498.462296651429));
#269607=CARTESIAN_POINT('Ctrl Pts',(-24.5915791233697,127.725542856289,
496.462296651428));
#269608=CARTESIAN_POINT('Ctrl Pts',(-14.5393608954789,129.660942106811,
494.462296651428));
#269609=CARTESIAN_POINT('Ctrl Pts',(-4.30813900827846,130.,492.462296651428));
#269610=CARTESIAN_POINT('Ctrl Pts',(5.92308287892194,130.339057893189,490.462296651429));
#269611=CARTESIAN_POINT('Ctrl Pts',(16.0813817870903,129.073425698447,488.462296651428));
#269612=CARTESIAN_POINT('Ctrl Pts',(26.2396806952586,127.807793503705,486.462296651428));
#269613=CARTESIAN_POINT('Ctrl Pts',(36.0749255918146,124.968635286058,484.462296651428));
#269614=CARTESIAN_POINT('Ctrl Pts',(45.9101704883706,122.129477068411,482.462296651428));
#269615=CARTESIAN_POINT('Ctrl Pts',(55.1801850026546,117.786702325804,480.462296651428));
#269616=CARTESIAN_POINT('Ctrl Pts',(64.4501995169386,113.443927583196,478.462296651429));
#269617=CARTESIAN_POINT('Ctrl Pts',(72.9267251261946,107.704469842635,476.462296651428));
#269618=CARTESIAN_POINT('Ctrl Pts',(81.4032507354506,101.965012102074,474.462296651428));
#269619=CARTESIAN_POINT('Ctrl Pts',(88.8775672472032,94.9701958612992,472.462296651428));
#269620=CARTESIAN_POINT('Ctrl Pts',(96.3518837589558,87.9753796205245,470.462296651428));
#269621=CARTESIAN_POINT('Ctrl Pts',(102.639948694851,79.8974404698484,468.462296651428));
#269622=CARTESIAN_POINT('Ctrl Pts',(108.928013630747,71.8195013191724,466.462296651428));
#269623=CARTESIAN_POINT('Ctrl Pts',(113.874993963172,62.8573449296276,464.462296651428));
#269624=CARTESIAN_POINT('Ctrl Pts',(118.821974295598,53.8951885400829,462.462296651428));
#269625=CARTESIAN_POINT('Ctrl Pts',(122.306058950682,44.2694929456717,460.462296651428));
#269626=CARTESIAN_POINT('Ctrl Pts',(125.790143605767,34.6437973512606,458.462296651429));
#269627=CARTESIAN_POINT('Ctrl Pts',(127.725542856289,24.5915791233698,456.462296651428));
#269628=CARTESIAN_POINT('Ctrl Pts',(129.660942106811,14.5393608954789,454.462296651429));
#269629=CARTESIAN_POINT('Ctrl Pts',(130.,4.30813900827846,452.462296651428));
#269630=CARTESIAN_POINT('Ctrl Pts',(130.339057893189,-5.92308287892194,
450.462296651428));
#269631=CARTESIAN_POINT('Ctrl Pts',(129.073425698447,-16.0813817870903,
448.462296651429));
#269632=CARTESIAN_POINT('Ctrl Pts',(127.807793503705,-26.2396806952586,
446.462296651429));
#269633=CARTESIAN_POINT('Ctrl Pts',(124.968635286058,-36.0749255918146,
444.462296651429));
#269634=CARTESIAN_POINT('Ctrl Pts',(122.129477068411,-45.9101704883706,
442.462296651429));
#269635=CARTESIAN_POINT('Ctrl Pts',(117.786702325804,-55.1801850026546,
440.462296651428));
#269636=CARTESIAN_POINT('Ctrl Pts',(113.443927583196,-64.4501995169386,
438.462296651429));
#269637=CARTESIAN_POINT('Ctrl Pts',(107.704469842635,-72.9267251261946,
436.462296651428));
#269638=CARTESIAN_POINT('Ctrl Pts',(101.965012102074,-81.4032507354506,
434.462296651429));
#269639=CARTESIAN_POINT('Ctrl Pts',(94.9701958612992,-88.8775672472032,
432.462296651428));
#269640=CARTESIAN_POINT('Ctrl Pts',(87.9753796205246,-96.3518837589557,
430.462296651429));
#269641=CARTESIAN_POINT('Ctrl Pts',(79.8974404698484,-102.639948694851,
428.462296651429));
#269642=CARTESIAN_POINT('Ctrl Pts',(71.8195013191723,-108.928013630747,
426.462296651428));
#269643=CARTESIAN_POINT('Ctrl Pts',(62.8573449296276,-113.874993963172,
424.462296651428));
#269644=CARTESIAN_POINT('Ctrl Pts',(53.8951885400829,-118.821974295598,
422.462296651428));
#269645=CARTESIAN_POINT('Ctrl Pts',(44.2694929456717,-122.306058950682,
420.462296651428));
#269646=CARTESIAN_POINT('Ctrl Pts',(34.6437973512606,-125.790143605767,
418.462296651429));
#269647=CARTESIAN_POINT('Ctrl Pts',(24.5915791233698,-127.725542856289,
416.462296651428));
#269648=CARTESIAN_POINT('Ctrl Pts',(14.5393608954789,-129.660942106811,
414.462296651429));
#269649=CARTESIAN_POINT('Ctrl Pts',(4.30813900827847,-130.,412.462296651428));
#269650=CARTESIAN_POINT('Ctrl Pts',(-5.92308287892199,-130.339057893189,
410.462296651428));
#269651=CARTESIAN_POINT('Ctrl Pts',(-16.0813817870903,-129.073425698447,
408.462296651428));
#269652=CARTESIAN_POINT('Ctrl Pts',(-26.2396806952585,-127.807793503705,
406.462296651429));
#269653=CARTESIAN_POINT('Ctrl Pts',(-36.0749255918146,-124.968635286058,
404.462296651428));
#269654=CARTESIAN_POINT('Ctrl Pts',(-45.9101704883706,-122.129477068411,
402.462296651429));
#269655=CARTESIAN_POINT('Ctrl Pts',(-55.1801850026546,-117.786702325804,
400.462296651428));
#269656=CARTESIAN_POINT('Ctrl Pts',(-64.4501995169385,-113.443927583197,
398.462296651429));
#269657=CARTESIAN_POINT('Ctrl Pts',(-72.9267251261946,-107.704469842635,
396.462296651428));
#269658=CARTESIAN_POINT('Ctrl Pts',(-81.4032507354507,-101.965012102074,
394.462296651429));
#269659=CARTESIAN_POINT('Ctrl Pts',(-88.8775672472032,-94.9701958612992,
392.462296651428));
#269660=CARTESIAN_POINT('Ctrl Pts',(-96.3518837589557,-87.9753796205246,
390.462296651428));
#269661=CARTESIAN_POINT('Ctrl Pts',(-102.639948694851,-79.8974404698484,
388.462296651428));
#269662=CARTESIAN_POINT('Ctrl Pts',(-108.928013630747,-71.8195013191723,
386.462296651428));
#269663=CARTESIAN_POINT('Ctrl Pts',(-113.874993963172,-62.8573449296276,
384.462296651428));
#269664=CARTESIAN_POINT('Ctrl Pts',(-118.821974295598,-53.8951885400829,
382.462296651429));
#269665=CARTESIAN_POINT('Ctrl Pts',(-122.306058950682,-44.2694929456718,
380.462296651428));
#269666=CARTESIAN_POINT('Ctrl Pts',(-125.790143605767,-34.6437973512606,
378.462296651429));
#269667=CARTESIAN_POINT('Ctrl Pts',(-127.725542856289,-24.5915791233698,
376.462296651428));
#269668=CARTESIAN_POINT('Ctrl Pts',(-129.660942106811,-14.5393608954789,
374.462296651428));
#269669=CARTESIAN_POINT('Ctrl Pts',(-130.,-4.30813900827845,372.462296651428));
#269670=CARTESIAN_POINT('Ctrl Pts',(-160.,-4.30813900827851,532.462296651429));
#269671=CARTESIAN_POINT('Ctrl Pts',(-160.339057893189,8.28413408366045,
530.462296651429));
#269672=CARTESIAN_POINT('Ctrl Pts',(-158.704075916301,20.7744157382972,
528.462296651429));
#269673=CARTESIAN_POINT('Ctrl Pts',(-157.069093939413,33.2646973929339,
526.462296651429));
#269674=CARTESIAN_POINT('Ctrl Pts',(-153.500330774912,45.345435423063,524.462296651428));
#269675=CARTESIAN_POINT('Ctrl Pts',(-149.931567610412,57.4261734531921,
522.462296651429));
#269676=CARTESIAN_POINT('Ctrl Pts',(-144.516898051455,68.7998999948409,
520.462296651428));
#269677=CARTESIAN_POINT('Ctrl Pts',(-139.102228492498,80.1736265364898,
518.462296651428));
#269678=CARTESIAN_POINT('Ctrl Pts',(-131.974979673884,90.5602826949688,
516.462296651428));
#269679=CARTESIAN_POINT('Ctrl Pts',(-124.84773085527,100.946938853448,514.462296651429));
#269680=CARTESIAN_POINT('Ctrl Pts',(-116.183399296896,110.0907706828,512.462296651428));
#269681=CARTESIAN_POINT('Ctrl Pts',(-107.519067738522,119.234602512151,
510.462296651429));
#269682=CARTESIAN_POINT('Ctrl Pts',(-97.5309980386227,126.9104585261,508.462296651429));
#269683=CARTESIAN_POINT('Ctrl Pts',(-87.5429283387237,134.586314540048,
506.462296651428));
#269684=CARTESIAN_POINT('Ctrl Pts',(-76.4770599218141,140.605189688823,
504.462296651429));
#269685=CARTESIAN_POINT('Ctrl Pts',(-65.4111915049045,146.624064837598,
502.462296651429));
#269686=CARTESIAN_POINT('Ctrl Pts',(-53.5400027769202,150.837754439537,
500.462296651429));
#269687=CARTESIAN_POINT('Ctrl Pts',(-41.668814048936,155.051444041475,498.462296651429));
#269688=CARTESIAN_POINT('Ctrl Pts',(-29.2846130745767,157.356193074143,
496.462296651429));
#269689=CARTESIAN_POINT('Ctrl Pts',(-16.9004121002175,159.660942106811,
494.462296651429));
#269690=CARTESIAN_POINT('Ctrl Pts',(-4.30813900827852,160.,492.462296651428));
#269691=CARTESIAN_POINT('Ctrl Pts',(8.28413408366043,160.339057893189,490.462296651429));
#269692=CARTESIAN_POINT('Ctrl Pts',(20.7744157382972,158.704075916301,488.462296651429));
#269693=CARTESIAN_POINT('Ctrl Pts',(33.2646973929339,157.069093939413,486.462296651429));
#269694=CARTESIAN_POINT('Ctrl Pts',(45.345435423063,153.500330774912,484.462296651429));
#269695=CARTESIAN_POINT('Ctrl Pts',(57.4261734531921,149.931567610412,482.462296651429));
#269696=CARTESIAN_POINT('Ctrl Pts',(68.7998999948409,144.516898051455,480.462296651428));
#269697=CARTESIAN_POINT('Ctrl Pts',(80.1736265364898,139.102228492498,478.462296651429));
#269698=CARTESIAN_POINT('Ctrl Pts',(90.5602826949688,131.974979673884,476.462296651428));
#269699=CARTESIAN_POINT('Ctrl Pts',(100.946938853448,124.84773085527,474.462296651429));
#269700=CARTESIAN_POINT('Ctrl Pts',(110.0907706828,116.183399296896,472.462296651429));
#269701=CARTESIAN_POINT('Ctrl Pts',(119.234602512151,107.519067738522,470.462296651429));
#269702=CARTESIAN_POINT('Ctrl Pts',(126.9104585261,97.5309980386227,468.462296651429));
#269703=CARTESIAN_POINT('Ctrl Pts',(134.586314540048,87.5429283387237,466.462296651429));
#269704=CARTESIAN_POINT('Ctrl Pts',(140.605189688823,76.4770599218141,464.462296651429));
#269705=CARTESIAN_POINT('Ctrl Pts',(146.624064837598,65.4111915049045,462.462296651429));
#269706=CARTESIAN_POINT('Ctrl Pts',(150.837754439537,53.5400027769202,460.462296651429));
#269707=CARTESIAN_POINT('Ctrl Pts',(155.051444041475,41.668814048936,458.462296651429));
#269708=CARTESIAN_POINT('Ctrl Pts',(157.356193074143,29.2846130745767,456.462296651429));
#269709=CARTESIAN_POINT('Ctrl Pts',(159.660942106811,16.9004121002175,454.462296651429));
#269710=CARTESIAN_POINT('Ctrl Pts',(160.,4.30813900827853,452.462296651429));
#269711=CARTESIAN_POINT('Ctrl Pts',(160.339057893189,-8.28413408366043,
450.462296651429));
#269712=CARTESIAN_POINT('Ctrl Pts',(158.704075916301,-20.7744157382971,
448.462296651429));
#269713=CARTESIAN_POINT('Ctrl Pts',(157.069093939413,-33.2646973929339,
446.462296651429));
#269714=CARTESIAN_POINT('Ctrl Pts',(153.500330774912,-45.345435423063,444.462296651429));
#269715=CARTESIAN_POINT('Ctrl Pts',(149.931567610412,-57.4261734531921,
442.462296651429));
#269716=CARTESIAN_POINT('Ctrl Pts',(144.516898051455,-68.7998999948409,
440.462296651429));
#269717=CARTESIAN_POINT('Ctrl Pts',(139.102228492498,-80.1736265364898,
438.462296651429));
#269718=CARTESIAN_POINT('Ctrl Pts',(131.974979673884,-90.5602826949688,
436.462296651429));
#269719=CARTESIAN_POINT('Ctrl Pts',(124.84773085527,-100.946938853448,434.462296651429));
#269720=CARTESIAN_POINT('Ctrl Pts',(116.183399296896,-110.0907706828,432.462296651429));
#269721=CARTESIAN_POINT('Ctrl Pts',(107.519067738522,-119.234602512151,
430.462296651429));
#269722=CARTESIAN_POINT('Ctrl Pts',(97.5309980386227,-126.9104585261,428.462296651429));
#269723=CARTESIAN_POINT('Ctrl Pts',(87.5429283387236,-134.586314540048,
426.462296651429));
#269724=CARTESIAN_POINT('Ctrl Pts',(76.4770599218141,-140.605189688823,
424.462296651429));
#269725=CARTESIAN_POINT('Ctrl Pts',(65.4111915049046,-146.624064837598,
422.462296651429));
#269726=CARTESIAN_POINT('Ctrl Pts',(53.5400027769202,-150.837754439537,
420.462296651429));
#269727=CARTESIAN_POINT('Ctrl Pts',(41.6688140489359,-155.051444041475,
418.462296651429));
#269728=CARTESIAN_POINT('Ctrl Pts',(29.2846130745768,-157.356193074143,
416.462296651429));
#269729=CARTESIAN_POINT('Ctrl Pts',(16.9004121002176,-159.660942106811,
414.462296651429));
#269730=CARTESIAN_POINT('Ctrl Pts',(4.30813900827854,-160.,412.462296651429));
#269731=CARTESIAN_POINT('Ctrl Pts',(-8.28413408366049,-160.339057893189,
410.462296651429));
#269732=CARTESIAN_POINT('Ctrl Pts',(-20.7744157382971,-158.704075916301,
408.462296651429));
#269733=CARTESIAN_POINT('Ctrl Pts',(-33.2646973929338,-157.069093939413,
406.462296651429));
#269734=CARTESIAN_POINT('Ctrl Pts',(-45.345435423063,-153.500330774912,
404.462296651429));
#269735=CARTESIAN_POINT('Ctrl Pts',(-57.4261734531921,-149.931567610412,
402.462296651429));
#269736=CARTESIAN_POINT('Ctrl Pts',(-68.7998999948409,-144.516898051455,
400.462296651429));
#269737=CARTESIAN_POINT('Ctrl Pts',(-80.1736265364897,-139.102228492498,
398.462296651429));
#269738=CARTESIAN_POINT('Ctrl Pts',(-90.5602826949688,-131.974979673884,
396.462296651429));
#269739=CARTESIAN_POINT('Ctrl Pts',(-100.946938853448,-124.84773085527,
394.462296651429));
#269740=CARTESIAN_POINT('Ctrl Pts',(-110.0907706828,-116.183399296896,392.462296651429));
#269741=CARTESIAN_POINT('Ctrl Pts',(-119.234602512151,-107.519067738522,
390.462296651429));
#269742=CARTESIAN_POINT('Ctrl Pts',(-126.9104585261,-97.5309980386227,388.462296651429));
#269743=CARTESIAN_POINT('Ctrl Pts',(-134.586314540048,-87.5429283387236,
386.462296651429));
#269744=CARTESIAN_POINT('Ctrl Pts',(-140.605189688823,-76.4770599218141,
384.462296651429));
#269745=CARTESIAN_POINT('Ctrl Pts',(-146.624064837598,-65.4111915049046,
382.462296651429));
#269746=CARTESIAN_POINT('Ctrl Pts',(-150.837754439537,-53.5400027769203,
380.462296651429));
#269747=CARTESIAN_POINT('Ctrl Pts',(-155.051444041475,-41.668814048936,
378.462296651429));
#269748=CARTESIAN_POINT('Ctrl Pts',(-157.356193074143,-29.2846130745768,
376.462296651429));
#269749=CARTESIAN_POINT('Ctrl Pts',(-159.660942106811,-16.9004121002176,
374.462296651429));
#269750=CARTESIAN_POINT('Ctrl Pts',(-160.,-4.30813900827851,372.462296651429));
#269751=CARTESIAN_POINT('Ctrl Pts',(160.,4.30813900827813,692.462296651428));
#269752=CARTESIAN_POINT('Ctrl Pts',(160.339057893189,-8.28413408366083,
690.462296651428));
#269753=CARTESIAN_POINT('Ctrl Pts',(158.704075916301,-20.7744157382975,
688.462296651428));
#269754=CARTESIAN_POINT('Ctrl Pts',(157.069093939413,-33.2646973929343,
686.462296651429));
#269755=CARTESIAN_POINT('Ctrl Pts',(153.500330774912,-45.3454354230633,
684.462296651428));
#269756=CARTESIAN_POINT('Ctrl Pts',(149.931567610412,-57.4261734531924,
682.462296651428));
#269757=CARTESIAN_POINT('Ctrl Pts',(144.516898051455,-68.7998999948413,
680.462296651428));
#269758=CARTESIAN_POINT('Ctrl Pts',(139.102228492497,-80.1736265364901,
678.462296651428));
#269759=CARTESIAN_POINT('Ctrl Pts',(131.974979673883,-90.5602826949691,
676.462296651428));
#269760=CARTESIAN_POINT('Ctrl Pts',(124.847730855269,-100.946938853448,
674.462296651428));
#269761=CARTESIAN_POINT('Ctrl Pts',(116.183399296895,-110.0907706828,672.462296651428));
#269762=CARTESIAN_POINT('Ctrl Pts',(107.519067738521,-119.234602512152,
670.462296651428));
#269763=CARTESIAN_POINT('Ctrl Pts',(97.5309980386224,-126.9104585261,668.462296651428));
#269764=CARTESIAN_POINT('Ctrl Pts',(87.5429283387234,-134.586314540048,
666.462296651428));
#269765=CARTESIAN_POINT('Ctrl Pts',(76.4770599218137,-140.605189688823,
664.462296651428));
#269766=CARTESIAN_POINT('Ctrl Pts',(65.4111915049041,-146.624064837599,
662.462296651428));
#269767=CARTESIAN_POINT('Ctrl Pts',(53.5400027769198,-150.837754439537,
660.462296651428));
#269768=CARTESIAN_POINT('Ctrl Pts',(41.6688140489356,-155.051444041475,
658.462296651428));
#269769=CARTESIAN_POINT('Ctrl Pts',(29.2846130745764,-157.356193074143,
656.462296651428));
#269770=CARTESIAN_POINT('Ctrl Pts',(16.9004121002171,-159.660942106811,
654.462296651428));
#269771=CARTESIAN_POINT('Ctrl Pts',(4.30813900827814,-160.,652.462296651428));
#269772=CARTESIAN_POINT('Ctrl Pts',(-8.28413408366082,-160.339057893189,
650.462296651428));
#269773=CARTESIAN_POINT('Ctrl Pts',(-20.7744157382975,-158.704075916301,
648.462296651428));
#269774=CARTESIAN_POINT('Ctrl Pts',(-33.2646973929342,-157.069093939413,
646.462296651428));
#269775=CARTESIAN_POINT('Ctrl Pts',(-45.3454354230633,-153.500330774912,
644.462296651428));
#269776=CARTESIAN_POINT('Ctrl Pts',(-57.4261734531924,-149.931567610412,
642.462296651428));
#269777=CARTESIAN_POINT('Ctrl Pts',(-68.7998999948413,-144.516898051455,
640.462296651428));
#269778=CARTESIAN_POINT('Ctrl Pts',(-80.1736265364901,-139.102228492497,
638.462296651428));
#269779=CARTESIAN_POINT('Ctrl Pts',(-90.5602826949691,-131.974979673883,
636.462296651428));
#269780=CARTESIAN_POINT('Ctrl Pts',(-100.946938853448,-124.847730855269,
634.462296651428));
#269781=CARTESIAN_POINT('Ctrl Pts',(-110.0907706828,-116.183399296895,632.462296651428));
#269782=CARTESIAN_POINT('Ctrl Pts',(-119.234602512152,-107.519067738521,
630.462296651428));
#269783=CARTESIAN_POINT('Ctrl Pts',(-126.9104585261,-97.5309980386224,628.462296651428));
#269784=CARTESIAN_POINT('Ctrl Pts',(-134.586314540048,-87.5429283387234,
626.462296651429));
#269785=CARTESIAN_POINT('Ctrl Pts',(-140.605189688823,-76.4770599218137,
624.462296651428));
#269786=CARTESIAN_POINT('Ctrl Pts',(-146.624064837599,-65.4111915049041,
622.462296651428));
#269787=CARTESIAN_POINT('Ctrl Pts',(-150.837754439537,-53.5400027769199,
620.462296651428));
#269788=CARTESIAN_POINT('Ctrl Pts',(-155.051444041475,-41.6688140489356,
618.462296651428));
#269789=CARTESIAN_POINT('Ctrl Pts',(-157.356193074143,-29.2846130745764,
616.462296651428));
#269790=CARTESIAN_POINT('Ctrl Pts',(-159.660942106811,-16.9004121002171,
614.462296651429));
#269791=CARTESIAN_POINT('Ctrl Pts',(-160.,-4.30813900827815,612.462296651428));
#269792=CARTESIAN_POINT('Ctrl Pts',(-160.339057893189,8.28413408366081,
610.462296651428));
#269793=CARTESIAN_POINT('Ctrl Pts',(-158.704075916301,20.7744157382975,
608.462296651428));
#269794=CARTESIAN_POINT('Ctrl Pts',(-157.069093939413,33.2646973929342,
606.462296651428));
#269795=CARTESIAN_POINT('Ctrl Pts',(-153.500330774912,45.3454354230633,
604.462296651428));
#269796=CARTESIAN_POINT('Ctrl Pts',(-149.931567610412,57.4261734531924,
602.462296651429));
#269797=CARTESIAN_POINT('Ctrl Pts',(-144.516898051455,68.7998999948413,
600.462296651428));
#269798=CARTESIAN_POINT('Ctrl Pts',(-139.102228492497,80.1736265364901,
598.462296651428));
#269799=CARTESIAN_POINT('Ctrl Pts',(-131.974979673883,90.5602826949691,
596.462296651428));
#269800=CARTESIAN_POINT('Ctrl Pts',(-124.847730855269,100.946938853448,
594.462296651428));
#269801=CARTESIAN_POINT('Ctrl Pts',(-116.183399296895,110.0907706828,592.462296651428));
#269802=CARTESIAN_POINT('Ctrl Pts',(-107.519067738521,119.234602512152,
590.462296651428));
#269803=CARTESIAN_POINT('Ctrl Pts',(-97.5309980386224,126.9104585261,588.462296651428));
#269804=CARTESIAN_POINT('Ctrl Pts',(-87.5429283387233,134.586314540048,
586.462296651428));
#269805=CARTESIAN_POINT('Ctrl Pts',(-76.4770599218137,140.605189688823,
584.462296651428));
#269806=CARTESIAN_POINT('Ctrl Pts',(-65.4111915049042,146.624064837599,
582.462296651428));
#269807=CARTESIAN_POINT('Ctrl Pts',(-53.5400027769199,150.837754439537,
580.462296651428));
#269808=CARTESIAN_POINT('Ctrl Pts',(-41.6688140489356,155.051444041475,
578.462296651428));
#269809=CARTESIAN_POINT('Ctrl Pts',(-29.2846130745764,157.356193074143,
576.462296651428));
#269810=CARTESIAN_POINT('Ctrl Pts',(-16.9004121002172,159.660942106811,
574.462296651428));
#269811=CARTESIAN_POINT('Ctrl Pts',(-4.30813900827816,160.,572.462296651428));
#269812=CARTESIAN_POINT('Ctrl Pts',(8.28413408366087,160.339057893189,570.462296651428));
#269813=CARTESIAN_POINT('Ctrl Pts',(20.7744157382975,158.704075916301,568.462296651428));
#269814=CARTESIAN_POINT('Ctrl Pts',(33.2646973929342,157.069093939413,566.462296651428));
#269815=CARTESIAN_POINT('Ctrl Pts',(45.3454354230633,153.500330774912,564.462296651428));
#269816=CARTESIAN_POINT('Ctrl Pts',(57.4261734531925,149.931567610412,562.462296651428));
#269817=CARTESIAN_POINT('Ctrl Pts',(68.7998999948413,144.516898051455,560.462296651428));
#269818=CARTESIAN_POINT('Ctrl Pts',(80.1736265364901,139.102228492498,558.462296651428));
#269819=CARTESIAN_POINT('Ctrl Pts',(90.560282694969,131.974979673883,556.462296651428));
#269820=CARTESIAN_POINT('Ctrl Pts',(100.946938853448,124.847730855269,554.462296651428));
#269821=CARTESIAN_POINT('Ctrl Pts',(110.0907706828,116.183399296895,552.462296651428));
#269822=CARTESIAN_POINT('Ctrl Pts',(119.234602512152,107.519067738521,550.462296651428));
#269823=CARTESIAN_POINT('Ctrl Pts',(126.9104585261,97.5309980386224,548.462296651428));
#269824=CARTESIAN_POINT('Ctrl Pts',(134.586314540048,87.5429283387233,546.462296651428));
#269825=CARTESIAN_POINT('Ctrl Pts',(140.605189688823,76.4770599218137,544.462296651428));
#269826=CARTESIAN_POINT('Ctrl Pts',(146.624064837599,65.4111915049042,542.462296651428));
#269827=CARTESIAN_POINT('Ctrl Pts',(150.837754439537,53.5400027769199,540.462296651428));
#269828=CARTESIAN_POINT('Ctrl Pts',(155.051444041475,41.6688140489356,538.462296651428));
#269829=CARTESIAN_POINT('Ctrl Pts',(157.356193074143,29.2846130745764,536.462296651428));
#269830=CARTESIAN_POINT('Ctrl Pts',(159.660942106811,16.9004121002172,534.462296651428));
#269831=CARTESIAN_POINT('Ctrl Pts',(160.,4.30813900827813,532.462296651428));
#269832=CARTESIAN_POINT('Ctrl Pts',(160.,-4.30813900827805,697.537703348572));
#269833=CARTESIAN_POINT('Ctrl Pts',(159.660942106811,-16.900412100217,695.537703348572));
#269834=CARTESIAN_POINT('Ctrl Pts',(157.356193074143,-29.2846130745763,
693.537703348572));
#269835=CARTESIAN_POINT('Ctrl Pts',(155.051444041475,-41.6688140489355,
691.537703348572));
#269836=CARTESIAN_POINT('Ctrl Pts',(150.837754439537,-53.5400027769198,
689.537703348572));
#269837=CARTESIAN_POINT('Ctrl Pts',(146.624064837599,-65.411191504904,687.537703348572));
#269838=CARTESIAN_POINT('Ctrl Pts',(140.605189688823,-76.4770599218136,
685.537703348572));
#269839=CARTESIAN_POINT('Ctrl Pts',(134.586314540048,-87.5429283387233,
683.537703348572));
#269840=CARTESIAN_POINT('Ctrl Pts',(126.9104585261,-97.5309980386223,681.537703348572));
#269841=CARTESIAN_POINT('Ctrl Pts',(119.234602512152,-107.519067738521,
679.537703348572));
#269842=CARTESIAN_POINT('Ctrl Pts',(110.0907706828,-116.183399296895,677.537703348572));
#269843=CARTESIAN_POINT('Ctrl Pts',(100.946938853448,-124.847730855269,
675.537703348572));
#269844=CARTESIAN_POINT('Ctrl Pts',(90.5602826949691,-131.974979673883,
673.537703348572));
#269845=CARTESIAN_POINT('Ctrl Pts',(80.1736265364902,-139.102228492497,
671.537703348572));
#269846=CARTESIAN_POINT('Ctrl Pts',(68.7998999948414,-144.516898051454,
669.537703348572));
#269847=CARTESIAN_POINT('Ctrl Pts',(57.4261734531925,-149.931567610412,
667.537703348572));
#269848=CARTESIAN_POINT('Ctrl Pts',(45.3454354230634,-153.500330774912,
665.537703348572));
#269849=CARTESIAN_POINT('Ctrl Pts',(33.2646973929343,-157.069093939413,
663.537703348572));
#269850=CARTESIAN_POINT('Ctrl Pts',(20.7744157382976,-158.704075916301,
661.537703348572));
#269851=CARTESIAN_POINT('Ctrl Pts',(8.28413408366091,-160.339057893189,
659.537703348572));
#269852=CARTESIAN_POINT('Ctrl Pts',(-4.30813900827804,-160.,657.537703348572));
#269853=CARTESIAN_POINT('Ctrl Pts',(-16.900412100217,-159.660942106811,
655.537703348572));
#269854=CARTESIAN_POINT('Ctrl Pts',(-29.2846130745763,-157.356193074143,
653.537703348572));
#269855=CARTESIAN_POINT('Ctrl Pts',(-41.6688140489355,-155.051444041475,
651.537703348572));
#269856=CARTESIAN_POINT('Ctrl Pts',(-53.5400027769198,-150.837754439537,
649.537703348572));
#269857=CARTESIAN_POINT('Ctrl Pts',(-65.411191504904,-146.624064837599,
647.537703348572));
#269858=CARTESIAN_POINT('Ctrl Pts',(-76.4770599218136,-140.605189688823,
645.537703348572));
#269859=CARTESIAN_POINT('Ctrl Pts',(-87.5429283387233,-134.586314540048,
643.537703348572));
#269860=CARTESIAN_POINT('Ctrl Pts',(-97.5309980386223,-126.9104585261,641.537703348572));
#269861=CARTESIAN_POINT('Ctrl Pts',(-107.519067738521,-119.234602512152,
639.537703348572));
#269862=CARTESIAN_POINT('Ctrl Pts',(-116.183399296895,-110.0907706828,637.537703348572));
#269863=CARTESIAN_POINT('Ctrl Pts',(-124.847730855269,-100.946938853448,
635.537703348572));
#269864=CARTESIAN_POINT('Ctrl Pts',(-131.974979673883,-90.5602826949692,
633.537703348572));
#269865=CARTESIAN_POINT('Ctrl Pts',(-139.102228492497,-80.1736265364902,
631.537703348572));
#269866=CARTESIAN_POINT('Ctrl Pts',(-144.516898051454,-68.7998999948414,
629.537703348572));
#269867=CARTESIAN_POINT('Ctrl Pts',(-149.931567610412,-57.4261734531925,
627.537703348572));
#269868=CARTESIAN_POINT('Ctrl Pts',(-153.500330774912,-45.3454354230634,
625.537703348572));
#269869=CARTESIAN_POINT('Ctrl Pts',(-157.069093939413,-33.2646973929344,
623.537703348572));
#269870=CARTESIAN_POINT('Ctrl Pts',(-158.704075916301,-20.7744157382976,
621.537703348572));
#269871=CARTESIAN_POINT('Ctrl Pts',(-160.339057893189,-8.28413408366092,
619.537703348572));
#269872=CARTESIAN_POINT('Ctrl Pts',(-160.,4.30813900827803,617.537703348572));
#269873=CARTESIAN_POINT('Ctrl Pts',(-159.660942106811,16.900412100217,615.537703348572));
#269874=CARTESIAN_POINT('Ctrl Pts',(-157.356193074143,29.2846130745763,
613.537703348572));
#269875=CARTESIAN_POINT('Ctrl Pts',(-155.051444041475,41.6688140489355,
611.537703348572));
#269876=CARTESIAN_POINT('Ctrl Pts',(-150.837754439537,53.5400027769198,
609.537703348572));
#269877=CARTESIAN_POINT('Ctrl Pts',(-146.624064837599,65.411191504904,607.537703348572));
#269878=CARTESIAN_POINT('Ctrl Pts',(-140.605189688823,76.4770599218136,
605.537703348572));
#269879=CARTESIAN_POINT('Ctrl Pts',(-134.586314540048,87.5429283387233,
603.537703348572));
#269880=CARTESIAN_POINT('Ctrl Pts',(-126.9104585261,97.5309980386223,601.537703348572));
#269881=CARTESIAN_POINT('Ctrl Pts',(-119.234602512152,107.519067738521,
599.537703348572));
#269882=CARTESIAN_POINT('Ctrl Pts',(-110.0907706828,116.183399296895,597.537703348572));
#269883=CARTESIAN_POINT('Ctrl Pts',(-100.946938853448,124.847730855269,
595.537703348572));
#269884=CARTESIAN_POINT('Ctrl Pts',(-90.5602826949692,131.974979673883,
593.537703348572));
#269885=CARTESIAN_POINT('Ctrl Pts',(-80.1736265364901,139.102228492497,
591.537703348572));
#269886=CARTESIAN_POINT('Ctrl Pts',(-68.7998999948414,144.516898051454,
589.537703348572));
#269887=CARTESIAN_POINT('Ctrl Pts',(-57.4261734531926,149.931567610412,
587.537703348572));
#269888=CARTESIAN_POINT('Ctrl Pts',(-45.3454354230634,153.500330774912,
585.537703348572));
#269889=CARTESIAN_POINT('Ctrl Pts',(-33.2646973929343,157.069093939413,
583.537703348572));
#269890=CARTESIAN_POINT('Ctrl Pts',(-20.7744157382976,158.704075916301,
581.537703348572));
#269891=CARTESIAN_POINT('Ctrl Pts',(-8.284134083661,160.339057893189,579.537703348572));
#269892=CARTESIAN_POINT('Ctrl Pts',(4.30813900827803,160.,577.537703348572));
#269893=CARTESIAN_POINT('Ctrl Pts',(16.9004121002171,159.660942106811,575.537703348572));
#269894=CARTESIAN_POINT('Ctrl Pts',(29.2846130745762,157.356193074143,573.537703348572));
#269895=CARTESIAN_POINT('Ctrl Pts',(41.6688140489354,155.051444041476,571.537703348572));
#269896=CARTESIAN_POINT('Ctrl Pts',(53.5400027769198,150.837754439537,569.537703348572));
#269897=CARTESIAN_POINT('Ctrl Pts',(65.4111915049041,146.624064837599,567.537703348572));
#269898=CARTESIAN_POINT('Ctrl Pts',(76.4770599218136,140.605189688823,565.537703348572));
#269899=CARTESIAN_POINT('Ctrl Pts',(87.5429283387232,134.586314540048,563.537703348572));
#269900=CARTESIAN_POINT('Ctrl Pts',(97.5309980386223,126.9104585261,561.537703348572));
#269901=CARTESIAN_POINT('Ctrl Pts',(107.519067738521,119.234602512152,559.537703348572));
#269902=CARTESIAN_POINT('Ctrl Pts',(116.183399296895,110.0907706828,557.537703348572));
#269903=CARTESIAN_POINT('Ctrl Pts',(124.847730855269,100.946938853448,555.537703348572));
#269904=CARTESIAN_POINT('Ctrl Pts',(131.974979673883,90.5602826949692,553.537703348572));
#269905=CARTESIAN_POINT('Ctrl Pts',(139.102228492497,80.1736265364902,551.537703348572));
#269906=CARTESIAN_POINT('Ctrl Pts',(144.516898051454,68.7998999948414,549.537703348572));
#269907=CARTESIAN_POINT('Ctrl Pts',(149.931567610412,57.4261734531926,547.537703348572));
#269908=CARTESIAN_POINT('Ctrl Pts',(153.500330774912,45.3454354230634,545.537703348572));
#269909=CARTESIAN_POINT('Ctrl Pts',(157.069093939413,33.2646973929343,543.537703348572));
#269910=CARTESIAN_POINT('Ctrl Pts',(158.704075916301,20.7744157382976,541.537703348572));
#269911=CARTESIAN_POINT('Ctrl Pts',(160.339057893189,8.28413408366101,539.537703348572));
#269912=CARTESIAN_POINT('Ctrl Pts',(160.,-4.30813900827805,537.537703348572));
#269913=CARTESIAN_POINT('Ctrl Pts',(159.937609420477,-6.20654127333164,
690.789436448355));
#269914=CARTESIAN_POINT('Ctrl Pts',(159.653854600275,-13.5186762622038,
689.624118246284));
#269915=CARTESIAN_POINT('Ctrl Pts',(158.704075916301,-20.7744157382975,
688.462296651428));
#269916=CARTESIAN_POINT('Ctrl Pts',(157.069093939413,-33.2646973929343,
686.462296651429));
#269917=CARTESIAN_POINT('Ctrl Pts',(153.500330774912,-45.3454354230633,
684.462296651428));
#269918=CARTESIAN_POINT('Ctrl Pts',(149.931567610412,-57.4261734531925,
682.462296651428));
#269919=CARTESIAN_POINT('Ctrl Pts',(144.516898051455,-68.7998999948413,
680.462296651428));
#269920=CARTESIAN_POINT('Ctrl Pts',(139.102228492497,-80.1736265364901,
678.462296651428));
#269921=CARTESIAN_POINT('Ctrl Pts',(131.974979673883,-90.5602826949691,
676.462296651428));
#269922=CARTESIAN_POINT('Ctrl Pts',(124.847730855269,-100.946938853448,
674.462296651428));
#269923=CARTESIAN_POINT('Ctrl Pts',(116.183399296895,-110.0907706828,672.462296651428));
#269924=CARTESIAN_POINT('Ctrl Pts',(107.519067738521,-119.234602512152,
670.462296651428));
#269925=CARTESIAN_POINT('Ctrl Pts',(97.5309980386224,-126.9104585261,668.462296651428));
#269926=CARTESIAN_POINT('Ctrl Pts',(87.5429283387234,-134.586314540048,
666.462296651428));
#269927=CARTESIAN_POINT('Ctrl Pts',(76.4770599218137,-140.605189688823,
664.462296651428));
#269928=CARTESIAN_POINT('Ctrl Pts',(65.4111915049041,-146.624064837599,
662.462296651428));
#269929=CARTESIAN_POINT('Ctrl Pts',(53.5400027769198,-150.837754439537,
660.462296651428));
#269930=CARTESIAN_POINT('Ctrl Pts',(41.6688140489356,-155.051444041475,
658.462296651428));
#269931=CARTESIAN_POINT('Ctrl Pts',(29.2846130745764,-157.356193074143,
656.462296651428));
#269932=CARTESIAN_POINT('Ctrl Pts',(16.9004121002171,-159.660942106811,
654.462296651428));
#269933=CARTESIAN_POINT('Ctrl Pts',(4.30813900827814,-160.,652.462296651428));
#269934=CARTESIAN_POINT('Ctrl Pts',(-8.28413408366082,-160.339057893189,
650.462296651428));
#269935=CARTESIAN_POINT('Ctrl Pts',(-20.7744157382975,-158.704075916301,
648.462296651428));
#269936=CARTESIAN_POINT('Ctrl Pts',(-33.2646973929342,-157.069093939413,
646.462296651428));
#269937=CARTESIAN_POINT('Ctrl Pts',(-45.3454354230633,-153.500330774912,
644.462296651428));
#269938=CARTESIAN_POINT('Ctrl Pts',(-57.4261734531924,-149.931567610412,
642.462296651428));
#269939=CARTESIAN_POINT('Ctrl Pts',(-68.7998999948413,-144.516898051455,
640.462296651428));
#269940=CARTESIAN_POINT('Ctrl Pts',(-80.1736265364901,-139.102228492497,
638.462296651428));
#269941=CARTESIAN_POINT('Ctrl Pts',(-90.5602826949691,-131.974979673883,
636.462296651428));
#269942=CARTESIAN_POINT('Ctrl Pts',(-100.946938853448,-124.847730855269,
634.462296651428));
#269943=CARTESIAN_POINT('Ctrl Pts',(-110.0907706828,-116.183399296895,632.462296651428));
#269944=CARTESIAN_POINT('Ctrl Pts',(-119.234602512152,-107.519067738521,
630.462296651428));
#269945=CARTESIAN_POINT('Ctrl Pts',(-126.9104585261,-97.5309980386224,628.462296651428));
#269946=CARTESIAN_POINT('Ctrl Pts',(-134.586314540048,-87.5429283387234,
626.462296651428));
#269947=CARTESIAN_POINT('Ctrl Pts',(-140.605189688823,-76.4770599218137,
624.462296651428));
#269948=CARTESIAN_POINT('Ctrl Pts',(-146.624064837599,-65.4111915049041,
622.462296651428));
#269949=CARTESIAN_POINT('Ctrl Pts',(-150.837754439537,-53.5400027769199,
620.462296651428));
#269950=CARTESIAN_POINT('Ctrl Pts',(-155.051444041475,-41.6688140489356,
618.462296651428));
#269951=CARTESIAN_POINT('Ctrl Pts',(-157.356193074143,-29.2846130745764,
616.462296651428));
#269952=CARTESIAN_POINT('Ctrl Pts',(-159.660942106811,-16.9004121002171,
614.462296651428));
#269953=CARTESIAN_POINT('Ctrl Pts',(-160.,-4.30813900827815,612.462296651428));
#269954=CARTESIAN_POINT('Ctrl Pts',(-160.339057893189,8.28413408366081,
610.462296651428));
#269955=CARTESIAN_POINT('Ctrl Pts',(-158.704075916301,20.7744157382975,
608.462296651428));
#269956=CARTESIAN_POINT('Ctrl Pts',(-157.069093939413,33.2646973929342,
606.462296651428));
#269957=CARTESIAN_POINT('Ctrl Pts',(-153.500330774912,45.3454354230633,
604.462296651428));
#269958=CARTESIAN_POINT('Ctrl Pts',(-149.931567610412,57.4261734531924,
602.462296651428));
#269959=CARTESIAN_POINT('Ctrl Pts',(-144.516898051455,68.7998999948413,
600.462296651428));
#269960=CARTESIAN_POINT('Ctrl Pts',(-139.102228492497,80.1736265364901,
598.462296651428));
#269961=CARTESIAN_POINT('Ctrl Pts',(-131.974979673883,90.5602826949691,
596.462296651428));
#269962=CARTESIAN_POINT('Ctrl Pts',(-124.847730855269,100.946938853448,
594.462296651428));
#269963=CARTESIAN_POINT('Ctrl Pts',(-116.183399296895,110.0907706828,592.462296651428));
#269964=CARTESIAN_POINT('Ctrl Pts',(-107.519067738521,119.234602512152,
590.462296651428));
#269965=CARTESIAN_POINT('Ctrl Pts',(-97.5309980386224,126.9104585261,588.462296651428));
#269966=CARTESIAN_POINT('Ctrl Pts',(-87.5429283387233,134.586314540048,
586.462296651428));
#269967=CARTESIAN_POINT('Ctrl Pts',(-76.4770599218137,140.605189688823,
584.462296651428));
#269968=CARTESIAN_POINT('Ctrl Pts',(-65.4111915049042,146.624064837599,
582.462296651428));
#269969=CARTESIAN_POINT('Ctrl Pts',(-53.5400027769199,150.837754439537,
580.462296651428));
#269970=CARTESIAN_POINT('Ctrl Pts',(-41.6688140489356,155.051444041475,
578.462296651428));
#269971=CARTESIAN_POINT('Ctrl Pts',(-29.2846130745764,157.356193074143,
576.462296651428));
#269972=CARTESIAN_POINT('Ctrl Pts',(-16.9004121002172,159.660942106811,
574.462296651428));
#269973=CARTESIAN_POINT('Ctrl Pts',(-4.30813900827816,160.,572.462296651428));
#269974=CARTESIAN_POINT('Ctrl Pts',(8.28413408366087,160.339057893189,570.462296651428));
#269975=CARTESIAN_POINT('Ctrl Pts',(20.7744157382975,158.704075916301,568.462296651428));
#269976=CARTESIAN_POINT('Ctrl Pts',(33.2646973929342,157.069093939413,566.462296651428));
#269977=CARTESIAN_POINT('Ctrl Pts',(45.3454354230633,153.500330774912,564.462296651428));
#269978=CARTESIAN_POINT('Ctrl Pts',(57.4261734531925,149.931567610412,562.462296651428));
#269979=CARTESIAN_POINT('Ctrl Pts',(68.7998999948413,144.516898051455,560.462296651428));
#269980=CARTESIAN_POINT('Ctrl Pts',(80.1736265364901,139.102228492498,558.462296651428));
#269981=CARTESIAN_POINT('Ctrl Pts',(90.560282694969,131.974979673883,556.462296651428));
#269982=CARTESIAN_POINT('Ctrl Pts',(100.946938853448,124.847730855269,554.462296651428));
#269983=CARTESIAN_POINT('Ctrl Pts',(110.0907706828,116.183399296895,552.462296651428));
#269984=CARTESIAN_POINT('Ctrl Pts',(119.234602512152,107.519067738521,550.462296651428));
#269985=CARTESIAN_POINT('Ctrl Pts',(126.9104585261,97.5309980386224,548.462296651428));
#269986=CARTESIAN_POINT('Ctrl Pts',(134.586314540048,87.5429283387233,546.462296651428));
#269987=CARTESIAN_POINT('Ctrl Pts',(140.605189688823,76.4770599218137,544.462296651428));
#269988=CARTESIAN_POINT('Ctrl Pts',(146.624064837599,65.4111915049042,542.462296651428));
#269989=CARTESIAN_POINT('Ctrl Pts',(150.837754439537,53.5400027769199,540.462296651428));
#269990=CARTESIAN_POINT('Ctrl Pts',(155.051444041475,41.6688140489356,538.462296651428));
#269991=CARTESIAN_POINT('Ctrl Pts',(157.356193074143,29.2846130745764,536.462296651428));
#269992=CARTESIAN_POINT('Ctrl Pts',(159.394142202012,18.3340187941081,534.693818523022));
#269993=CARTESIAN_POINT('Ctrl Pts',(159.895664541343,7.20669984090287,532.923108716584));
#269994=CARTESIAN_POINT('Ctrl Pts',(159.895664541343,-7.20669984090406,
697.076891283416));
#269995=CARTESIAN_POINT('Ctrl Pts',(159.394142202012,-18.3340187941086,
695.306181476978));
#269996=CARTESIAN_POINT('Ctrl Pts',(157.356193074143,-29.2846130745763,
693.537703348572));
#269997=CARTESIAN_POINT('Ctrl Pts',(155.051444041475,-41.6688140489355,
691.537703348572));
#269998=CARTESIAN_POINT('Ctrl Pts',(150.837754439537,-53.5400027769198,
689.537703348572));
#269999=CARTESIAN_POINT('Ctrl Pts',(146.624064837599,-65.411191504904,687.537703348572));
#270000=CARTESIAN_POINT('Ctrl Pts',(140.605189688823,-76.4770599218136,
685.537703348572));
#270001=CARTESIAN_POINT('Ctrl Pts',(134.586314540048,-87.5429283387233,
683.537703348572));
#270002=CARTESIAN_POINT('Ctrl Pts',(126.9104585261,-97.5309980386223,681.537703348572));
#270003=CARTESIAN_POINT('Ctrl Pts',(119.234602512152,-107.519067738521,
679.537703348572));
#270004=CARTESIAN_POINT('Ctrl Pts',(110.0907706828,-116.183399296895,677.537703348572));
#270005=CARTESIAN_POINT('Ctrl Pts',(100.946938853448,-124.847730855269,
675.537703348572));
#270006=CARTESIAN_POINT('Ctrl Pts',(90.5602826949691,-131.974979673883,
673.537703348572));
#270007=CARTESIAN_POINT('Ctrl Pts',(80.1736265364902,-139.102228492497,
671.537703348572));
#270008=CARTESIAN_POINT('Ctrl Pts',(68.7998999948414,-144.516898051454,
669.537703348572));
#270009=CARTESIAN_POINT('Ctrl Pts',(57.4261734531925,-149.931567610412,
667.537703348572));
#270010=CARTESIAN_POINT('Ctrl Pts',(45.3454354230634,-153.500330774912,
665.537703348572));
#270011=CARTESIAN_POINT('Ctrl Pts',(33.2646973929343,-157.069093939413,
663.537703348572));
#270012=CARTESIAN_POINT('Ctrl Pts',(20.7744157382976,-158.704075916301,
661.537703348572));
#270013=CARTESIAN_POINT('Ctrl Pts',(8.28413408366091,-160.339057893189,
659.537703348572));
#270014=CARTESIAN_POINT('Ctrl Pts',(-4.30813900827804,-160.,657.537703348572));
#270015=CARTESIAN_POINT('Ctrl Pts',(-16.900412100217,-159.660942106811,
655.537703348572));
#270016=CARTESIAN_POINT('Ctrl Pts',(-29.2846130745763,-157.356193074143,
653.537703348572));
#270017=CARTESIAN_POINT('Ctrl Pts',(-41.6688140489355,-155.051444041475,
651.537703348572));
#270018=CARTESIAN_POINT('Ctrl Pts',(-53.5400027769198,-150.837754439537,
649.537703348572));
#270019=CARTESIAN_POINT('Ctrl Pts',(-65.411191504904,-146.624064837599,
647.537703348572));
#270020=CARTESIAN_POINT('Ctrl Pts',(-76.4770599218136,-140.605189688823,
645.537703348572));
#270021=CARTESIAN_POINT('Ctrl Pts',(-87.5429283387233,-134.586314540048,
643.537703348572));
#270022=CARTESIAN_POINT('Ctrl Pts',(-97.5309980386223,-126.9104585261,641.537703348572));
#270023=CARTESIAN_POINT('Ctrl Pts',(-107.519067738521,-119.234602512152,
639.537703348572));
#270024=CARTESIAN_POINT('Ctrl Pts',(-116.183399296895,-110.0907706828,637.537703348572));
#270025=CARTESIAN_POINT('Ctrl Pts',(-124.847730855269,-100.946938853448,
635.537703348572));
#270026=CARTESIAN_POINT('Ctrl Pts',(-131.974979673883,-90.5602826949692,
633.537703348572));
#270027=CARTESIAN_POINT('Ctrl Pts',(-139.102228492497,-80.1736265364902,
631.537703348572));
#270028=CARTESIAN_POINT('Ctrl Pts',(-144.516898051454,-68.7998999948414,
629.537703348572));
#270029=CARTESIAN_POINT('Ctrl Pts',(-149.931567610412,-57.4261734531925,
627.537703348572));
#270030=CARTESIAN_POINT('Ctrl Pts',(-153.500330774912,-45.3454354230634,
625.537703348572));
#270031=CARTESIAN_POINT('Ctrl Pts',(-157.069093939413,-33.2646973929344,
623.537703348572));
#270032=CARTESIAN_POINT('Ctrl Pts',(-158.704075916301,-20.7744157382976,
621.537703348572));
#270033=CARTESIAN_POINT('Ctrl Pts',(-160.339057893189,-8.28413408366092,
619.537703348572));
#270034=CARTESIAN_POINT('Ctrl Pts',(-160.,4.30813900827803,617.537703348572));
#270035=CARTESIAN_POINT('Ctrl Pts',(-159.660942106811,16.900412100217,615.537703348572));
#270036=CARTESIAN_POINT('Ctrl Pts',(-157.356193074143,29.2846130745763,
613.537703348572));
#270037=CARTESIAN_POINT('Ctrl Pts',(-155.051444041475,41.6688140489355,
611.537703348572));
#270038=CARTESIAN_POINT('Ctrl Pts',(-150.837754439537,53.5400027769198,
609.537703348572));
#270039=CARTESIAN_POINT('Ctrl Pts',(-146.624064837599,65.411191504904,607.537703348572));
#270040=CARTESIAN_POINT('Ctrl Pts',(-140.605189688823,76.4770599218136,
605.537703348572));
#270041=CARTESIAN_POINT('Ctrl Pts',(-134.586314540048,87.5429283387233,
603.537703348572));
#270042=CARTESIAN_POINT('Ctrl Pts',(-126.9104585261,97.5309980386223,601.537703348572));
#270043=CARTESIAN_POINT('Ctrl Pts',(-119.234602512152,107.519067738521,
599.537703348572));
#270044=CARTESIAN_POINT('Ctrl Pts',(-110.0907706828,116.183399296895,597.537703348572));
#270045=CARTESIAN_POINT('Ctrl Pts',(-100.946938853448,124.847730855269,
595.537703348572));
#270046=CARTESIAN_POINT('Ctrl Pts',(-90.5602826949692,131.974979673883,
593.537703348572));
#270047=CARTESIAN_POINT('Ctrl Pts',(-80.1736265364902,139.102228492497,
591.537703348572));
#270048=CARTESIAN_POINT('Ctrl Pts',(-68.7998999948414,144.516898051454,
589.537703348572));
#270049=CARTESIAN_POINT('Ctrl Pts',(-57.4261734531926,149.931567610412,
587.537703348572));
#270050=CARTESIAN_POINT('Ctrl Pts',(-45.3454354230634,153.500330774912,
585.537703348572));
#270051=CARTESIAN_POINT('Ctrl Pts',(-33.2646973929343,157.069093939413,
583.537703348572));
#270052=CARTESIAN_POINT('Ctrl Pts',(-20.7744157382976,158.704075916301,
581.537703348572));
#270053=CARTESIAN_POINT('Ctrl Pts',(-8.284134083661,160.339057893189,579.537703348572));
#270054=CARTESIAN_POINT('Ctrl Pts',(4.30813900827803,160.,577.537703348572));
#270055=CARTESIAN_POINT('Ctrl Pts',(16.9004121002171,159.660942106811,575.537703348572));
#270056=CARTESIAN_POINT('Ctrl Pts',(29.2846130745762,157.356193074143,573.537703348572));
#270057=CARTESIAN_POINT('Ctrl Pts',(41.6688140489354,155.051444041476,571.537703348572));
#270058=CARTESIAN_POINT('Ctrl Pts',(53.5400027769198,150.837754439537,569.537703348572));
#270059=CARTESIAN_POINT('Ctrl Pts',(65.4111915049041,146.624064837599,567.537703348572));
#270060=CARTESIAN_POINT('Ctrl Pts',(76.4770599218136,140.605189688823,565.537703348572));
#270061=CARTESIAN_POINT('Ctrl Pts',(87.5429283387232,134.586314540048,563.537703348572));
#270062=CARTESIAN_POINT('Ctrl Pts',(97.5309980386223,126.9104585261,561.537703348572));
#270063=CARTESIAN_POINT('Ctrl Pts',(107.519067738521,119.234602512152,559.537703348572));
#270064=CARTESIAN_POINT('Ctrl Pts',(116.183399296895,110.0907706828,557.537703348572));
#270065=CARTESIAN_POINT('Ctrl Pts',(124.847730855269,100.946938853448,555.537703348572));
#270066=CARTESIAN_POINT('Ctrl Pts',(131.974979673883,90.5602826949692,553.537703348572));
#270067=CARTESIAN_POINT('Ctrl Pts',(139.102228492497,80.1736265364902,551.537703348572));
#270068=CARTESIAN_POINT('Ctrl Pts',(144.516898051454,68.7998999948414,549.537703348572));
#270069=CARTESIAN_POINT('Ctrl Pts',(149.931567610412,57.4261734531926,547.537703348572));
#270070=CARTESIAN_POINT('Ctrl Pts',(153.500330774912,45.3454354230634,545.537703348572));
#270071=CARTESIAN_POINT('Ctrl Pts',(157.069093939413,33.2646973929343,543.537703348572));
#270072=CARTESIAN_POINT('Ctrl Pts',(158.704075916301,20.7744157382976,541.537703348572));
#270073=CARTESIAN_POINT('Ctrl Pts',(159.653854600275,13.5186762622035,540.375881753716));
#270074=CARTESIAN_POINT('Ctrl Pts',(159.937609420477,6.20654127333082,539.210563551645));
#270075=CARTESIAN_POINT('Ctrl Pts',(130.,4.30813900827812,692.462296651428));
#270076=CARTESIAN_POINT('Ctrl Pts',(130.339057893189,-5.92308287892228,
690.462296651428));
#270077=CARTESIAN_POINT('Ctrl Pts',(129.073425698447,-16.0813817870906,
688.462296651428));
#270078=CARTESIAN_POINT('Ctrl Pts',(127.807793503704,-26.2396806952589,
686.462296651429));
#270079=CARTESIAN_POINT('Ctrl Pts',(124.968635286058,-36.0749255918149,
684.462296651428));
#270080=CARTESIAN_POINT('Ctrl Pts',(122.129477068411,-45.9101704883709,
682.462296651428));
#270081=CARTESIAN_POINT('Ctrl Pts',(117.786702325803,-55.1801850026549,
680.462296651428));
#270082=CARTESIAN_POINT('Ctrl Pts',(113.443927583196,-64.4501995169389,
678.462296651428));
#270083=CARTESIAN_POINT('Ctrl Pts',(107.704469842635,-72.9267251261949,
676.462296651428));
#270084=CARTESIAN_POINT('Ctrl Pts',(101.965012102074,-81.4032507354509,
674.462296651428));
#270085=CARTESIAN_POINT('Ctrl Pts',(94.9701958612989,-88.8775672472035,
672.462296651428));
#270086=CARTESIAN_POINT('Ctrl Pts',(87.9753796205242,-96.351883758956,670.462296651428));
#270087=CARTESIAN_POINT('Ctrl Pts',(79.8974404698481,-102.639948694851,
668.462296651428));
#270088=CARTESIAN_POINT('Ctrl Pts',(71.8195013191721,-108.928013630747,
666.462296651428));
#270089=CARTESIAN_POINT('Ctrl Pts',(62.8573449296273,-113.874993963172,
664.462296651428));
#270090=CARTESIAN_POINT('Ctrl Pts',(53.8951885400825,-118.821974295598,
662.462296651428));
#270091=CARTESIAN_POINT('Ctrl Pts',(44.2694929456714,-122.306058950682,
660.462296651428));
#270092=CARTESIAN_POINT('Ctrl Pts',(34.6437973512603,-125.790143605767,
658.462296651428));
#270093=CARTESIAN_POINT('Ctrl Pts',(24.5915791233694,-127.725542856289,
656.462296651428));
#270094=CARTESIAN_POINT('Ctrl Pts',(14.5393608954785,-129.660942106811,
654.462296651428));
#270095=CARTESIAN_POINT('Ctrl Pts',(4.30813900827813,-130.,652.462296651428));
#270096=CARTESIAN_POINT('Ctrl Pts',(-5.92308287892227,-130.339057893189,
650.462296651428));
#270097=CARTESIAN_POINT('Ctrl Pts',(-16.0813817870906,-129.073425698447,
648.462296651428));
#270098=CARTESIAN_POINT('Ctrl Pts',(-26.2396806952589,-127.807793503705,
646.462296651428));
#270099=CARTESIAN_POINT('Ctrl Pts',(-36.0749255918149,-124.968635286058,
644.462296651428));
#270100=CARTESIAN_POINT('Ctrl Pts',(-45.9101704883709,-122.129477068411,
642.462296651428));
#270101=CARTESIAN_POINT('Ctrl Pts',(-55.1801850026549,-117.786702325803,
640.462296651428));
#270102=CARTESIAN_POINT('Ctrl Pts',(-64.4501995169389,-113.443927583196,
638.462296651428));
#270103=CARTESIAN_POINT('Ctrl Pts',(-72.9267251261949,-107.704469842635,
636.462296651428));
#270104=CARTESIAN_POINT('Ctrl Pts',(-81.4032507354509,-101.965012102074,
634.462296651428));
#270105=CARTESIAN_POINT('Ctrl Pts',(-88.8775672472034,-94.9701958612989,
632.462296651428));
#270106=CARTESIAN_POINT('Ctrl Pts',(-96.351883758956,-87.9753796205242,
630.462296651428));
#270107=CARTESIAN_POINT('Ctrl Pts',(-102.639948694851,-79.8974404698482,
628.462296651428));
#270108=CARTESIAN_POINT('Ctrl Pts',(-108.928013630747,-71.8195013191721,
626.462296651429));
#270109=CARTESIAN_POINT('Ctrl Pts',(-113.874993963172,-62.8573449296273,
624.462296651428));
#270110=CARTESIAN_POINT('Ctrl Pts',(-118.821974295598,-53.8951885400825,
622.462296651428));
#270111=CARTESIAN_POINT('Ctrl Pts',(-122.306058950682,-44.2694929456714,
620.462296651428));
#270112=CARTESIAN_POINT('Ctrl Pts',(-125.790143605767,-34.6437973512603,
618.462296651428));
#270113=CARTESIAN_POINT('Ctrl Pts',(-127.725542856289,-24.5915791233694,
616.462296651428));
#270114=CARTESIAN_POINT('Ctrl Pts',(-129.660942106811,-14.5393608954785,
614.462296651429));
#270115=CARTESIAN_POINT('Ctrl Pts',(-130.,-4.30813900827813,612.462296651428));
#270116=CARTESIAN_POINT('Ctrl Pts',(-130.339057893189,5.92308287892227,
610.462296651428));
#270117=CARTESIAN_POINT('Ctrl Pts',(-129.073425698447,16.0813817870906,
608.462296651428));
#270118=CARTESIAN_POINT('Ctrl Pts',(-127.807793503705,26.2396806952589,
606.462296651428));
#270119=CARTESIAN_POINT('Ctrl Pts',(-124.968635286058,36.0749255918149,
604.462296651428));
#270120=CARTESIAN_POINT('Ctrl Pts',(-122.129477068411,45.9101704883709,
602.462296651429));
#270121=CARTESIAN_POINT('Ctrl Pts',(-117.786702325803,55.1801850026549,
600.462296651428));
#270122=CARTESIAN_POINT('Ctrl Pts',(-113.443927583196,64.4501995169388,
598.462296651428));
#270123=CARTESIAN_POINT('Ctrl Pts',(-107.704469842635,72.9267251261949,
596.462296651428));
#270124=CARTESIAN_POINT('Ctrl Pts',(-101.965012102074,81.4032507354509,
594.462296651428));
#270125=CARTESIAN_POINT('Ctrl Pts',(-94.9701958612989,88.8775672472034,
592.462296651428));
#270126=CARTESIAN_POINT('Ctrl Pts',(-87.9753796205243,96.3518837589559,
590.462296651428));
#270127=CARTESIAN_POINT('Ctrl Pts',(-79.8974404698482,102.639948694851,
588.462296651428));
#270128=CARTESIAN_POINT('Ctrl Pts',(-71.819501319172,108.928013630747,586.462296651428));
#270129=CARTESIAN_POINT('Ctrl Pts',(-62.8573449296273,113.874993963172,
584.462296651428));
#270130=CARTESIAN_POINT('Ctrl Pts',(-53.8951885400826,118.821974295598,
582.462296651428));
#270131=CARTESIAN_POINT('Ctrl Pts',(-44.2694929456714,122.306058950682,
580.462296651428));
#270132=CARTESIAN_POINT('Ctrl Pts',(-34.6437973512603,125.790143605767,
578.462296651428));
#270133=CARTESIAN_POINT('Ctrl Pts',(-24.5915791233694,127.725542856289,
576.462296651428));
#270134=CARTESIAN_POINT('Ctrl Pts',(-14.5393608954786,129.660942106811,
574.462296651428));
#270135=CARTESIAN_POINT('Ctrl Pts',(-4.30813900827814,130.,572.462296651428));
#270136=CARTESIAN_POINT('Ctrl Pts',(5.92308287892232,130.339057893189,570.462296651428));
#270137=CARTESIAN_POINT('Ctrl Pts',(16.0813817870906,129.073425698447,568.462296651428));
#270138=CARTESIAN_POINT('Ctrl Pts',(26.2396806952589,127.807793503705,566.462296651428));
#270139=CARTESIAN_POINT('Ctrl Pts',(36.0749255918149,124.968635286058,564.462296651428));
#270140=CARTESIAN_POINT('Ctrl Pts',(45.9101704883709,122.129477068411,562.462296651428));
#270141=CARTESIAN_POINT('Ctrl Pts',(55.1801850026549,117.786702325803,560.462296651428));
#270142=CARTESIAN_POINT('Ctrl Pts',(64.4501995169388,113.443927583196,558.462296651428));
#270143=CARTESIAN_POINT('Ctrl Pts',(72.9267251261949,107.704469842635,556.462296651428));
#270144=CARTESIAN_POINT('Ctrl Pts',(81.4032507354509,101.965012102074,554.462296651428));
#270145=CARTESIAN_POINT('Ctrl Pts',(88.8775672472034,94.9701958612989,552.462296651428));
#270146=CARTESIAN_POINT('Ctrl Pts',(96.3518837589559,87.9753796205243,550.462296651428));
#270147=CARTESIAN_POINT('Ctrl Pts',(102.639948694851,79.8974404698482,548.462296651428));
#270148=CARTESIAN_POINT('Ctrl Pts',(108.928013630747,71.819501319172,546.462296651428));
#270149=CARTESIAN_POINT('Ctrl Pts',(113.874993963172,62.8573449296273,544.462296651428));
#270150=CARTESIAN_POINT('Ctrl Pts',(118.821974295598,53.8951885400826,542.462296651428));
#270151=CARTESIAN_POINT('Ctrl Pts',(122.306058950682,44.2694929456714,540.462296651428));
#270152=CARTESIAN_POINT('Ctrl Pts',(125.790143605767,34.6437973512603,538.462296651428));
#270153=CARTESIAN_POINT('Ctrl Pts',(127.725542856289,24.5915791233694,536.462296651428));
#270154=CARTESIAN_POINT('Ctrl Pts',(129.660942106811,14.5393608954786,534.462296651428));
#270155=CARTESIAN_POINT('Ctrl Pts',(130.,4.30813900827812,532.462296651428));
#270156=CARTESIAN_POINT('Ctrl Pts',(160.,4.30813900827813,692.462296651428));
#270157=CARTESIAN_POINT('Ctrl Pts',(160.339057893189,-8.28413408366083,
690.462296651428));
#270158=CARTESIAN_POINT('Ctrl Pts',(158.704075916301,-20.7744157382975,
688.462296651428));
#270159=CARTESIAN_POINT('Ctrl Pts',(157.069093939413,-33.2646973929343,
686.462296651429));
#270160=CARTESIAN_POINT('Ctrl Pts',(153.500330774912,-45.3454354230633,
684.462296651428));
#270161=CARTESIAN_POINT('Ctrl Pts',(149.931567610412,-57.4261734531924,
682.462296651428));
#270162=CARTESIAN_POINT('Ctrl Pts',(144.516898051455,-68.7998999948413,
680.462296651428));
#270163=CARTESIAN_POINT('Ctrl Pts',(139.102228492497,-80.1736265364901,
678.462296651428));
#270164=CARTESIAN_POINT('Ctrl Pts',(131.974979673883,-90.5602826949691,
676.462296651428));
#270165=CARTESIAN_POINT('Ctrl Pts',(124.847730855269,-100.946938853448,
674.462296651428));
#270166=CARTESIAN_POINT('Ctrl Pts',(116.183399296895,-110.0907706828,672.462296651428));
#270167=CARTESIAN_POINT('Ctrl Pts',(107.519067738521,-119.234602512152,
670.462296651428));
#270168=CARTESIAN_POINT('Ctrl Pts',(97.5309980386224,-126.9104585261,668.462296651428));
#270169=CARTESIAN_POINT('Ctrl Pts',(87.5429283387234,-134.586314540048,
666.462296651428));
#270170=CARTESIAN_POINT('Ctrl Pts',(76.4770599218137,-140.605189688823,
664.462296651428));
#270171=CARTESIAN_POINT('Ctrl Pts',(65.4111915049041,-146.624064837599,
662.462296651428));
#270172=CARTESIAN_POINT('Ctrl Pts',(53.5400027769198,-150.837754439537,
660.462296651428));
#270173=CARTESIAN_POINT('Ctrl Pts',(41.6688140489356,-155.051444041475,
658.462296651428));
#270174=CARTESIAN_POINT('Ctrl Pts',(29.2846130745764,-157.356193074143,
656.462296651428));
#270175=CARTESIAN_POINT('Ctrl Pts',(16.9004121002171,-159.660942106811,
654.462296651428));
#270176=CARTESIAN_POINT('Ctrl Pts',(4.30813900827814,-160.,652.462296651428));
#270177=CARTESIAN_POINT('Ctrl Pts',(-8.28413408366082,-160.339057893189,
650.462296651428));
#270178=CARTESIAN_POINT('Ctrl Pts',(-20.7744157382975,-158.704075916301,
648.462296651428));
#270179=CARTESIAN_POINT('Ctrl Pts',(-33.2646973929342,-157.069093939413,
646.462296651428));
#270180=CARTESIAN_POINT('Ctrl Pts',(-45.3454354230633,-153.500330774912,
644.462296651428));
#270181=CARTESIAN_POINT('Ctrl Pts',(-57.4261734531924,-149.931567610412,
642.462296651428));
#270182=CARTESIAN_POINT('Ctrl Pts',(-68.7998999948413,-144.516898051455,
640.462296651428));
#270183=CARTESIAN_POINT('Ctrl Pts',(-80.1736265364901,-139.102228492497,
638.462296651428));
#270184=CARTESIAN_POINT('Ctrl Pts',(-90.5602826949691,-131.974979673883,
636.462296651428));
#270185=CARTESIAN_POINT('Ctrl Pts',(-100.946938853448,-124.847730855269,
634.462296651428));
#270186=CARTESIAN_POINT('Ctrl Pts',(-110.0907706828,-116.183399296895,632.462296651428));
#270187=CARTESIAN_POINT('Ctrl Pts',(-119.234602512152,-107.519067738521,
630.462296651428));
#270188=CARTESIAN_POINT('Ctrl Pts',(-126.9104585261,-97.5309980386224,628.462296651428));
#270189=CARTESIAN_POINT('Ctrl Pts',(-134.586314540048,-87.5429283387234,
626.462296651429));
#270190=CARTESIAN_POINT('Ctrl Pts',(-140.605189688823,-76.4770599218137,
624.462296651428));
#270191=CARTESIAN_POINT('Ctrl Pts',(-146.624064837599,-65.4111915049041,
622.462296651428));
#270192=CARTESIAN_POINT('Ctrl Pts',(-150.837754439537,-53.5400027769199,
620.462296651428));
#270193=CARTESIAN_POINT('Ctrl Pts',(-155.051444041475,-41.6688140489356,
618.462296651428));
#270194=CARTESIAN_POINT('Ctrl Pts',(-157.356193074143,-29.2846130745764,
616.462296651428));
#270195=CARTESIAN_POINT('Ctrl Pts',(-159.660942106811,-16.9004121002171,
614.462296651429));
#270196=CARTESIAN_POINT('Ctrl Pts',(-160.,-4.30813900827815,612.462296651428));
#270197=CARTESIAN_POINT('Ctrl Pts',(-160.339057893189,8.28413408366081,
610.462296651428));
#270198=CARTESIAN_POINT('Ctrl Pts',(-158.704075916301,20.7744157382975,
608.462296651428));
#270199=CARTESIAN_POINT('Ctrl Pts',(-157.069093939413,33.2646973929342,
606.462296651428));
#270200=CARTESIAN_POINT('Ctrl Pts',(-153.500330774912,45.3454354230633,
604.462296651428));
#270201=CARTESIAN_POINT('Ctrl Pts',(-149.931567610412,57.4261734531924,
602.462296651429));
#270202=CARTESIAN_POINT('Ctrl Pts',(-144.516898051455,68.7998999948413,
600.462296651428));
#270203=CARTESIAN_POINT('Ctrl Pts',(-139.102228492497,80.1736265364901,
598.462296651428));
#270204=CARTESIAN_POINT('Ctrl Pts',(-131.974979673883,90.5602826949691,
596.462296651428));
#270205=CARTESIAN_POINT('Ctrl Pts',(-124.847730855269,100.946938853448,
594.462296651428));
#270206=CARTESIAN_POINT('Ctrl Pts',(-116.183399296895,110.0907706828,592.462296651428));
#270207=CARTESIAN_POINT('Ctrl Pts',(-107.519067738521,119.234602512152,
590.462296651428));
#270208=CARTESIAN_POINT('Ctrl Pts',(-97.5309980386224,126.9104585261,588.462296651428));
#270209=CARTESIAN_POINT('Ctrl Pts',(-87.5429283387233,134.586314540048,
586.462296651428));
#270210=CARTESIAN_POINT('Ctrl Pts',(-76.4770599218137,140.605189688823,
584.462296651428));
#270211=CARTESIAN_POINT('Ctrl Pts',(-65.4111915049042,146.624064837599,
582.462296651428));
#270212=CARTESIAN_POINT('Ctrl Pts',(-53.5400027769199,150.837754439537,
580.462296651428));
#270213=CARTESIAN_POINT('Ctrl Pts',(-41.6688140489356,155.051444041475,
578.462296651428));
#270214=CARTESIAN_POINT('Ctrl Pts',(-29.2846130745764,157.356193074143,
576.462296651428));
#270215=CARTESIAN_POINT('Ctrl Pts',(-16.9004121002172,159.660942106811,
574.462296651428));
#270216=CARTESIAN_POINT('Ctrl Pts',(-4.30813900827816,160.,572.462296651428));
#270217=CARTESIAN_POINT('Ctrl Pts',(8.28413408366087,160.339057893189,570.462296651428));
#270218=CARTESIAN_POINT('Ctrl Pts',(20.7744157382975,158.704075916301,568.462296651428));
#270219=CARTESIAN_POINT('Ctrl Pts',(33.2646973929342,157.069093939413,566.462296651428));
#270220=CARTESIAN_POINT('Ctrl Pts',(45.3454354230633,153.500330774912,564.462296651428));
#270221=CARTESIAN_POINT('Ctrl Pts',(57.4261734531925,149.931567610412,562.462296651428));
#270222=CARTESIAN_POINT('Ctrl Pts',(68.7998999948413,144.516898051455,560.462296651428));
#270223=CARTESIAN_POINT('Ctrl Pts',(80.1736265364901,139.102228492498,558.462296651428));
#270224=CARTESIAN_POINT('Ctrl Pts',(90.560282694969,131.974979673883,556.462296651428));
#270225=CARTESIAN_POINT('Ctrl Pts',(100.946938853448,124.847730855269,554.462296651428));
#270226=CARTESIAN_POINT('Ctrl Pts',(110.0907706828,116.183399296895,552.462296651428));
#270227=CARTESIAN_POINT('Ctrl Pts',(119.234602512152,107.519067738521,550.462296651428));
#270228=CARTESIAN_POINT('Ctrl Pts',(126.9104585261,97.5309980386224,548.462296651428));
#270229=CARTESIAN_POINT('Ctrl Pts',(134.586314540048,87.5429283387233,546.462296651428));
#270230=CARTESIAN_POINT('Ctrl Pts',(140.605189688823,76.4770599218137,544.462296651428));
#270231=CARTESIAN_POINT('Ctrl Pts',(146.624064837599,65.4111915049042,542.462296651428));
#270232=CARTESIAN_POINT('Ctrl Pts',(150.837754439537,53.5400027769199,540.462296651428));
#270233=CARTESIAN_POINT('Ctrl Pts',(155.051444041475,41.6688140489356,538.462296651428));
#270234=CARTESIAN_POINT('Ctrl Pts',(157.356193074143,29.2846130745764,536.462296651428));
#270235=CARTESIAN_POINT('Ctrl Pts',(159.660942106811,16.9004121002172,534.462296651428));
#270236=CARTESIAN_POINT('Ctrl Pts',(160.,4.30813900827813,532.462296651428));
#270237=CARTESIAN_POINT('Ctrl Pts',(129.934615416877,-5.96286660784778,
690.450909781393));
#270238=CARTESIAN_POINT('Ctrl Pts',(129.701667605591,-11.0389459941992,
689.45506834253));
#270239=CARTESIAN_POINT('Ctrl Pts',(129.073425698447,-16.0813817870906,
688.462296651428));
#270240=CARTESIAN_POINT('Ctrl Pts',(127.807793503704,-26.2396806952589,
686.462296651429));
#270241=CARTESIAN_POINT('Ctrl Pts',(124.968635286058,-36.0749255918149,
684.462296651428));
#270242=CARTESIAN_POINT('Ctrl Pts',(122.129477068411,-45.9101704883709,
682.462296651428));
#270243=CARTESIAN_POINT('Ctrl Pts',(117.786702325803,-55.1801850026549,
680.462296651428));
#270244=CARTESIAN_POINT('Ctrl Pts',(113.443927583196,-64.4501995169389,
678.462296651428));
#270245=CARTESIAN_POINT('Ctrl Pts',(107.704469842635,-72.9267251261949,
676.462296651428));
#270246=CARTESIAN_POINT('Ctrl Pts',(101.965012102074,-81.4032507354509,
674.462296651428));
#270247=CARTESIAN_POINT('Ctrl Pts',(94.9701958612989,-88.8775672472035,
672.462296651428));
#270248=CARTESIAN_POINT('Ctrl Pts',(87.9753796205242,-96.351883758956,670.462296651428));
#270249=CARTESIAN_POINT('Ctrl Pts',(79.8974404698481,-102.639948694851,
668.462296651428));
#270250=CARTESIAN_POINT('Ctrl Pts',(71.8195013191721,-108.928013630747,
666.462296651428));
#270251=CARTESIAN_POINT('Ctrl Pts',(62.8573449296273,-113.874993963172,
664.462296651428));
#270252=CARTESIAN_POINT('Ctrl Pts',(53.8951885400825,-118.821974295598,
662.462296651428));
#270253=CARTESIAN_POINT('Ctrl Pts',(44.2694929456714,-122.306058950682,
660.462296651428));
#270254=CARTESIAN_POINT('Ctrl Pts',(34.6437973512603,-125.790143605767,
658.462296651428));
#270255=CARTESIAN_POINT('Ctrl Pts',(24.5915791233694,-127.725542856289,
656.462296651428));
#270256=CARTESIAN_POINT('Ctrl Pts',(14.5393608954785,-129.660942106811,
654.462296651428));
#270257=CARTESIAN_POINT('Ctrl Pts',(4.30813900827813,-130.,652.462296651428));
#270258=CARTESIAN_POINT('Ctrl Pts',(-5.92308287892227,-130.339057893189,
650.462296651428));
#270259=CARTESIAN_POINT('Ctrl Pts',(-16.0813817870906,-129.073425698447,
648.462296651428));
#270260=CARTESIAN_POINT('Ctrl Pts',(-26.2396806952589,-127.807793503705,
646.462296651428));
#270261=CARTESIAN_POINT('Ctrl Pts',(-36.0749255918149,-124.968635286058,
644.462296651428));
#270262=CARTESIAN_POINT('Ctrl Pts',(-45.9101704883709,-122.129477068411,
642.462296651428));
#270263=CARTESIAN_POINT('Ctrl Pts',(-55.1801850026549,-117.786702325803,
640.462296651428));
#270264=CARTESIAN_POINT('Ctrl Pts',(-64.4501995169389,-113.443927583196,
638.462296651428));
#270265=CARTESIAN_POINT('Ctrl Pts',(-72.9267251261949,-107.704469842635,
636.462296651428));
#270266=CARTESIAN_POINT('Ctrl Pts',(-81.4032507354509,-101.965012102074,
634.462296651428));
#270267=CARTESIAN_POINT('Ctrl Pts',(-88.8775672472034,-94.9701958612989,
632.462296651428));
#270268=CARTESIAN_POINT('Ctrl Pts',(-96.351883758956,-87.9753796205242,
630.462296651428));
#270269=CARTESIAN_POINT('Ctrl Pts',(-102.639948694851,-79.8974404698482,
628.462296651428));
#270270=CARTESIAN_POINT('Ctrl Pts',(-108.928013630747,-71.8195013191721,
626.462296651428));
#270271=CARTESIAN_POINT('Ctrl Pts',(-113.874993963172,-62.8573449296273,
624.462296651428));
#270272=CARTESIAN_POINT('Ctrl Pts',(-118.821974295598,-53.8951885400825,
622.462296651428));
#270273=CARTESIAN_POINT('Ctrl Pts',(-122.306058950682,-44.2694929456714,
620.462296651428));
#270274=CARTESIAN_POINT('Ctrl Pts',(-125.790143605767,-34.6437973512603,
618.462296651428));
#270275=CARTESIAN_POINT('Ctrl Pts',(-127.725542856289,-24.5915791233694,
616.462296651428));
#270276=CARTESIAN_POINT('Ctrl Pts',(-129.660942106811,-14.5393608954785,
614.462296651428));
#270277=CARTESIAN_POINT('Ctrl Pts',(-130.,-4.30813900827813,612.462296651428));
#270278=CARTESIAN_POINT('Ctrl Pts',(-130.339057893189,5.92308287892227,
610.462296651428));
#270279=CARTESIAN_POINT('Ctrl Pts',(-129.073425698447,16.0813817870906,
608.462296651428));
#270280=CARTESIAN_POINT('Ctrl Pts',(-127.807793503705,26.2396806952589,
606.462296651428));
#270281=CARTESIAN_POINT('Ctrl Pts',(-124.968635286058,36.0749255918149,
604.462296651428));
#270282=CARTESIAN_POINT('Ctrl Pts',(-122.129477068411,45.9101704883709,
602.462296651428));
#270283=CARTESIAN_POINT('Ctrl Pts',(-117.786702325803,55.1801850026549,
600.462296651428));
#270284=CARTESIAN_POINT('Ctrl Pts',(-113.443927583196,64.4501995169388,
598.462296651428));
#270285=CARTESIAN_POINT('Ctrl Pts',(-107.704469842635,72.9267251261949,
596.462296651428));
#270286=CARTESIAN_POINT('Ctrl Pts',(-101.965012102074,81.4032507354509,
594.462296651428));
#270287=CARTESIAN_POINT('Ctrl Pts',(-94.9701958612989,88.8775672472034,
592.462296651428));
#270288=CARTESIAN_POINT('Ctrl Pts',(-87.9753796205243,96.3518837589559,
590.462296651428));
#270289=CARTESIAN_POINT('Ctrl Pts',(-79.8974404698482,102.639948694851,
588.462296651428));
#270290=CARTESIAN_POINT('Ctrl Pts',(-71.819501319172,108.928013630747,586.462296651428));
#270291=CARTESIAN_POINT('Ctrl Pts',(-62.8573449296273,113.874993963172,
584.462296651428));
#270292=CARTESIAN_POINT('Ctrl Pts',(-53.8951885400826,118.821974295598,
582.462296651428));
#270293=CARTESIAN_POINT('Ctrl Pts',(-44.2694929456714,122.306058950682,
580.462296651428));
#270294=CARTESIAN_POINT('Ctrl Pts',(-34.6437973512603,125.790143605767,
578.462296651428));
#270295=CARTESIAN_POINT('Ctrl Pts',(-24.5915791233694,127.725542856289,
576.462296651428));
#270296=CARTESIAN_POINT('Ctrl Pts',(-14.5393608954786,129.660942106811,
574.462296651428));
#270297=CARTESIAN_POINT('Ctrl Pts',(-4.30813900827814,130.,572.462296651428));
#270298=CARTESIAN_POINT('Ctrl Pts',(5.92308287892232,130.339057893189,570.462296651428));
#270299=CARTESIAN_POINT('Ctrl Pts',(16.0813817870906,129.073425698447,568.462296651428));
#270300=CARTESIAN_POINT('Ctrl Pts',(26.2396806952589,127.807793503705,566.462296651428));
#270301=CARTESIAN_POINT('Ctrl Pts',(36.0749255918149,124.968635286058,564.462296651428));
#270302=CARTESIAN_POINT('Ctrl Pts',(45.9101704883709,122.129477068411,562.462296651428));
#270303=CARTESIAN_POINT('Ctrl Pts',(55.1801850026549,117.786702325803,560.462296651428));
#270304=CARTESIAN_POINT('Ctrl Pts',(64.4501995169388,113.443927583196,558.462296651428));
#270305=CARTESIAN_POINT('Ctrl Pts',(72.9267251261949,107.704469842635,556.462296651428));
#270306=CARTESIAN_POINT('Ctrl Pts',(81.403250735451,101.965012102074,554.462296651428));
#270307=CARTESIAN_POINT('Ctrl Pts',(88.8775672472034,94.9701958612989,552.462296651428));
#270308=CARTESIAN_POINT('Ctrl Pts',(96.3518837589559,87.9753796205243,550.462296651428));
#270309=CARTESIAN_POINT('Ctrl Pts',(102.639948694851,79.8974404698482,548.462296651428));
#270310=CARTESIAN_POINT('Ctrl Pts',(108.928013630747,71.8195013191721,546.462296651428));
#270311=CARTESIAN_POINT('Ctrl Pts',(113.874993963172,62.8573449296273,544.462296651428));
#270312=CARTESIAN_POINT('Ctrl Pts',(118.821974295598,53.8951885400826,542.462296651428));
#270313=CARTESIAN_POINT('Ctrl Pts',(122.306058950682,44.2694929456714,540.462296651428));
#270314=CARTESIAN_POINT('Ctrl Pts',(125.790143605767,34.6437973512603,538.462296651428));
#270315=CARTESIAN_POINT('Ctrl Pts',(127.725542856289,24.5915791233694,536.462296651428));
#270316=CARTESIAN_POINT('Ctrl Pts',(129.382196958681,15.9871278397994,534.750345898172));
#270317=CARTESIAN_POINT('Ctrl Pts',(129.869812400585,7.23822414350004,533.035792462989));
#270318=CARTESIAN_POINT('Ctrl Pts',(130.,-4.30813900827807,697.537703348572));
#270319=CARTESIAN_POINT('Ctrl Pts',(129.660942106811,-14.5393608954785,
695.537703348572));
#270320=CARTESIAN_POINT('Ctrl Pts',(127.725542856289,-24.5915791233694,
693.537703348572));
#270321=CARTESIAN_POINT('Ctrl Pts',(125.790143605767,-34.6437973512603,
691.537703348572));
#270322=CARTESIAN_POINT('Ctrl Pts',(122.306058950682,-44.2694929456714,
689.537703348572));
#270323=CARTESIAN_POINT('Ctrl Pts',(118.821974295598,-53.8951885400825,
687.537703348572));
#270324=CARTESIAN_POINT('Ctrl Pts',(113.874993963172,-62.8573449296272,
685.537703348572));
#270325=CARTESIAN_POINT('Ctrl Pts',(108.928013630747,-71.819501319172,683.537703348572));
#270326=CARTESIAN_POINT('Ctrl Pts',(102.639948694851,-79.8974404698481,
681.537703348572));
#270327=CARTESIAN_POINT('Ctrl Pts',(96.351883758956,-87.9753796205242,679.537703348572));
#270328=CARTESIAN_POINT('Ctrl Pts',(88.8775672472035,-94.9701958612989,
677.537703348572));
#270329=CARTESIAN_POINT('Ctrl Pts',(81.403250735451,-101.965012102074,675.537703348572));
#270330=CARTESIAN_POINT('Ctrl Pts',(72.9267251261949,-107.704469842635,
673.537703348572));
#270331=CARTESIAN_POINT('Ctrl Pts',(64.4501995169389,-113.443927583196,
671.537703348572));
#270332=CARTESIAN_POINT('Ctrl Pts',(55.1801850026549,-117.786702325803,
669.537703348572));
#270333=CARTESIAN_POINT('Ctrl Pts',(45.910170488371,-122.129477068411,667.537703348572));
#270334=CARTESIAN_POINT('Ctrl Pts',(36.074925591815,-124.968635286058,665.537703348572));
#270335=CARTESIAN_POINT('Ctrl Pts',(26.239680695259,-127.807793503704,663.537703348572));
#270336=CARTESIAN_POINT('Ctrl Pts',(16.0813817870907,-129.073425698447,
661.537703348572));
#270337=CARTESIAN_POINT('Ctrl Pts',(5.92308287892234,-130.339057893189,
659.537703348572));
#270338=CARTESIAN_POINT('Ctrl Pts',(-4.30813900827806,-130.,657.537703348572));
#270339=CARTESIAN_POINT('Ctrl Pts',(-14.5393608954785,-129.660942106811,
655.537703348572));
#270340=CARTESIAN_POINT('Ctrl Pts',(-24.5915791233694,-127.725542856289,
653.537703348572));
#270341=CARTESIAN_POINT('Ctrl Pts',(-34.6437973512603,-125.790143605767,
651.537703348572));
#270342=CARTESIAN_POINT('Ctrl Pts',(-44.2694929456713,-122.306058950682,
649.537703348572));
#270343=CARTESIAN_POINT('Ctrl Pts',(-53.8951885400825,-118.821974295598,
647.537703348572));
#270344=CARTESIAN_POINT('Ctrl Pts',(-62.8573449296272,-113.874993963172,
645.537703348572));
#270345=CARTESIAN_POINT('Ctrl Pts',(-71.819501319172,-108.928013630747,
643.537703348572));
#270346=CARTESIAN_POINT('Ctrl Pts',(-79.8974404698481,-102.639948694851,
641.537703348572));
#270347=CARTESIAN_POINT('Ctrl Pts',(-87.9753796205242,-96.351883758956,
639.537703348572));
#270348=CARTESIAN_POINT('Ctrl Pts',(-94.9701958612989,-88.8775672472035,
637.537703348572));
#270349=CARTESIAN_POINT('Ctrl Pts',(-101.965012102074,-81.403250735451,
635.537703348572));
#270350=CARTESIAN_POINT('Ctrl Pts',(-107.704469842635,-72.9267251261949,
633.537703348572));
#270351=CARTESIAN_POINT('Ctrl Pts',(-113.443927583196,-64.4501995169389,
631.537703348572));
#270352=CARTESIAN_POINT('Ctrl Pts',(-117.786702325803,-55.1801850026549,
629.537703348572));
#270353=CARTESIAN_POINT('Ctrl Pts',(-122.129477068411,-45.910170488371,
627.537703348572));
#270354=CARTESIAN_POINT('Ctrl Pts',(-124.968635286058,-36.074925591815,
625.537703348572));
#270355=CARTESIAN_POINT('Ctrl Pts',(-127.807793503704,-26.239680695259,
623.537703348572));
#270356=CARTESIAN_POINT('Ctrl Pts',(-129.073425698447,-16.0813817870907,
621.537703348572));
#270357=CARTESIAN_POINT('Ctrl Pts',(-130.339057893189,-5.92308287892235,
619.537703348572));
#270358=CARTESIAN_POINT('Ctrl Pts',(-130.,4.30813900827805,617.537703348572));
#270359=CARTESIAN_POINT('Ctrl Pts',(-129.660942106811,14.5393608954784,
615.537703348572));
#270360=CARTESIAN_POINT('Ctrl Pts',(-127.725542856289,24.5915791233693,
613.537703348572));
#270361=CARTESIAN_POINT('Ctrl Pts',(-125.790143605767,34.6437973512602,
611.537703348572));
#270362=CARTESIAN_POINT('Ctrl Pts',(-122.306058950682,44.2694929456713,
609.537703348572));
#270363=CARTESIAN_POINT('Ctrl Pts',(-118.821974295598,53.8951885400825,
607.537703348572));
#270364=CARTESIAN_POINT('Ctrl Pts',(-113.874993963172,62.8573449296272,
605.537703348572));
#270365=CARTESIAN_POINT('Ctrl Pts',(-108.928013630747,71.819501319172,603.537703348572));
#270366=CARTESIAN_POINT('Ctrl Pts',(-102.639948694851,79.8974404698481,
601.537703348572));
#270367=CARTESIAN_POINT('Ctrl Pts',(-96.3518837589561,87.9753796205242,
599.537703348572));
#270368=CARTESIAN_POINT('Ctrl Pts',(-88.8775672472035,94.9701958612989,
597.537703348572));
#270369=CARTESIAN_POINT('Ctrl Pts',(-81.403250735451,101.965012102074,595.537703348572));
#270370=CARTESIAN_POINT('Ctrl Pts',(-72.9267251261949,107.704469842635,
593.537703348572));
#270371=CARTESIAN_POINT('Ctrl Pts',(-64.4501995169389,113.443927583196,
591.537703348572));
#270372=CARTESIAN_POINT('Ctrl Pts',(-55.1801850026549,117.786702325803,
589.537703348572));
#270373=CARTESIAN_POINT('Ctrl Pts',(-45.910170488371,122.129477068411,587.537703348572));
#270374=CARTESIAN_POINT('Ctrl Pts',(-36.074925591815,124.968635286058,585.537703348572));
#270375=CARTESIAN_POINT('Ctrl Pts',(-26.239680695259,127.807793503704,583.537703348572));
#270376=CARTESIAN_POINT('Ctrl Pts',(-16.0813817870907,129.073425698447,
581.537703348572));
#270377=CARTESIAN_POINT('Ctrl Pts',(-5.92308287892242,130.339057893189,
579.537703348572));
#270378=CARTESIAN_POINT('Ctrl Pts',(4.30813900827804,130.,577.537703348572));
#270379=CARTESIAN_POINT('Ctrl Pts',(14.5393608954785,129.660942106811,575.537703348572));
#270380=CARTESIAN_POINT('Ctrl Pts',(24.5915791233693,127.725542856289,573.537703348572));
#270381=CARTESIAN_POINT('Ctrl Pts',(34.6437973512602,125.790143605767,571.537703348572));
#270382=CARTESIAN_POINT('Ctrl Pts',(44.2694929456713,122.306058950682,569.537703348572));
#270383=CARTESIAN_POINT('Ctrl Pts',(53.8951885400825,118.821974295598,567.537703348572));
#270384=CARTESIAN_POINT('Ctrl Pts',(62.8573449296272,113.874993963172,565.537703348572));
#270385=CARTESIAN_POINT('Ctrl Pts',(71.819501319172,108.928013630747,563.537703348572));
#270386=CARTESIAN_POINT('Ctrl Pts',(79.8974404698481,102.639948694851,561.537703348572));
#270387=CARTESIAN_POINT('Ctrl Pts',(87.9753796205242,96.351883758956,559.537703348572));
#270388=CARTESIAN_POINT('Ctrl Pts',(94.9701958612989,88.8775672472035,557.537703348572));
#270389=CARTESIAN_POINT('Ctrl Pts',(101.965012102074,81.403250735451,555.537703348572));
#270390=CARTESIAN_POINT('Ctrl Pts',(107.704469842635,72.926725126195,553.537703348572));
#270391=CARTESIAN_POINT('Ctrl Pts',(113.443927583196,64.4501995169389,551.537703348572));
#270392=CARTESIAN_POINT('Ctrl Pts',(117.786702325803,55.1801850026549,549.537703348572));
#270393=CARTESIAN_POINT('Ctrl Pts',(122.129477068411,45.910170488371,547.537703348572));
#270394=CARTESIAN_POINT('Ctrl Pts',(124.968635286058,36.074925591815,545.537703348572));
#270395=CARTESIAN_POINT('Ctrl Pts',(127.807793503704,26.239680695259,543.537703348572));
#270396=CARTESIAN_POINT('Ctrl Pts',(129.073425698447,16.0813817870907,541.537703348572));
#270397=CARTESIAN_POINT('Ctrl Pts',(130.339057893189,5.92308287892242,539.537703348572));
#270398=CARTESIAN_POINT('Ctrl Pts',(130.,-4.30813900827807,537.537703348572));
#270399=CARTESIAN_POINT('Ctrl Pts',(130.,4.30813900827812,692.462296651428));
#270400=CARTESIAN_POINT('Ctrl Pts',(130.339057893189,-5.92308287892228,
690.462296651428));
#270401=CARTESIAN_POINT('Ctrl Pts',(129.073425698447,-16.0813817870906,
688.462296651428));
#270402=CARTESIAN_POINT('Ctrl Pts',(127.807793503704,-26.2396806952589,
686.462296651429));
#270403=CARTESIAN_POINT('Ctrl Pts',(124.968635286058,-36.0749255918149,
684.462296651428));
#270404=CARTESIAN_POINT('Ctrl Pts',(122.129477068411,-45.9101704883709,
682.462296651428));
#270405=CARTESIAN_POINT('Ctrl Pts',(117.786702325803,-55.1801850026549,
680.462296651428));
#270406=CARTESIAN_POINT('Ctrl Pts',(113.443927583196,-64.4501995169389,
678.462296651428));
#270407=CARTESIAN_POINT('Ctrl Pts',(107.704469842635,-72.9267251261949,
676.462296651428));
#270408=CARTESIAN_POINT('Ctrl Pts',(101.965012102074,-81.4032507354509,
674.462296651428));
#270409=CARTESIAN_POINT('Ctrl Pts',(94.9701958612989,-88.8775672472035,
672.462296651428));
#270410=CARTESIAN_POINT('Ctrl Pts',(87.9753796205242,-96.351883758956,670.462296651428));
#270411=CARTESIAN_POINT('Ctrl Pts',(79.8974404698481,-102.639948694851,
668.462296651428));
#270412=CARTESIAN_POINT('Ctrl Pts',(71.8195013191721,-108.928013630747,
666.462296651428));
#270413=CARTESIAN_POINT('Ctrl Pts',(62.8573449296273,-113.874993963172,
664.462296651428));
#270414=CARTESIAN_POINT('Ctrl Pts',(53.8951885400825,-118.821974295598,
662.462296651428));
#270415=CARTESIAN_POINT('Ctrl Pts',(44.2694929456714,-122.306058950682,
660.462296651428));
#270416=CARTESIAN_POINT('Ctrl Pts',(34.6437973512603,-125.790143605767,
658.462296651428));
#270417=CARTESIAN_POINT('Ctrl Pts',(24.5915791233694,-127.725542856289,
656.462296651428));
#270418=CARTESIAN_POINT('Ctrl Pts',(14.5393608954785,-129.660942106811,
654.462296651428));
#270419=CARTESIAN_POINT('Ctrl Pts',(4.30813900827813,-130.,652.462296651428));
#270420=CARTESIAN_POINT('Ctrl Pts',(-5.92308287892227,-130.339057893189,
650.462296651428));
#270421=CARTESIAN_POINT('Ctrl Pts',(-16.0813817870906,-129.073425698447,
648.462296651428));
#270422=CARTESIAN_POINT('Ctrl Pts',(-26.2396806952589,-127.807793503705,
646.462296651428));
#270423=CARTESIAN_POINT('Ctrl Pts',(-36.0749255918149,-124.968635286058,
644.462296651428));
#270424=CARTESIAN_POINT('Ctrl Pts',(-45.9101704883709,-122.129477068411,
642.462296651428));
#270425=CARTESIAN_POINT('Ctrl Pts',(-55.1801850026549,-117.786702325803,
640.462296651428));
#270426=CARTESIAN_POINT('Ctrl Pts',(-64.4501995169389,-113.443927583196,
638.462296651428));
#270427=CARTESIAN_POINT('Ctrl Pts',(-72.9267251261949,-107.704469842635,
636.462296651428));
#270428=CARTESIAN_POINT('Ctrl Pts',(-81.4032507354509,-101.965012102074,
634.462296651428));
#270429=CARTESIAN_POINT('Ctrl Pts',(-88.8775672472034,-94.9701958612989,
632.462296651428));
#270430=CARTESIAN_POINT('Ctrl Pts',(-96.351883758956,-87.9753796205242,
630.462296651428));
#270431=CARTESIAN_POINT('Ctrl Pts',(-102.639948694851,-79.8974404698482,
628.462296651428));
#270432=CARTESIAN_POINT('Ctrl Pts',(-108.928013630747,-71.8195013191721,
626.462296651429));
#270433=CARTESIAN_POINT('Ctrl Pts',(-113.874993963172,-62.8573449296273,
624.462296651428));
#270434=CARTESIAN_POINT('Ctrl Pts',(-118.821974295598,-53.8951885400825,
622.462296651428));
#270435=CARTESIAN_POINT('Ctrl Pts',(-122.306058950682,-44.2694929456714,
620.462296651428));
#270436=CARTESIAN_POINT('Ctrl Pts',(-125.790143605767,-34.6437973512603,
618.462296651428));
#270437=CARTESIAN_POINT('Ctrl Pts',(-127.725542856289,-24.5915791233694,
616.462296651428));
#270438=CARTESIAN_POINT('Ctrl Pts',(-129.660942106811,-14.5393608954785,
614.462296651429));
#270439=CARTESIAN_POINT('Ctrl Pts',(-130.,-4.30813900827813,612.462296651428));
#270440=CARTESIAN_POINT('Ctrl Pts',(-130.339057893189,5.92308287892227,
610.462296651428));
#270441=CARTESIAN_POINT('Ctrl Pts',(-129.073425698447,16.0813817870906,
608.462296651428));
#270442=CARTESIAN_POINT('Ctrl Pts',(-127.807793503705,26.2396806952589,
606.462296651428));
#270443=CARTESIAN_POINT('Ctrl Pts',(-124.968635286058,36.0749255918149,
604.462296651428));
#270444=CARTESIAN_POINT('Ctrl Pts',(-122.129477068411,45.9101704883709,
602.462296651429));
#270445=CARTESIAN_POINT('Ctrl Pts',(-117.786702325803,55.1801850026549,
600.462296651428));
#270446=CARTESIAN_POINT('Ctrl Pts',(-113.443927583196,64.4501995169388,
598.462296651428));
#270447=CARTESIAN_POINT('Ctrl Pts',(-107.704469842635,72.9267251261949,
596.462296651428));
#270448=CARTESIAN_POINT('Ctrl Pts',(-101.965012102074,81.4032507354509,
594.462296651428));
#270449=CARTESIAN_POINT('Ctrl Pts',(-94.9701958612989,88.8775672472034,
592.462296651428));
#270450=CARTESIAN_POINT('Ctrl Pts',(-87.9753796205243,96.3518837589559,
590.462296651428));
#270451=CARTESIAN_POINT('Ctrl Pts',(-79.8974404698482,102.639948694851,
588.462296651428));
#270452=CARTESIAN_POINT('Ctrl Pts',(-71.819501319172,108.928013630747,586.462296651428));
#270453=CARTESIAN_POINT('Ctrl Pts',(-62.8573449296273,113.874993963172,
584.462296651428));
#270454=CARTESIAN_POINT('Ctrl Pts',(-53.8951885400826,118.821974295598,
582.462296651428));
#270455=CARTESIAN_POINT('Ctrl Pts',(-44.2694929456714,122.306058950682,
580.462296651428));
#270456=CARTESIAN_POINT('Ctrl Pts',(-34.6437973512603,125.790143605767,
578.462296651428));
#270457=CARTESIAN_POINT('Ctrl Pts',(-24.5915791233694,127.725542856289,
576.462296651428));
#270458=CARTESIAN_POINT('Ctrl Pts',(-14.5393608954786,129.660942106811,
574.462296651428));
#270459=CARTESIAN_POINT('Ctrl Pts',(-4.30813900827814,130.,572.462296651428));
#270460=CARTESIAN_POINT('Ctrl Pts',(5.92308287892232,130.339057893189,570.462296651428));
#270461=CARTESIAN_POINT('Ctrl Pts',(16.0813817870906,129.073425698447,568.462296651428));
#270462=CARTESIAN_POINT('Ctrl Pts',(26.2396806952589,127.807793503705,566.462296651428));
#270463=CARTESIAN_POINT('Ctrl Pts',(36.0749255918149,124.968635286058,564.462296651428));
#270464=CARTESIAN_POINT('Ctrl Pts',(45.9101704883709,122.129477068411,562.462296651428));
#270465=CARTESIAN_POINT('Ctrl Pts',(55.1801850026549,117.786702325803,560.462296651428));
#270466=CARTESIAN_POINT('Ctrl Pts',(64.4501995169388,113.443927583196,558.462296651428));
#270467=CARTESIAN_POINT('Ctrl Pts',(72.9267251261949,107.704469842635,556.462296651428));
#270468=CARTESIAN_POINT('Ctrl Pts',(81.4032507354509,101.965012102074,554.462296651428));
#270469=CARTESIAN_POINT('Ctrl Pts',(88.8775672472034,94.9701958612989,552.462296651428));
#270470=CARTESIAN_POINT('Ctrl Pts',(96.3518837589559,87.9753796205243,550.462296651428));
#270471=CARTESIAN_POINT('Ctrl Pts',(102.639948694851,79.8974404698482,548.462296651428));
#270472=CARTESIAN_POINT('Ctrl Pts',(108.928013630747,71.819501319172,546.462296651428));
#270473=CARTESIAN_POINT('Ctrl Pts',(113.874993963172,62.8573449296273,544.462296651428));
#270474=CARTESIAN_POINT('Ctrl Pts',(118.821974295598,53.8951885400826,542.462296651428));
#270475=CARTESIAN_POINT('Ctrl Pts',(122.306058950682,44.2694929456714,540.462296651428));
#270476=CARTESIAN_POINT('Ctrl Pts',(125.790143605767,34.6437973512603,538.462296651428));
#270477=CARTESIAN_POINT('Ctrl Pts',(127.725542856289,24.5915791233694,536.462296651428));
#270478=CARTESIAN_POINT('Ctrl Pts',(129.660942106811,14.5393608954786,534.462296651428));
#270479=CARTESIAN_POINT('Ctrl Pts',(130.,4.30813900827812,532.462296651428));
#270480=CARTESIAN_POINT('Ctrl Pts',(129.869812400585,-7.23822414350117,
696.964207537011));
#270481=CARTESIAN_POINT('Ctrl Pts',(129.382196958681,-15.9871278397999,
695.249654101829));
#270482=CARTESIAN_POINT('Ctrl Pts',(127.725542856289,-24.5915791233694,
693.537703348572));
#270483=CARTESIAN_POINT('Ctrl Pts',(125.790143605767,-34.6437973512603,
691.537703348572));
#270484=CARTESIAN_POINT('Ctrl Pts',(122.306058950682,-44.2694929456714,
689.537703348572));
#270485=CARTESIAN_POINT('Ctrl Pts',(118.821974295598,-53.8951885400825,
687.537703348572));
#270486=CARTESIAN_POINT('Ctrl Pts',(113.874993963172,-62.8573449296272,
685.537703348572));
#270487=CARTESIAN_POINT('Ctrl Pts',(108.928013630747,-71.819501319172,683.537703348572));
#270488=CARTESIAN_POINT('Ctrl Pts',(102.639948694851,-79.8974404698481,
681.537703348572));
#270489=CARTESIAN_POINT('Ctrl Pts',(96.351883758956,-87.9753796205242,679.537703348572));
#270490=CARTESIAN_POINT('Ctrl Pts',(88.8775672472035,-94.9701958612989,
677.537703348572));
#270491=CARTESIAN_POINT('Ctrl Pts',(81.403250735451,-101.965012102074,675.537703348572));
#270492=CARTESIAN_POINT('Ctrl Pts',(72.9267251261949,-107.704469842635,
673.537703348572));
#270493=CARTESIAN_POINT('Ctrl Pts',(64.4501995169389,-113.443927583196,
671.537703348572));
#270494=CARTESIAN_POINT('Ctrl Pts',(55.1801850026549,-117.786702325803,
669.537703348572));
#270495=CARTESIAN_POINT('Ctrl Pts',(45.910170488371,-122.129477068411,667.537703348572));
#270496=CARTESIAN_POINT('Ctrl Pts',(36.074925591815,-124.968635286058,665.537703348572));
#270497=CARTESIAN_POINT('Ctrl Pts',(26.239680695259,-127.807793503704,663.537703348572));
#270498=CARTESIAN_POINT('Ctrl Pts',(16.0813817870907,-129.073425698447,
661.537703348572));
#270499=CARTESIAN_POINT('Ctrl Pts',(5.92308287892234,-130.339057893189,
659.537703348572));
#270500=CARTESIAN_POINT('Ctrl Pts',(-4.30813900827806,-130.,657.537703348572));
#270501=CARTESIAN_POINT('Ctrl Pts',(-14.5393608954785,-129.660942106811,
655.537703348572));
#270502=CARTESIAN_POINT('Ctrl Pts',(-24.5915791233694,-127.725542856289,
653.537703348572));
#270503=CARTESIAN_POINT('Ctrl Pts',(-34.6437973512602,-125.790143605767,
651.537703348572));
#270504=CARTESIAN_POINT('Ctrl Pts',(-44.2694929456713,-122.306058950682,
649.537703348572));
#270505=CARTESIAN_POINT('Ctrl Pts',(-53.8951885400825,-118.821974295598,
647.537703348572));
#270506=CARTESIAN_POINT('Ctrl Pts',(-62.8573449296272,-113.874993963172,
645.537703348572));
#270507=CARTESIAN_POINT('Ctrl Pts',(-71.819501319172,-108.928013630747,
643.537703348572));
#270508=CARTESIAN_POINT('Ctrl Pts',(-79.8974404698481,-102.639948694851,
641.537703348572));
#270509=CARTESIAN_POINT('Ctrl Pts',(-87.9753796205242,-96.351883758956,
639.537703348572));
#270510=CARTESIAN_POINT('Ctrl Pts',(-94.9701958612989,-88.8775672472035,
637.537703348572));
#270511=CARTESIAN_POINT('Ctrl Pts',(-101.965012102074,-81.403250735451,
635.537703348572));
#270512=CARTESIAN_POINT('Ctrl Pts',(-107.704469842635,-72.9267251261949,
633.537703348572));
#270513=CARTESIAN_POINT('Ctrl Pts',(-113.443927583196,-64.4501995169389,
631.537703348572));
#270514=CARTESIAN_POINT('Ctrl Pts',(-117.786702325803,-55.1801850026549,
629.537703348572));
#270515=CARTESIAN_POINT('Ctrl Pts',(-122.129477068411,-45.910170488371,
627.537703348572));
#270516=CARTESIAN_POINT('Ctrl Pts',(-124.968635286058,-36.074925591815,
625.537703348572));
#270517=CARTESIAN_POINT('Ctrl Pts',(-127.807793503704,-26.239680695259,
623.537703348572));
#270518=CARTESIAN_POINT('Ctrl Pts',(-129.073425698447,-16.0813817870907,
621.537703348572));
#270519=CARTESIAN_POINT('Ctrl Pts',(-130.339057893189,-5.92308287892235,
619.537703348572));
#270520=CARTESIAN_POINT('Ctrl Pts',(-130.,4.30813900827805,617.537703348572));
#270521=CARTESIAN_POINT('Ctrl Pts',(-129.660942106811,14.5393608954784,
615.537703348572));
#270522=CARTESIAN_POINT('Ctrl Pts',(-127.725542856289,24.5915791233693,
613.537703348572));
#270523=CARTESIAN_POINT('Ctrl Pts',(-125.790143605767,34.6437973512602,
611.537703348572));
#270524=CARTESIAN_POINT('Ctrl Pts',(-122.306058950682,44.2694929456713,
609.537703348572));
#270525=CARTESIAN_POINT('Ctrl Pts',(-118.821974295598,53.8951885400825,
607.537703348572));
#270526=CARTESIAN_POINT('Ctrl Pts',(-113.874993963172,62.8573449296272,
605.537703348572));
#270527=CARTESIAN_POINT('Ctrl Pts',(-108.928013630747,71.819501319172,603.537703348572));
#270528=CARTESIAN_POINT('Ctrl Pts',(-102.639948694851,79.8974404698481,
601.537703348572));
#270529=CARTESIAN_POINT('Ctrl Pts',(-96.3518837589561,87.9753796205242,
599.537703348572));
#270530=CARTESIAN_POINT('Ctrl Pts',(-88.8775672472035,94.9701958612989,
597.537703348572));
#270531=CARTESIAN_POINT('Ctrl Pts',(-81.403250735451,101.965012102074,595.537703348572));
#270532=CARTESIAN_POINT('Ctrl Pts',(-72.9267251261949,107.704469842635,
593.537703348572));
#270533=CARTESIAN_POINT('Ctrl Pts',(-64.4501995169389,113.443927583196,
591.537703348572));
#270534=CARTESIAN_POINT('Ctrl Pts',(-55.1801850026549,117.786702325803,
589.537703348572));
#270535=CARTESIAN_POINT('Ctrl Pts',(-45.910170488371,122.129477068411,587.537703348572));
#270536=CARTESIAN_POINT('Ctrl Pts',(-36.074925591815,124.968635286058,585.537703348572));
#270537=CARTESIAN_POINT('Ctrl Pts',(-26.239680695259,127.807793503704,583.537703348572));
#270538=CARTESIAN_POINT('Ctrl Pts',(-16.0813817870907,129.073425698447,
581.537703348572));
#270539=CARTESIAN_POINT('Ctrl Pts',(-5.92308287892242,130.339057893189,
579.537703348572));
#270540=CARTESIAN_POINT('Ctrl Pts',(4.30813900827804,130.,577.537703348572));
#270541=CARTESIAN_POINT('Ctrl Pts',(14.5393608954785,129.660942106811,575.537703348572));
#270542=CARTESIAN_POINT('Ctrl Pts',(24.5915791233693,127.725542856289,573.537703348572));
#270543=CARTESIAN_POINT('Ctrl Pts',(34.6437973512602,125.790143605767,571.537703348572));
#270544=CARTESIAN_POINT('Ctrl Pts',(44.2694929456713,122.306058950682,569.537703348572));
#270545=CARTESIAN_POINT('Ctrl Pts',(53.8951885400825,118.821974295598,567.537703348572));
#270546=CARTESIAN_POINT('Ctrl Pts',(62.8573449296272,113.874993963172,565.537703348572));
#270547=CARTESIAN_POINT('Ctrl Pts',(71.819501319172,108.928013630747,563.537703348572));
#270548=CARTESIAN_POINT('Ctrl Pts',(79.8974404698481,102.639948694851,561.537703348572));
#270549=CARTESIAN_POINT('Ctrl Pts',(87.9753796205242,96.351883758956,559.537703348572));
#270550=CARTESIAN_POINT('Ctrl Pts',(94.9701958612989,88.8775672472035,557.537703348572));
#270551=CARTESIAN_POINT('Ctrl Pts',(101.965012102074,81.403250735451,555.537703348572));
#270552=CARTESIAN_POINT('Ctrl Pts',(107.704469842635,72.926725126195,553.537703348572));
#270553=CARTESIAN_POINT('Ctrl Pts',(113.443927583196,64.4501995169389,551.537703348572));
#270554=CARTESIAN_POINT('Ctrl Pts',(117.786702325803,55.1801850026549,549.537703348572));
#270555=CARTESIAN_POINT('Ctrl Pts',(122.129477068411,45.910170488371,547.537703348572));
#270556=CARTESIAN_POINT('Ctrl Pts',(124.968635286058,36.074925591815,545.537703348572));
#270557=CARTESIAN_POINT('Ctrl Pts',(127.807793503704,26.239680695259,543.537703348572));
#270558=CARTESIAN_POINT('Ctrl Pts',(129.073425698447,16.0813817870907,541.537703348572));
#270559=CARTESIAN_POINT('Ctrl Pts',(129.701667605591,11.0389459941988,540.54493165747));
#270560=CARTESIAN_POINT('Ctrl Pts',(129.934615416877,5.96286660784701,539.549090218607));
#270561=CARTESIAN_POINT('Ctrl Pts',(160.,-4.30813900827805,697.537703348572));
#270562=CARTESIAN_POINT('Ctrl Pts',(159.660942106811,-16.900412100217,695.537703348572));
#270563=CARTESIAN_POINT('Ctrl Pts',(157.356193074143,-29.2846130745763,
693.537703348572));
#270564=CARTESIAN_POINT('Ctrl Pts',(155.051444041475,-41.6688140489355,
691.537703348572));
#270565=CARTESIAN_POINT('Ctrl Pts',(150.837754439537,-53.5400027769198,
689.537703348572));
#270566=CARTESIAN_POINT('Ctrl Pts',(146.624064837599,-65.411191504904,687.537703348572));
#270567=CARTESIAN_POINT('Ctrl Pts',(140.605189688823,-76.4770599218136,
685.537703348572));
#270568=CARTESIAN_POINT('Ctrl Pts',(134.586314540048,-87.5429283387233,
683.537703348572));
#270569=CARTESIAN_POINT('Ctrl Pts',(126.9104585261,-97.5309980386223,681.537703348572));
#270570=CARTESIAN_POINT('Ctrl Pts',(119.234602512152,-107.519067738521,
679.537703348572));
#270571=CARTESIAN_POINT('Ctrl Pts',(110.0907706828,-116.183399296895,677.537703348572));
#270572=CARTESIAN_POINT('Ctrl Pts',(100.946938853448,-124.847730855269,
675.537703348572));
#270573=CARTESIAN_POINT('Ctrl Pts',(90.5602826949691,-131.974979673883,
673.537703348572));
#270574=CARTESIAN_POINT('Ctrl Pts',(80.1736265364902,-139.102228492497,
671.537703348572));
#270575=CARTESIAN_POINT('Ctrl Pts',(68.7998999948414,-144.516898051454,
669.537703348572));
#270576=CARTESIAN_POINT('Ctrl Pts',(57.4261734531925,-149.931567610412,
667.537703348572));
#270577=CARTESIAN_POINT('Ctrl Pts',(45.3454354230634,-153.500330774912,
665.537703348572));
#270578=CARTESIAN_POINT('Ctrl Pts',(33.2646973929343,-157.069093939413,
663.537703348572));
#270579=CARTESIAN_POINT('Ctrl Pts',(20.7744157382976,-158.704075916301,
661.537703348572));
#270580=CARTESIAN_POINT('Ctrl Pts',(8.28413408366091,-160.339057893189,
659.537703348572));
#270581=CARTESIAN_POINT('Ctrl Pts',(-4.30813900827804,-160.,657.537703348572));
#270582=CARTESIAN_POINT('Ctrl Pts',(-16.900412100217,-159.660942106811,
655.537703348572));
#270583=CARTESIAN_POINT('Ctrl Pts',(-29.2846130745763,-157.356193074143,
653.537703348572));
#270584=CARTESIAN_POINT('Ctrl Pts',(-41.6688140489355,-155.051444041475,
651.537703348572));
#270585=CARTESIAN_POINT('Ctrl Pts',(-53.5400027769198,-150.837754439537,
649.537703348572));
#270586=CARTESIAN_POINT('Ctrl Pts',(-65.411191504904,-146.624064837599,
647.537703348572));
#270587=CARTESIAN_POINT('Ctrl Pts',(-76.4770599218136,-140.605189688823,
645.537703348572));
#270588=CARTESIAN_POINT('Ctrl Pts',(-87.5429283387233,-134.586314540048,
643.537703348572));
#270589=CARTESIAN_POINT('Ctrl Pts',(-97.5309980386223,-126.9104585261,641.537703348572));
#270590=CARTESIAN_POINT('Ctrl Pts',(-107.519067738521,-119.234602512152,
639.537703348572));
#270591=CARTESIAN_POINT('Ctrl Pts',(-116.183399296895,-110.0907706828,637.537703348572));
#270592=CARTESIAN_POINT('Ctrl Pts',(-124.847730855269,-100.946938853448,
635.537703348572));
#270593=CARTESIAN_POINT('Ctrl Pts',(-131.974979673883,-90.5602826949692,
633.537703348572));
#270594=CARTESIAN_POINT('Ctrl Pts',(-139.102228492497,-80.1736265364902,
631.537703348572));
#270595=CARTESIAN_POINT('Ctrl Pts',(-144.516898051454,-68.7998999948414,
629.537703348572));
#270596=CARTESIAN_POINT('Ctrl Pts',(-149.931567610412,-57.4261734531925,
627.537703348572));
#270597=CARTESIAN_POINT('Ctrl Pts',(-153.500330774912,-45.3454354230634,
625.537703348572));
#270598=CARTESIAN_POINT('Ctrl Pts',(-157.069093939413,-33.2646973929344,
623.537703348572));
#270599=CARTESIAN_POINT('Ctrl Pts',(-158.704075916301,-20.7744157382976,
621.537703348572));
#270600=CARTESIAN_POINT('Ctrl Pts',(-160.339057893189,-8.28413408366092,
619.537703348572));
#270601=CARTESIAN_POINT('Ctrl Pts',(-160.,4.30813900827803,617.537703348572));
#270602=CARTESIAN_POINT('Ctrl Pts',(-159.660942106811,16.900412100217,615.537703348572));
#270603=CARTESIAN_POINT('Ctrl Pts',(-157.356193074143,29.2846130745763,
613.537703348572));
#270604=CARTESIAN_POINT('Ctrl Pts',(-155.051444041475,41.6688140489355,
611.537703348572));
#270605=CARTESIAN_POINT('Ctrl Pts',(-150.837754439537,53.5400027769198,
609.537703348572));
#270606=CARTESIAN_POINT('Ctrl Pts',(-146.624064837599,65.411191504904,607.537703348572));
#270607=CARTESIAN_POINT('Ctrl Pts',(-140.605189688823,76.4770599218136,
605.537703348572));
#270608=CARTESIAN_POINT('Ctrl Pts',(-134.586314540048,87.5429283387233,
603.537703348572));
#270609=CARTESIAN_POINT('Ctrl Pts',(-126.9104585261,97.5309980386223,601.537703348572));
#270610=CARTESIAN_POINT('Ctrl Pts',(-119.234602512152,107.519067738521,
599.537703348572));
#270611=CARTESIAN_POINT('Ctrl Pts',(-110.0907706828,116.183399296895,597.537703348572));
#270612=CARTESIAN_POINT('Ctrl Pts',(-100.946938853448,124.847730855269,
595.537703348572));
#270613=CARTESIAN_POINT('Ctrl Pts',(-90.5602826949692,131.974979673883,
593.537703348572));
#270614=CARTESIAN_POINT('Ctrl Pts',(-80.1736265364901,139.102228492497,
591.537703348572));
#270615=CARTESIAN_POINT('Ctrl Pts',(-68.7998999948414,144.516898051454,
589.537703348572));
#270616=CARTESIAN_POINT('Ctrl Pts',(-57.4261734531926,149.931567610412,
587.537703348572));
#270617=CARTESIAN_POINT('Ctrl Pts',(-45.3454354230634,153.500330774912,
585.537703348572));
#270618=CARTESIAN_POINT('Ctrl Pts',(-33.2646973929343,157.069093939413,
583.537703348572));
#270619=CARTESIAN_POINT('Ctrl Pts',(-20.7744157382976,158.704075916301,
581.537703348572));
#270620=CARTESIAN_POINT('Ctrl Pts',(-8.284134083661,160.339057893189,579.537703348572));
#270621=CARTESIAN_POINT('Ctrl Pts',(4.30813900827803,160.,577.537703348572));
#270622=CARTESIAN_POINT('Ctrl Pts',(16.9004121002171,159.660942106811,575.537703348572));
#270623=CARTESIAN_POINT('Ctrl Pts',(29.2846130745762,157.356193074143,573.537703348572));
#270624=CARTESIAN_POINT('Ctrl Pts',(41.6688140489354,155.051444041476,571.537703348572));
#270625=CARTESIAN_POINT('Ctrl Pts',(53.5400027769198,150.837754439537,569.537703348572));
#270626=CARTESIAN_POINT('Ctrl Pts',(65.4111915049041,146.624064837599,567.537703348572));
#270627=CARTESIAN_POINT('Ctrl Pts',(76.4770599218136,140.605189688823,565.537703348572));
#270628=CARTESIAN_POINT('Ctrl Pts',(87.5429283387232,134.586314540048,563.537703348572));
#270629=CARTESIAN_POINT('Ctrl Pts',(97.5309980386223,126.9104585261,561.537703348572));
#270630=CARTESIAN_POINT('Ctrl Pts',(107.519067738521,119.234602512152,559.537703348572));
#270631=CARTESIAN_POINT('Ctrl Pts',(116.183399296895,110.0907706828,557.537703348572));
#270632=CARTESIAN_POINT('Ctrl Pts',(124.847730855269,100.946938853448,555.537703348572));
#270633=CARTESIAN_POINT('Ctrl Pts',(131.974979673883,90.5602826949692,553.537703348572));
#270634=CARTESIAN_POINT('Ctrl Pts',(139.102228492497,80.1736265364902,551.537703348572));
#270635=CARTESIAN_POINT('Ctrl Pts',(144.516898051454,68.7998999948414,549.537703348572));
#270636=CARTESIAN_POINT('Ctrl Pts',(149.931567610412,57.4261734531926,547.537703348572));
#270637=CARTESIAN_POINT('Ctrl Pts',(153.500330774912,45.3454354230634,545.537703348572));
#270638=CARTESIAN_POINT('Ctrl Pts',(157.069093939413,33.2646973929343,543.537703348572));
#270639=CARTESIAN_POINT('Ctrl Pts',(158.704075916301,20.7744157382976,541.537703348572));
#270640=CARTESIAN_POINT('Ctrl Pts',(160.339057893189,8.28413408366101,539.537703348572));
#270641=CARTESIAN_POINT('Ctrl Pts',(160.,-4.30813900827805,537.537703348572));
#270642=CARTESIAN_POINT('Ctrl Pts',(130.,-4.30813900827807,697.537703348572));
#270643=CARTESIAN_POINT('Ctrl Pts',(129.660942106811,-14.5393608954785,
695.537703348572));
#270644=CARTESIAN_POINT('Ctrl Pts',(127.725542856289,-24.5915791233694,
693.537703348572));
#270645=CARTESIAN_POINT('Ctrl Pts',(125.790143605767,-34.6437973512603,
691.537703348572));
#270646=CARTESIAN_POINT('Ctrl Pts',(122.306058950682,-44.2694929456714,
689.537703348572));
#270647=CARTESIAN_POINT('Ctrl Pts',(118.821974295598,-53.8951885400825,
687.537703348572));
#270648=CARTESIAN_POINT('Ctrl Pts',(113.874993963172,-62.8573449296272,
685.537703348572));
#270649=CARTESIAN_POINT('Ctrl Pts',(108.928013630747,-71.819501319172,683.537703348572));
#270650=CARTESIAN_POINT('Ctrl Pts',(102.639948694851,-79.8974404698481,
681.537703348572));
#270651=CARTESIAN_POINT('Ctrl Pts',(96.351883758956,-87.9753796205242,679.537703348572));
#270652=CARTESIAN_POINT('Ctrl Pts',(88.8775672472035,-94.9701958612989,
677.537703348572));
#270653=CARTESIAN_POINT('Ctrl Pts',(81.403250735451,-101.965012102074,675.537703348572));
#270654=CARTESIAN_POINT('Ctrl Pts',(72.9267251261949,-107.704469842635,
673.537703348572));
#270655=CARTESIAN_POINT('Ctrl Pts',(64.4501995169389,-113.443927583196,
671.537703348572));
#270656=CARTESIAN_POINT('Ctrl Pts',(55.1801850026549,-117.786702325803,
669.537703348572));
#270657=CARTESIAN_POINT('Ctrl Pts',(45.910170488371,-122.129477068411,667.537703348572));
#270658=CARTESIAN_POINT('Ctrl Pts',(36.074925591815,-124.968635286058,665.537703348572));
#270659=CARTESIAN_POINT('Ctrl Pts',(26.239680695259,-127.807793503704,663.537703348572));
#270660=CARTESIAN_POINT('Ctrl Pts',(16.0813817870907,-129.073425698447,
661.537703348572));
#270661=CARTESIAN_POINT('Ctrl Pts',(5.92308287892234,-130.339057893189,
659.537703348572));
#270662=CARTESIAN_POINT('Ctrl Pts',(-4.30813900827806,-130.,657.537703348572));
#270663=CARTESIAN_POINT('Ctrl Pts',(-14.5393608954785,-129.660942106811,
655.537703348572));
#270664=CARTESIAN_POINT('Ctrl Pts',(-24.5915791233694,-127.725542856289,
653.537703348572));
#270665=CARTESIAN_POINT('Ctrl Pts',(-34.6437973512603,-125.790143605767,
651.537703348572));
#270666=CARTESIAN_POINT('Ctrl Pts',(-44.2694929456713,-122.306058950682,
649.537703348572));
#270667=CARTESIAN_POINT('Ctrl Pts',(-53.8951885400825,-118.821974295598,
647.537703348572));
#270668=CARTESIAN_POINT('Ctrl Pts',(-62.8573449296272,-113.874993963172,
645.537703348572));
#270669=CARTESIAN_POINT('Ctrl Pts',(-71.819501319172,-108.928013630747,
643.537703348572));
#270670=CARTESIAN_POINT('Ctrl Pts',(-79.8974404698481,-102.639948694851,
641.537703348572));
#270671=CARTESIAN_POINT('Ctrl Pts',(-87.9753796205242,-96.351883758956,
639.537703348572));
#270672=CARTESIAN_POINT('Ctrl Pts',(-94.9701958612989,-88.8775672472035,
637.537703348572));
#270673=CARTESIAN_POINT('Ctrl Pts',(-101.965012102074,-81.403250735451,
635.537703348572));
#270674=CARTESIAN_POINT('Ctrl Pts',(-107.704469842635,-72.9267251261949,
633.537703348572));
#270675=CARTESIAN_POINT('Ctrl Pts',(-113.443927583196,-64.4501995169389,
631.537703348572));
#270676=CARTESIAN_POINT('Ctrl Pts',(-117.786702325803,-55.1801850026549,
629.537703348572));
#270677=CARTESIAN_POINT('Ctrl Pts',(-122.129477068411,-45.910170488371,
627.537703348572));
#270678=CARTESIAN_POINT('Ctrl Pts',(-124.968635286058,-36.074925591815,
625.537703348572));
#270679=CARTESIAN_POINT('Ctrl Pts',(-127.807793503704,-26.239680695259,
623.537703348572));
#270680=CARTESIAN_POINT('Ctrl Pts',(-129.073425698447,-16.0813817870907,
621.537703348572));
#270681=CARTESIAN_POINT('Ctrl Pts',(-130.339057893189,-5.92308287892235,
619.537703348572));
#270682=CARTESIAN_POINT('Ctrl Pts',(-130.,4.30813900827805,617.537703348572));
#270683=CARTESIAN_POINT('Ctrl Pts',(-129.660942106811,14.5393608954784,
615.537703348572));
#270684=CARTESIAN_POINT('Ctrl Pts',(-127.725542856289,24.5915791233693,
613.537703348572));
#270685=CARTESIAN_POINT('Ctrl Pts',(-125.790143605767,34.6437973512602,
611.537703348572));
#270686=CARTESIAN_POINT('Ctrl Pts',(-122.306058950682,44.2694929456713,
609.537703348572));
#270687=CARTESIAN_POINT('Ctrl Pts',(-118.821974295598,53.8951885400825,
607.537703348572));
#270688=CARTESIAN_POINT('Ctrl Pts',(-113.874993963172,62.8573449296272,
605.537703348572));
#270689=CARTESIAN_POINT('Ctrl Pts',(-108.928013630747,71.819501319172,603.537703348572));
#270690=CARTESIAN_POINT('Ctrl Pts',(-102.639948694851,79.8974404698481,
601.537703348572));
#270691=CARTESIAN_POINT('Ctrl Pts',(-96.3518837589561,87.9753796205242,
599.537703348572));
#270692=CARTESIAN_POINT('Ctrl Pts',(-88.8775672472035,94.9701958612989,
597.537703348572));
#270693=CARTESIAN_POINT('Ctrl Pts',(-81.403250735451,101.965012102074,595.537703348572));
#270694=CARTESIAN_POINT('Ctrl Pts',(-72.9267251261949,107.704469842635,
593.537703348572));
#270695=CARTESIAN_POINT('Ctrl Pts',(-64.4501995169389,113.443927583196,
591.537703348572));
#270696=CARTESIAN_POINT('Ctrl Pts',(-55.1801850026549,117.786702325803,
589.537703348572));
#270697=CARTESIAN_POINT('Ctrl Pts',(-45.910170488371,122.129477068411,587.537703348572));
#270698=CARTESIAN_POINT('Ctrl Pts',(-36.074925591815,124.968635286058,585.537703348572));
#270699=CARTESIAN_POINT('Ctrl Pts',(-26.239680695259,127.807793503704,583.537703348572));
#270700=CARTESIAN_POINT('Ctrl Pts',(-16.0813817870907,129.073425698447,
581.537703348572));
#270701=CARTESIAN_POINT('Ctrl Pts',(-5.92308287892242,130.339057893189,
579.537703348572));
#270702=CARTESIAN_POINT('Ctrl Pts',(4.30813900827804,130.,577.537703348572));
#270703=CARTESIAN_POINT('Ctrl Pts',(14.5393608954785,129.660942106811,575.537703348572));
#270704=CARTESIAN_POINT('Ctrl Pts',(24.5915791233693,127.725542856289,573.537703348572));
#270705=CARTESIAN_POINT('Ctrl Pts',(34.6437973512602,125.790143605767,571.537703348572));
#270706=CARTESIAN_POINT('Ctrl Pts',(44.2694929456713,122.306058950682,569.537703348572));
#270707=CARTESIAN_POINT('Ctrl Pts',(53.8951885400825,118.821974295598,567.537703348572));
#270708=CARTESIAN_POINT('Ctrl Pts',(62.8573449296272,113.874993963172,565.537703348572));
#270709=CARTESIAN_POINT('Ctrl Pts',(71.819501319172,108.928013630747,563.537703348572));
#270710=CARTESIAN_POINT('Ctrl Pts',(79.8974404698481,102.639948694851,561.537703348572));
#270711=CARTESIAN_POINT('Ctrl Pts',(87.9753796205242,96.351883758956,559.537703348572));
#270712=CARTESIAN_POINT('Ctrl Pts',(94.9701958612989,88.8775672472035,557.537703348572));
#270713=CARTESIAN_POINT('Ctrl Pts',(101.965012102074,81.403250735451,555.537703348572));
#270714=CARTESIAN_POINT('Ctrl Pts',(107.704469842635,72.926725126195,553.537703348572));
#270715=CARTESIAN_POINT('Ctrl Pts',(113.443927583196,64.4501995169389,551.537703348572));
#270716=CARTESIAN_POINT('Ctrl Pts',(117.786702325803,55.1801850026549,549.537703348572));
#270717=CARTESIAN_POINT('Ctrl Pts',(122.129477068411,45.910170488371,547.537703348572));
#270718=CARTESIAN_POINT('Ctrl Pts',(124.968635286058,36.074925591815,545.537703348572));
#270719=CARTESIAN_POINT('Ctrl Pts',(127.807793503704,26.239680695259,543.537703348572));
#270720=CARTESIAN_POINT('Ctrl Pts',(129.073425698447,16.0813817870907,541.537703348572));
#270721=CARTESIAN_POINT('Ctrl Pts',(130.339057893189,5.92308287892242,539.537703348572));
#270722=CARTESIAN_POINT('Ctrl Pts',(130.,-4.30813900827807,537.537703348572));
#270723=CARTESIAN_POINT('Ctrl Pts',(130.,-4.30813900827807,537.537703348572));
#270724=CARTESIAN_POINT('Ctrl Pts',(129.660942106811,-14.5393608954785,
535.537703348572));
#270725=CARTESIAN_POINT('Ctrl Pts',(127.725542856289,-24.5915791233694,
533.537703348572));
#270726=CARTESIAN_POINT('Ctrl Pts',(125.790143605767,-34.6437973512603,
531.537703348572));
#270727=CARTESIAN_POINT('Ctrl Pts',(122.306058950682,-44.2694929456714,
529.537703348572));
#270728=CARTESIAN_POINT('Ctrl Pts',(118.821974295598,-53.8951885400825,
527.537703348572));
#270729=CARTESIAN_POINT('Ctrl Pts',(113.874993963172,-62.8573449296272,
525.537703348572));
#270730=CARTESIAN_POINT('Ctrl Pts',(108.928013630747,-71.819501319172,523.537703348572));
#270731=CARTESIAN_POINT('Ctrl Pts',(102.639948694851,-79.8974404698481,
521.537703348572));
#270732=CARTESIAN_POINT('Ctrl Pts',(96.351883758956,-87.9753796205242,519.537703348572));
#270733=CARTESIAN_POINT('Ctrl Pts',(88.8775672472035,-94.9701958612989,
517.537703348572));
#270734=CARTESIAN_POINT('Ctrl Pts',(81.403250735451,-101.965012102074,515.537703348572));
#270735=CARTESIAN_POINT('Ctrl Pts',(72.9267251261949,-107.704469842635,
513.537703348572));
#270736=CARTESIAN_POINT('Ctrl Pts',(64.4501995169389,-113.443927583196,
511.537703348572));
#270737=CARTESIAN_POINT('Ctrl Pts',(55.1801850026549,-117.786702325803,
509.537703348572));
#270738=CARTESIAN_POINT('Ctrl Pts',(45.910170488371,-122.129477068411,507.537703348572));
#270739=CARTESIAN_POINT('Ctrl Pts',(36.074925591815,-124.968635286058,505.537703348572));
#270740=CARTESIAN_POINT('Ctrl Pts',(26.239680695259,-127.807793503704,503.537703348572));
#270741=CARTESIAN_POINT('Ctrl Pts',(16.0813817870907,-129.073425698447,
501.537703348572));
#270742=CARTESIAN_POINT('Ctrl Pts',(5.92308287892234,-130.339057893189,
499.537703348572));
#270743=CARTESIAN_POINT('Ctrl Pts',(-4.30813900827806,-130.,497.537703348572));
#270744=CARTESIAN_POINT('Ctrl Pts',(-14.5393608954785,-129.660942106811,
495.537703348572));
#270745=CARTESIAN_POINT('Ctrl Pts',(-24.5915791233694,-127.725542856289,
493.537703348572));
#270746=CARTESIAN_POINT('Ctrl Pts',(-34.6437973512603,-125.790143605767,
491.537703348572));
#270747=CARTESIAN_POINT('Ctrl Pts',(-44.2694929456713,-122.306058950682,
489.537703348572));
#270748=CARTESIAN_POINT('Ctrl Pts',(-53.8951885400825,-118.821974295598,
487.537703348572));
#270749=CARTESIAN_POINT('Ctrl Pts',(-62.8573449296272,-113.874993963172,
485.537703348572));
#270750=CARTESIAN_POINT('Ctrl Pts',(-71.819501319172,-108.928013630747,
483.537703348572));
#270751=CARTESIAN_POINT('Ctrl Pts',(-79.8974404698481,-102.639948694851,
481.537703348572));
#270752=CARTESIAN_POINT('Ctrl Pts',(-87.9753796205242,-96.351883758956,
479.537703348572));
#270753=CARTESIAN_POINT('Ctrl Pts',(-94.9701958612989,-88.8775672472035,
477.537703348572));
#270754=CARTESIAN_POINT('Ctrl Pts',(-101.965012102074,-81.403250735451,
475.537703348572));
#270755=CARTESIAN_POINT('Ctrl Pts',(-107.704469842635,-72.9267251261949,
473.537703348572));
#270756=CARTESIAN_POINT('Ctrl Pts',(-113.443927583196,-64.4501995169389,
471.537703348572));
#270757=CARTESIAN_POINT('Ctrl Pts',(-117.786702325803,-55.1801850026549,
469.537703348572));
#270758=CARTESIAN_POINT('Ctrl Pts',(-122.129477068411,-45.910170488371,
467.537703348572));
#270759=CARTESIAN_POINT('Ctrl Pts',(-124.968635286058,-36.074925591815,
465.537703348572));
#270760=CARTESIAN_POINT('Ctrl Pts',(-127.807793503704,-26.239680695259,
463.537703348572));
#270761=CARTESIAN_POINT('Ctrl Pts',(-129.073425698447,-16.0813817870907,
461.537703348572));
#270762=CARTESIAN_POINT('Ctrl Pts',(-130.339057893189,-5.92308287892235,
459.537703348572));
#270763=CARTESIAN_POINT('Ctrl Pts',(-130.,4.30813900827805,457.537703348572));
#270764=CARTESIAN_POINT('Ctrl Pts',(-129.660942106811,14.5393608954784,
455.537703348572));
#270765=CARTESIAN_POINT('Ctrl Pts',(-127.725542856289,24.5915791233693,
453.537703348572));
#270766=CARTESIAN_POINT('Ctrl Pts',(-125.790143605767,34.6437973512602,
451.537703348572));
#270767=CARTESIAN_POINT('Ctrl Pts',(-122.306058950682,44.2694929456713,
449.537703348572));
#270768=CARTESIAN_POINT('Ctrl Pts',(-118.821974295598,53.8951885400825,
447.537703348572));
#270769=CARTESIAN_POINT('Ctrl Pts',(-113.874993963172,62.8573449296272,
445.537703348572));
#270770=CARTESIAN_POINT('Ctrl Pts',(-108.928013630747,71.819501319172,443.537703348572));
#270771=CARTESIAN_POINT('Ctrl Pts',(-102.639948694851,79.8974404698481,
441.537703348572));
#270772=CARTESIAN_POINT('Ctrl Pts',(-96.3518837589561,87.9753796205242,
439.537703348572));
#270773=CARTESIAN_POINT('Ctrl Pts',(-88.8775672472035,94.9701958612989,
437.537703348572));
#270774=CARTESIAN_POINT('Ctrl Pts',(-81.403250735451,101.965012102074,435.537703348572));
#270775=CARTESIAN_POINT('Ctrl Pts',(-72.9267251261949,107.704469842635,
433.537703348572));
#270776=CARTESIAN_POINT('Ctrl Pts',(-64.4501995169389,113.443927583196,
431.537703348572));
#270777=CARTESIAN_POINT('Ctrl Pts',(-55.1801850026549,117.786702325803,
429.537703348572));
#270778=CARTESIAN_POINT('Ctrl Pts',(-45.910170488371,122.129477068411,427.537703348572));
#270779=CARTESIAN_POINT('Ctrl Pts',(-36.074925591815,124.968635286058,425.537703348572));
#270780=CARTESIAN_POINT('Ctrl Pts',(-26.239680695259,127.807793503704,423.537703348572));
#270781=CARTESIAN_POINT('Ctrl Pts',(-16.0813817870907,129.073425698447,
421.537703348572));
#270782=CARTESIAN_POINT('Ctrl Pts',(-5.92308287892242,130.339057893189,
419.537703348572));
#270783=CARTESIAN_POINT('Ctrl Pts',(4.30813900827804,130.,417.537703348572));
#270784=CARTESIAN_POINT('Ctrl Pts',(14.5393608954785,129.660942106811,415.537703348572));
#270785=CARTESIAN_POINT('Ctrl Pts',(24.5915791233693,127.725542856289,413.537703348572));
#270786=CARTESIAN_POINT('Ctrl Pts',(34.6437973512602,125.790143605767,411.537703348572));
#270787=CARTESIAN_POINT('Ctrl Pts',(44.2694929456713,122.306058950682,409.537703348572));
#270788=CARTESIAN_POINT('Ctrl Pts',(53.8951885400825,118.821974295598,407.537703348572));
#270789=CARTESIAN_POINT('Ctrl Pts',(62.8573449296272,113.874993963172,405.537703348572));
#270790=CARTESIAN_POINT('Ctrl Pts',(71.819501319172,108.928013630747,403.537703348572));
#270791=CARTESIAN_POINT('Ctrl Pts',(79.8974404698481,102.639948694851,401.537703348572));
#270792=CARTESIAN_POINT('Ctrl Pts',(87.9753796205242,96.351883758956,399.537703348572));
#270793=CARTESIAN_POINT('Ctrl Pts',(94.9701958612989,88.8775672472035,397.537703348572));
#270794=CARTESIAN_POINT('Ctrl Pts',(101.965012102074,81.403250735451,395.537703348572));
#270795=CARTESIAN_POINT('Ctrl Pts',(107.704469842635,72.926725126195,393.537703348572));
#270796=CARTESIAN_POINT('Ctrl Pts',(113.443927583196,64.4501995169389,391.537703348572));
#270797=CARTESIAN_POINT('Ctrl Pts',(117.786702325803,55.1801850026549,389.537703348572));
#270798=CARTESIAN_POINT('Ctrl Pts',(122.129477068411,45.910170488371,387.537703348572));
#270799=CARTESIAN_POINT('Ctrl Pts',(124.968635286058,36.074925591815,385.537703348572));
#270800=CARTESIAN_POINT('Ctrl Pts',(127.807793503704,26.239680695259,383.537703348572));
#270801=CARTESIAN_POINT('Ctrl Pts',(129.073425698447,16.0813817870907,381.537703348572));
#270802=CARTESIAN_POINT('Ctrl Pts',(130.339057893189,5.92308287892242,379.537703348572));
#270803=CARTESIAN_POINT('Ctrl Pts',(130.,-4.30813900827807,377.537703348572));
#270804=CARTESIAN_POINT('Ctrl Pts',(130.,4.30813900827812,532.462296651428));
#270805=CARTESIAN_POINT('Ctrl Pts',(130.339057893189,-5.92308287892228,
530.462296651428));
#270806=CARTESIAN_POINT('Ctrl Pts',(129.073425698447,-16.0813817870906,
528.462296651428));
#270807=CARTESIAN_POINT('Ctrl Pts',(127.807793503704,-26.2396806952589,
526.462296651428));
#270808=CARTESIAN_POINT('Ctrl Pts',(124.968635286058,-36.0749255918149,
524.462296651428));
#270809=CARTESIAN_POINT('Ctrl Pts',(122.129477068411,-45.9101704883709,
522.462296651428));
#270810=CARTESIAN_POINT('Ctrl Pts',(117.786702325803,-55.1801850026549,
520.462296651428));
#270811=CARTESIAN_POINT('Ctrl Pts',(113.443927583196,-64.4501995169389,
518.462296651428));
#270812=CARTESIAN_POINT('Ctrl Pts',(107.704469842635,-72.9267251261949,
516.462296651428));
#270813=CARTESIAN_POINT('Ctrl Pts',(101.965012102074,-81.4032507354509,
514.462296651428));
#270814=CARTESIAN_POINT('Ctrl Pts',(94.9701958612989,-88.8775672472035,
512.462296651428));
#270815=CARTESIAN_POINT('Ctrl Pts',(87.9753796205242,-96.351883758956,510.462296651428));
#270816=CARTESIAN_POINT('Ctrl Pts',(79.8974404698481,-102.639948694851,
508.462296651428));
#270817=CARTESIAN_POINT('Ctrl Pts',(71.8195013191721,-108.928013630747,
506.462296651428));
#270818=CARTESIAN_POINT('Ctrl Pts',(62.8573449296273,-113.874993963172,
504.462296651428));
#270819=CARTESIAN_POINT('Ctrl Pts',(53.8951885400825,-118.821974295598,
502.462296651428));
#270820=CARTESIAN_POINT('Ctrl Pts',(44.2694929456714,-122.306058950682,
500.462296651428));
#270821=CARTESIAN_POINT('Ctrl Pts',(34.6437973512603,-125.790143605767,
498.462296651428));
#270822=CARTESIAN_POINT('Ctrl Pts',(24.5915791233694,-127.725542856289,
496.462296651428));
#270823=CARTESIAN_POINT('Ctrl Pts',(14.5393608954785,-129.660942106811,
494.462296651428));
#270824=CARTESIAN_POINT('Ctrl Pts',(4.30813900827813,-130.,492.462296651428));
#270825=CARTESIAN_POINT('Ctrl Pts',(-5.92308287892227,-130.339057893189,
490.462296651428));
#270826=CARTESIAN_POINT('Ctrl Pts',(-16.0813817870906,-129.073425698447,
488.462296651428));
#270827=CARTESIAN_POINT('Ctrl Pts',(-26.2396806952589,-127.807793503705,
486.462296651428));
#270828=CARTESIAN_POINT('Ctrl Pts',(-36.0749255918149,-124.968635286058,
484.462296651428));
#270829=CARTESIAN_POINT('Ctrl Pts',(-45.9101704883709,-122.129477068411,
482.462296651428));
#270830=CARTESIAN_POINT('Ctrl Pts',(-55.1801850026549,-117.786702325803,
480.462296651428));
#270831=CARTESIAN_POINT('Ctrl Pts',(-64.4501995169389,-113.443927583196,
478.462296651428));
#270832=CARTESIAN_POINT('Ctrl Pts',(-72.9267251261949,-107.704469842635,
476.462296651428));
#270833=CARTESIAN_POINT('Ctrl Pts',(-81.4032507354509,-101.965012102074,
474.462296651428));
#270834=CARTESIAN_POINT('Ctrl Pts',(-88.8775672472034,-94.9701958612989,
472.462296651428));
#270835=CARTESIAN_POINT('Ctrl Pts',(-96.351883758956,-87.9753796205242,
470.462296651428));
#270836=CARTESIAN_POINT('Ctrl Pts',(-102.639948694851,-79.8974404698482,
468.462296651428));
#270837=CARTESIAN_POINT('Ctrl Pts',(-108.928013630747,-71.8195013191721,
466.462296651428));
#270838=CARTESIAN_POINT('Ctrl Pts',(-113.874993963172,-62.8573449296273,
464.462296651428));
#270839=CARTESIAN_POINT('Ctrl Pts',(-118.821974295598,-53.8951885400825,
462.462296651428));
#270840=CARTESIAN_POINT('Ctrl Pts',(-122.306058950682,-44.2694929456714,
460.462296651428));
#270841=CARTESIAN_POINT('Ctrl Pts',(-125.790143605767,-34.6437973512603,
458.462296651428));
#270842=CARTESIAN_POINT('Ctrl Pts',(-127.725542856289,-24.5915791233694,
456.462296651428));
#270843=CARTESIAN_POINT('Ctrl Pts',(-129.660942106811,-14.5393608954785,
454.462296651429));
#270844=CARTESIAN_POINT('Ctrl Pts',(-130.,-4.30813900827813,452.462296651428));
#270845=CARTESIAN_POINT('Ctrl Pts',(-130.339057893189,5.92308287892227,
450.462296651428));
#270846=CARTESIAN_POINT('Ctrl Pts',(-129.073425698447,16.0813817870906,
448.462296651428));
#270847=CARTESIAN_POINT('Ctrl Pts',(-127.807793503705,26.2396806952589,
446.462296651428));
#270848=CARTESIAN_POINT('Ctrl Pts',(-124.968635286058,36.0749255918149,
444.462296651428));
#270849=CARTESIAN_POINT('Ctrl Pts',(-122.129477068411,45.9101704883709,
442.462296651428));
#270850=CARTESIAN_POINT('Ctrl Pts',(-117.786702325803,55.1801850026549,
440.462296651428));
#270851=CARTESIAN_POINT('Ctrl Pts',(-113.443927583196,64.4501995169388,
438.462296651428));
#270852=CARTESIAN_POINT('Ctrl Pts',(-107.704469842635,72.9267251261949,
436.462296651428));
#270853=CARTESIAN_POINT('Ctrl Pts',(-101.965012102074,81.4032507354509,
434.462296651428));
#270854=CARTESIAN_POINT('Ctrl Pts',(-94.9701958612989,88.8775672472034,
432.462296651428));
#270855=CARTESIAN_POINT('Ctrl Pts',(-87.9753796205243,96.3518837589559,
430.462296651428));
#270856=CARTESIAN_POINT('Ctrl Pts',(-79.8974404698482,102.639948694851,
428.462296651428));
#270857=CARTESIAN_POINT('Ctrl Pts',(-71.819501319172,108.928013630747,426.462296651428));
#270858=CARTESIAN_POINT('Ctrl Pts',(-62.8573449296273,113.874993963172,
424.462296651428));
#270859=CARTESIAN_POINT('Ctrl Pts',(-53.8951885400826,118.821974295598,
422.462296651428));
#270860=CARTESIAN_POINT('Ctrl Pts',(-44.2694929456714,122.306058950682,
420.462296651428));
#270861=CARTESIAN_POINT('Ctrl Pts',(-34.6437973512603,125.790143605767,
418.462296651428));
#270862=CARTESIAN_POINT('Ctrl Pts',(-24.5915791233694,127.725542856289,
416.462296651428));
#270863=CARTESIAN_POINT('Ctrl Pts',(-14.5393608954786,129.660942106811,
414.462296651428));
#270864=CARTESIAN_POINT('Ctrl Pts',(-4.30813900827814,130.,412.462296651428));
#270865=CARTESIAN_POINT('Ctrl Pts',(5.92308287892232,130.339057893189,410.462296651428));
#270866=CARTESIAN_POINT('Ctrl Pts',(16.0813817870906,129.073425698447,408.462296651428));
#270867=CARTESIAN_POINT('Ctrl Pts',(26.2396806952589,127.807793503705,406.462296651428));
#270868=CARTESIAN_POINT('Ctrl Pts',(36.0749255918149,124.968635286058,404.462296651428));
#270869=CARTESIAN_POINT('Ctrl Pts',(45.9101704883709,122.129477068411,402.462296651428));
#270870=CARTESIAN_POINT('Ctrl Pts',(55.1801850026549,117.786702325803,400.462296651428));
#270871=CARTESIAN_POINT('Ctrl Pts',(64.4501995169388,113.443927583196,398.462296651428));
#270872=CARTESIAN_POINT('Ctrl Pts',(72.9267251261949,107.704469842635,396.462296651428));
#270873=CARTESIAN_POINT('Ctrl Pts',(81.4032507354509,101.965012102074,394.462296651428));
#270874=CARTESIAN_POINT('Ctrl Pts',(88.8775672472034,94.9701958612989,392.462296651428));
#270875=CARTESIAN_POINT('Ctrl Pts',(96.3518837589559,87.9753796205243,390.462296651428));
#270876=CARTESIAN_POINT('Ctrl Pts',(102.639948694851,79.8974404698482,388.462296651428));
#270877=CARTESIAN_POINT('Ctrl Pts',(108.928013630747,71.819501319172,386.462296651428));
#270878=CARTESIAN_POINT('Ctrl Pts',(113.874993963172,62.8573449296273,384.462296651428));
#270879=CARTESIAN_POINT('Ctrl Pts',(118.821974295598,53.8951885400826,382.462296651428));
#270880=CARTESIAN_POINT('Ctrl Pts',(122.306058950682,44.2694929456714,380.462296651428));
#270881=CARTESIAN_POINT('Ctrl Pts',(125.790143605767,34.6437973512603,378.462296651428));
#270882=CARTESIAN_POINT('Ctrl Pts',(127.725542856289,24.5915791233694,376.462296651428));
#270883=CARTESIAN_POINT('Ctrl Pts',(129.660942106811,14.5393608954786,374.462296651428));
#270884=CARTESIAN_POINT('Ctrl Pts',(130.,4.30813900827812,372.462296651428));
#270885=CARTESIAN_POINT('Ctrl Pts',(129.934615416877,-5.96286660784692,
530.450909781393));
#270886=CARTESIAN_POINT('Ctrl Pts',(129.701667605591,-11.0389459941987,
529.455068342531));
#270887=CARTESIAN_POINT('Ctrl Pts',(129.073425698447,-16.0813817870906,
528.462296651428));
#270888=CARTESIAN_POINT('Ctrl Pts',(127.807793503704,-26.2396806952589,
526.462296651428));
#270889=CARTESIAN_POINT('Ctrl Pts',(124.968635286058,-36.0749255918149,
524.462296651428));
#270890=CARTESIAN_POINT('Ctrl Pts',(122.129477068411,-45.9101704883709,
522.462296651428));
#270891=CARTESIAN_POINT('Ctrl Pts',(117.786702325803,-55.1801850026549,
520.462296651428));
#270892=CARTESIAN_POINT('Ctrl Pts',(113.443927583196,-64.4501995169389,
518.462296651428));
#270893=CARTESIAN_POINT('Ctrl Pts',(107.704469842635,-72.9267251261949,
516.462296651428));
#270894=CARTESIAN_POINT('Ctrl Pts',(101.965012102074,-81.4032507354509,
514.462296651428));
#270895=CARTESIAN_POINT('Ctrl Pts',(94.9701958612989,-88.8775672472035,
512.462296651428));
#270896=CARTESIAN_POINT('Ctrl Pts',(87.9753796205242,-96.351883758956,510.462296651428));
#270897=CARTESIAN_POINT('Ctrl Pts',(79.8974404698481,-102.639948694851,
508.462296651428));
#270898=CARTESIAN_POINT('Ctrl Pts',(71.8195013191721,-108.928013630747,
506.462296651428));
#270899=CARTESIAN_POINT('Ctrl Pts',(62.8573449296273,-113.874993963172,
504.462296651428));
#270900=CARTESIAN_POINT('Ctrl Pts',(53.8951885400825,-118.821974295598,
502.462296651428));
#270901=CARTESIAN_POINT('Ctrl Pts',(44.2694929456714,-122.306058950682,
500.462296651428));
#270902=CARTESIAN_POINT('Ctrl Pts',(34.6437973512603,-125.790143605767,
498.462296651428));
#270903=CARTESIAN_POINT('Ctrl Pts',(24.5915791233694,-127.725542856289,
496.462296651428));
#270904=CARTESIAN_POINT('Ctrl Pts',(14.5393608954785,-129.660942106811,
494.462296651428));
#270905=CARTESIAN_POINT('Ctrl Pts',(4.30813900827813,-130.,492.462296651428));
#270906=CARTESIAN_POINT('Ctrl Pts',(-5.92308287892227,-130.339057893189,
490.462296651428));
#270907=CARTESIAN_POINT('Ctrl Pts',(-16.0813817870906,-129.073425698447,
488.462296651428));
#270908=CARTESIAN_POINT('Ctrl Pts',(-26.2396806952589,-127.807793503705,
486.462296651428));
#270909=CARTESIAN_POINT('Ctrl Pts',(-36.0749255918149,-124.968635286058,
484.462296651428));
#270910=CARTESIAN_POINT('Ctrl Pts',(-45.9101704883709,-122.129477068411,
482.462296651428));
#270911=CARTESIAN_POINT('Ctrl Pts',(-55.1801850026549,-117.786702325803,
480.462296651428));
#270912=CARTESIAN_POINT('Ctrl Pts',(-64.4501995169389,-113.443927583196,
478.462296651428));
#270913=CARTESIAN_POINT('Ctrl Pts',(-72.9267251261949,-107.704469842635,
476.462296651428));
#270914=CARTESIAN_POINT('Ctrl Pts',(-81.4032507354509,-101.965012102074,
474.462296651428));
#270915=CARTESIAN_POINT('Ctrl Pts',(-88.8775672472034,-94.9701958612989,
472.462296651428));
#270916=CARTESIAN_POINT('Ctrl Pts',(-96.351883758956,-87.9753796205242,
470.462296651428));
#270917=CARTESIAN_POINT('Ctrl Pts',(-102.639948694851,-79.8974404698482,
468.462296651428));
#270918=CARTESIAN_POINT('Ctrl Pts',(-108.928013630747,-71.8195013191721,
466.462296651428));
#270919=CARTESIAN_POINT('Ctrl Pts',(-113.874993963172,-62.8573449296273,
464.462296651428));
#270920=CARTESIAN_POINT('Ctrl Pts',(-118.821974295598,-53.8951885400825,
462.462296651428));
#270921=CARTESIAN_POINT('Ctrl Pts',(-122.306058950682,-44.2694929456714,
460.462296651428));
#270922=CARTESIAN_POINT('Ctrl Pts',(-125.790143605767,-34.6437973512603,
458.462296651428));
#270923=CARTESIAN_POINT('Ctrl Pts',(-127.725542856289,-24.5915791233694,
456.462296651428));
#270924=CARTESIAN_POINT('Ctrl Pts',(-129.660942106811,-14.5393608954785,
454.462296651429));
#270925=CARTESIAN_POINT('Ctrl Pts',(-130.,-4.30813900827813,452.462296651428));
#270926=CARTESIAN_POINT('Ctrl Pts',(-130.339057893189,5.92308287892227,
450.462296651428));
#270927=CARTESIAN_POINT('Ctrl Pts',(-129.073425698447,16.0813817870906,
448.462296651428));
#270928=CARTESIAN_POINT('Ctrl Pts',(-127.807793503705,26.2396806952589,
446.462296651428));
#270929=CARTESIAN_POINT('Ctrl Pts',(-124.968635286058,36.0749255918149,
444.462296651428));
#270930=CARTESIAN_POINT('Ctrl Pts',(-122.129477068411,45.9101704883709,
442.462296651428));
#270931=CARTESIAN_POINT('Ctrl Pts',(-117.786702325803,55.1801850026549,
440.462296651428));
#270932=CARTESIAN_POINT('Ctrl Pts',(-113.443927583196,64.4501995169388,
438.462296651428));
#270933=CARTESIAN_POINT('Ctrl Pts',(-107.704469842635,72.9267251261949,
436.462296651428));
#270934=CARTESIAN_POINT('Ctrl Pts',(-101.965012102074,81.4032507354509,
434.462296651428));
#270935=CARTESIAN_POINT('Ctrl Pts',(-94.9701958612989,88.8775672472034,
432.462296651428));
#270936=CARTESIAN_POINT('Ctrl Pts',(-87.9753796205243,96.3518837589559,
430.462296651428));
#270937=CARTESIAN_POINT('Ctrl Pts',(-79.8974404698482,102.639948694851,
428.462296651428));
#270938=CARTESIAN_POINT('Ctrl Pts',(-71.819501319172,108.928013630747,426.462296651428));
#270939=CARTESIAN_POINT('Ctrl Pts',(-62.8573449296273,113.874993963172,
424.462296651428));
#270940=CARTESIAN_POINT('Ctrl Pts',(-53.8951885400826,118.821974295598,
422.462296651428));
#270941=CARTESIAN_POINT('Ctrl Pts',(-44.2694929456714,122.306058950682,
420.462296651428));
#270942=CARTESIAN_POINT('Ctrl Pts',(-34.6437973512603,125.790143605767,
418.462296651428));
#270943=CARTESIAN_POINT('Ctrl Pts',(-24.5915791233694,127.725542856289,
416.462296651428));
#270944=CARTESIAN_POINT('Ctrl Pts',(-14.5393608954786,129.660942106811,
414.462296651428));
#270945=CARTESIAN_POINT('Ctrl Pts',(-4.30813900827814,130.,412.462296651428));
#270946=CARTESIAN_POINT('Ctrl Pts',(5.92308287892232,130.339057893189,410.462296651428));
#270947=CARTESIAN_POINT('Ctrl Pts',(16.0813817870906,129.073425698447,408.462296651428));
#270948=CARTESIAN_POINT('Ctrl Pts',(26.2396806952589,127.807793503705,406.462296651428));
#270949=CARTESIAN_POINT('Ctrl Pts',(36.0749255918149,124.968635286058,404.462296651428));
#270950=CARTESIAN_POINT('Ctrl Pts',(45.9101704883709,122.129477068411,402.462296651428));
#270951=CARTESIAN_POINT('Ctrl Pts',(55.1801850026549,117.786702325803,400.462296651428));
#270952=CARTESIAN_POINT('Ctrl Pts',(64.4501995169388,113.443927583196,398.462296651428));
#270953=CARTESIAN_POINT('Ctrl Pts',(72.9267251261949,107.704469842635,396.462296651428));
#270954=CARTESIAN_POINT('Ctrl Pts',(81.403250735451,101.965012102074,394.462296651428));
#270955=CARTESIAN_POINT('Ctrl Pts',(88.8775672472034,94.9701958612989,392.462296651428));
#270956=CARTESIAN_POINT('Ctrl Pts',(96.3518837589559,87.9753796205243,390.462296651428));
#270957=CARTESIAN_POINT('Ctrl Pts',(102.639948694851,79.8974404698482,388.462296651428));
#270958=CARTESIAN_POINT('Ctrl Pts',(108.928013630747,71.8195013191721,386.462296651428));
#270959=CARTESIAN_POINT('Ctrl Pts',(113.874993963172,62.8573449296273,384.462296651428));
#270960=CARTESIAN_POINT('Ctrl Pts',(118.821974295598,53.8951885400826,382.462296651428));
#270961=CARTESIAN_POINT('Ctrl Pts',(122.306058950682,44.2694929456714,380.462296651428));
#270962=CARTESIAN_POINT('Ctrl Pts',(125.790143605767,34.6437973512603,378.462296651428));
#270963=CARTESIAN_POINT('Ctrl Pts',(127.725542856289,24.5915791233694,376.462296651428));
#270964=CARTESIAN_POINT('Ctrl Pts',(129.382196958681,15.9871278397994,374.750345898171));
#270965=CARTESIAN_POINT('Ctrl Pts',(129.869812400585,7.23822414350007,373.035792462989));
#270966=CARTESIAN_POINT('Ctrl Pts',(129.869812400585,-7.23822414349995,
536.964207537012));
#270967=CARTESIAN_POINT('Ctrl Pts',(129.382196958681,-15.9871278397992,
535.249654101829));
#270968=CARTESIAN_POINT('Ctrl Pts',(127.725542856289,-24.5915791233694,
533.537703348572));
#270969=CARTESIAN_POINT('Ctrl Pts',(125.790143605767,-34.6437973512603,
531.537703348572));
#270970=CARTESIAN_POINT('Ctrl Pts',(122.306058950682,-44.2694929456714,
529.537703348572));
#270971=CARTESIAN_POINT('Ctrl Pts',(118.821974295598,-53.8951885400825,
527.537703348572));
#270972=CARTESIAN_POINT('Ctrl Pts',(113.874993963172,-62.8573449296272,
525.537703348572));
#270973=CARTESIAN_POINT('Ctrl Pts',(108.928013630747,-71.819501319172,523.537703348572));
#270974=CARTESIAN_POINT('Ctrl Pts',(102.639948694851,-79.8974404698481,
521.537703348572));
#270975=CARTESIAN_POINT('Ctrl Pts',(96.351883758956,-87.9753796205242,519.537703348572));
#270976=CARTESIAN_POINT('Ctrl Pts',(88.8775672472035,-94.9701958612989,
517.537703348572));
#270977=CARTESIAN_POINT('Ctrl Pts',(81.403250735451,-101.965012102074,515.537703348572));
#270978=CARTESIAN_POINT('Ctrl Pts',(72.9267251261949,-107.704469842635,
513.537703348572));
#270979=CARTESIAN_POINT('Ctrl Pts',(64.4501995169389,-113.443927583196,
511.537703348572));
#270980=CARTESIAN_POINT('Ctrl Pts',(55.1801850026549,-117.786702325803,
509.537703348572));
#270981=CARTESIAN_POINT('Ctrl Pts',(45.910170488371,-122.129477068411,507.537703348572));
#270982=CARTESIAN_POINT('Ctrl Pts',(36.074925591815,-124.968635286058,505.537703348572));
#270983=CARTESIAN_POINT('Ctrl Pts',(26.239680695259,-127.807793503704,503.537703348572));
#270984=CARTESIAN_POINT('Ctrl Pts',(16.0813817870907,-129.073425698447,
501.537703348572));
#270985=CARTESIAN_POINT('Ctrl Pts',(5.92308287892234,-130.339057893189,
499.537703348572));
#270986=CARTESIAN_POINT('Ctrl Pts',(-4.30813900827806,-130.,497.537703348572));
#270987=CARTESIAN_POINT('Ctrl Pts',(-14.5393608954785,-129.660942106811,
495.537703348572));
#270988=CARTESIAN_POINT('Ctrl Pts',(-24.5915791233694,-127.725542856289,
493.537703348572));
#270989=CARTESIAN_POINT('Ctrl Pts',(-34.6437973512602,-125.790143605767,
491.537703348572));
#270990=CARTESIAN_POINT('Ctrl Pts',(-44.2694929456713,-122.306058950682,
489.537703348572));
#270991=CARTESIAN_POINT('Ctrl Pts',(-53.8951885400825,-118.821974295598,
487.537703348572));
#270992=CARTESIAN_POINT('Ctrl Pts',(-62.8573449296272,-113.874993963172,
485.537703348572));
#270993=CARTESIAN_POINT('Ctrl Pts',(-71.819501319172,-108.928013630747,
483.537703348572));
#270994=CARTESIAN_POINT('Ctrl Pts',(-79.8974404698481,-102.639948694851,
481.537703348572));
#270995=CARTESIAN_POINT('Ctrl Pts',(-87.9753796205242,-96.351883758956,
479.537703348572));
#270996=CARTESIAN_POINT('Ctrl Pts',(-94.9701958612989,-88.8775672472035,
477.537703348572));
#270997=CARTESIAN_POINT('Ctrl Pts',(-101.965012102074,-81.403250735451,
475.537703348572));
#270998=CARTESIAN_POINT('Ctrl Pts',(-107.704469842635,-72.9267251261949,
473.537703348572));
#270999=CARTESIAN_POINT('Ctrl Pts',(-113.443927583196,-64.4501995169389,
471.537703348572));
#271000=CARTESIAN_POINT('Ctrl Pts',(-117.786702325803,-55.1801850026549,
469.537703348572));
#271001=CARTESIAN_POINT('Ctrl Pts',(-122.129477068411,-45.910170488371,
467.537703348572));
#271002=CARTESIAN_POINT('Ctrl Pts',(-124.968635286058,-36.074925591815,
465.537703348572));
#271003=CARTESIAN_POINT('Ctrl Pts',(-127.807793503704,-26.239680695259,
463.537703348572));
#271004=CARTESIAN_POINT('Ctrl Pts',(-129.073425698447,-16.0813817870907,
461.537703348572));
#271005=CARTESIAN_POINT('Ctrl Pts',(-130.339057893189,-5.92308287892235,
459.537703348572));
#271006=CARTESIAN_POINT('Ctrl Pts',(-130.,4.30813900827805,457.537703348572));
#271007=CARTESIAN_POINT('Ctrl Pts',(-129.660942106811,14.5393608954784,
455.537703348572));
#271008=CARTESIAN_POINT('Ctrl Pts',(-127.725542856289,24.5915791233693,
453.537703348572));
#271009=CARTESIAN_POINT('Ctrl Pts',(-125.790143605767,34.6437973512602,
451.537703348572));
#271010=CARTESIAN_POINT('Ctrl Pts',(-122.306058950682,44.2694929456713,
449.537703348572));
#271011=CARTESIAN_POINT('Ctrl Pts',(-118.821974295598,53.8951885400825,
447.537703348572));
#271012=CARTESIAN_POINT('Ctrl Pts',(-113.874993963172,62.8573449296272,
445.537703348572));
#271013=CARTESIAN_POINT('Ctrl Pts',(-108.928013630747,71.819501319172,443.537703348572));
#271014=CARTESIAN_POINT('Ctrl Pts',(-102.639948694851,79.8974404698481,
441.537703348572));
#271015=CARTESIAN_POINT('Ctrl Pts',(-96.3518837589561,87.9753796205242,
439.537703348572));
#271016=CARTESIAN_POINT('Ctrl Pts',(-88.8775672472035,94.9701958612989,
437.537703348572));
#271017=CARTESIAN_POINT('Ctrl Pts',(-81.403250735451,101.965012102074,435.537703348572));
#271018=CARTESIAN_POINT('Ctrl Pts',(-72.9267251261949,107.704469842635,
433.537703348572));
#271019=CARTESIAN_POINT('Ctrl Pts',(-64.4501995169389,113.443927583196,
431.537703348572));
#271020=CARTESIAN_POINT('Ctrl Pts',(-55.1801850026549,117.786702325803,
429.537703348572));
#271021=CARTESIAN_POINT('Ctrl Pts',(-45.910170488371,122.129477068411,427.537703348572));
#271022=CARTESIAN_POINT('Ctrl Pts',(-36.074925591815,124.968635286058,425.537703348572));
#271023=CARTESIAN_POINT('Ctrl Pts',(-26.239680695259,127.807793503704,423.537703348572));
#271024=CARTESIAN_POINT('Ctrl Pts',(-16.0813817870907,129.073425698447,
421.537703348572));
#271025=CARTESIAN_POINT('Ctrl Pts',(-5.92308287892242,130.339057893189,
419.537703348572));
#271026=CARTESIAN_POINT('Ctrl Pts',(4.30813900827804,130.,417.537703348572));
#271027=CARTESIAN_POINT('Ctrl Pts',(14.5393608954785,129.660942106811,415.537703348572));
#271028=CARTESIAN_POINT('Ctrl Pts',(24.5915791233693,127.725542856289,413.537703348572));
#271029=CARTESIAN_POINT('Ctrl Pts',(34.6437973512602,125.790143605767,411.537703348572));
#271030=CARTESIAN_POINT('Ctrl Pts',(44.2694929456713,122.306058950682,409.537703348572));
#271031=CARTESIAN_POINT('Ctrl Pts',(53.8951885400825,118.821974295598,407.537703348572));
#271032=CARTESIAN_POINT('Ctrl Pts',(62.8573449296272,113.874993963172,405.537703348572));
#271033=CARTESIAN_POINT('Ctrl Pts',(71.819501319172,108.928013630747,403.537703348572));
#271034=CARTESIAN_POINT('Ctrl Pts',(79.8974404698481,102.639948694851,401.537703348572));
#271035=CARTESIAN_POINT('Ctrl Pts',(87.9753796205242,96.351883758956,399.537703348572));
#271036=CARTESIAN_POINT('Ctrl Pts',(94.9701958612989,88.8775672472035,397.537703348572));
#271037=CARTESIAN_POINT('Ctrl Pts',(101.965012102074,81.403250735451,395.537703348572));
#271038=CARTESIAN_POINT('Ctrl Pts',(107.704469842635,72.926725126195,393.537703348572));
#271039=CARTESIAN_POINT('Ctrl Pts',(113.443927583196,64.4501995169389,391.537703348572));
#271040=CARTESIAN_POINT('Ctrl Pts',(117.786702325803,55.1801850026549,389.537703348572));
#271041=CARTESIAN_POINT('Ctrl Pts',(122.129477068411,45.910170488371,387.537703348572));
#271042=CARTESIAN_POINT('Ctrl Pts',(124.968635286058,36.074925591815,385.537703348572));
#271043=CARTESIAN_POINT('Ctrl Pts',(127.807793503704,26.239680695259,383.537703348572));
#271044=CARTESIAN_POINT('Ctrl Pts',(129.073425698447,16.0813817870907,381.537703348572));
#271045=CARTESIAN_POINT('Ctrl Pts',(129.701667605591,11.0389459941988,380.54493165747));
#271046=CARTESIAN_POINT('Ctrl Pts',(129.934615416877,5.96286660784696,379.549090218607));
#271047=CARTESIAN_POINT('Ctrl Pts',(130.,4.30813900827812,532.462296651428));
#271048=CARTESIAN_POINT('Ctrl Pts',(130.339057893189,-5.92308287892228,
530.462296651428));
#271049=CARTESIAN_POINT('Ctrl Pts',(129.073425698447,-16.0813817870906,
528.462296651428));
#271050=CARTESIAN_POINT('Ctrl Pts',(127.807793503704,-26.2396806952589,
526.462296651428));
#271051=CARTESIAN_POINT('Ctrl Pts',(124.968635286058,-36.0749255918149,
524.462296651428));
#271052=CARTESIAN_POINT('Ctrl Pts',(122.129477068411,-45.9101704883709,
522.462296651428));
#271053=CARTESIAN_POINT('Ctrl Pts',(117.786702325803,-55.1801850026549,
520.462296651428));
#271054=CARTESIAN_POINT('Ctrl Pts',(113.443927583196,-64.4501995169389,
518.462296651428));
#271055=CARTESIAN_POINT('Ctrl Pts',(107.704469842635,-72.9267251261949,
516.462296651428));
#271056=CARTESIAN_POINT('Ctrl Pts',(101.965012102074,-81.4032507354509,
514.462296651428));
#271057=CARTESIAN_POINT('Ctrl Pts',(94.9701958612989,-88.8775672472035,
512.462296651428));
#271058=CARTESIAN_POINT('Ctrl Pts',(87.9753796205242,-96.351883758956,510.462296651428));
#271059=CARTESIAN_POINT('Ctrl Pts',(79.8974404698481,-102.639948694851,
508.462296651428));
#271060=CARTESIAN_POINT('Ctrl Pts',(71.8195013191721,-108.928013630747,
506.462296651428));
#271061=CARTESIAN_POINT('Ctrl Pts',(62.8573449296273,-113.874993963172,
504.462296651428));
#271062=CARTESIAN_POINT('Ctrl Pts',(53.8951885400825,-118.821974295598,
502.462296651428));
#271063=CARTESIAN_POINT('Ctrl Pts',(44.2694929456714,-122.306058950682,
500.462296651428));
#271064=CARTESIAN_POINT('Ctrl Pts',(34.6437973512603,-125.790143605767,
498.462296651428));
#271065=CARTESIAN_POINT('Ctrl Pts',(24.5915791233694,-127.725542856289,
496.462296651428));
#271066=CARTESIAN_POINT('Ctrl Pts',(14.5393608954785,-129.660942106811,
494.462296651428));
#271067=CARTESIAN_POINT('Ctrl Pts',(4.30813900827813,-130.,492.462296651428));
#271068=CARTESIAN_POINT('Ctrl Pts',(-5.92308287892227,-130.339057893189,
490.462296651428));
#271069=CARTESIAN_POINT('Ctrl Pts',(-16.0813817870906,-129.073425698447,
488.462296651428));
#271070=CARTESIAN_POINT('Ctrl Pts',(-26.2396806952589,-127.807793503705,
486.462296651428));
#271071=CARTESIAN_POINT('Ctrl Pts',(-36.0749255918149,-124.968635286058,
484.462296651428));
#271072=CARTESIAN_POINT('Ctrl Pts',(-45.9101704883709,-122.129477068411,
482.462296651428));
#271073=CARTESIAN_POINT('Ctrl Pts',(-55.1801850026549,-117.786702325803,
480.462296651428));
#271074=CARTESIAN_POINT('Ctrl Pts',(-64.4501995169389,-113.443927583196,
478.462296651428));
#271075=CARTESIAN_POINT('Ctrl Pts',(-72.9267251261949,-107.704469842635,
476.462296651428));
#271076=CARTESIAN_POINT('Ctrl Pts',(-81.4032507354509,-101.965012102074,
474.462296651428));
#271077=CARTESIAN_POINT('Ctrl Pts',(-88.8775672472034,-94.9701958612989,
472.462296651428));
#271078=CARTESIAN_POINT('Ctrl Pts',(-96.351883758956,-87.9753796205242,
470.462296651428));
#271079=CARTESIAN_POINT('Ctrl Pts',(-102.639948694851,-79.8974404698482,
468.462296651428));
#271080=CARTESIAN_POINT('Ctrl Pts',(-108.928013630747,-71.8195013191721,
466.462296651428));
#271081=CARTESIAN_POINT('Ctrl Pts',(-113.874993963172,-62.8573449296273,
464.462296651428));
#271082=CARTESIAN_POINT('Ctrl Pts',(-118.821974295598,-53.8951885400825,
462.462296651428));
#271083=CARTESIAN_POINT('Ctrl Pts',(-122.306058950682,-44.2694929456714,
460.462296651428));
#271084=CARTESIAN_POINT('Ctrl Pts',(-125.790143605767,-34.6437973512603,
458.462296651428));
#271085=CARTESIAN_POINT('Ctrl Pts',(-127.725542856289,-24.5915791233694,
456.462296651428));
#271086=CARTESIAN_POINT('Ctrl Pts',(-129.660942106811,-14.5393608954785,
454.462296651429));
#271087=CARTESIAN_POINT('Ctrl Pts',(-130.,-4.30813900827813,452.462296651428));
#271088=CARTESIAN_POINT('Ctrl Pts',(-130.339057893189,5.92308287892227,
450.462296651428));
#271089=CARTESIAN_POINT('Ctrl Pts',(-129.073425698447,16.0813817870906,
448.462296651428));
#271090=CARTESIAN_POINT('Ctrl Pts',(-127.807793503705,26.2396806952589,
446.462296651428));
#271091=CARTESIAN_POINT('Ctrl Pts',(-124.968635286058,36.0749255918149,
444.462296651428));
#271092=CARTESIAN_POINT('Ctrl Pts',(-122.129477068411,45.9101704883709,
442.462296651428));
#271093=CARTESIAN_POINT('Ctrl Pts',(-117.786702325803,55.1801850026549,
440.462296651428));
#271094=CARTESIAN_POINT('Ctrl Pts',(-113.443927583196,64.4501995169388,
438.462296651428));
#271095=CARTESIAN_POINT('Ctrl Pts',(-107.704469842635,72.9267251261949,
436.462296651428));
#271096=CARTESIAN_POINT('Ctrl Pts',(-101.965012102074,81.4032507354509,
434.462296651428));
#271097=CARTESIAN_POINT('Ctrl Pts',(-94.9701958612989,88.8775672472034,
432.462296651428));
#271098=CARTESIAN_POINT('Ctrl Pts',(-87.9753796205243,96.3518837589559,
430.462296651428));
#271099=CARTESIAN_POINT('Ctrl Pts',(-79.8974404698482,102.639948694851,
428.462296651428));
#271100=CARTESIAN_POINT('Ctrl Pts',(-71.819501319172,108.928013630747,426.462296651428));
#271101=CARTESIAN_POINT('Ctrl Pts',(-62.8573449296273,113.874993963172,
424.462296651428));
#271102=CARTESIAN_POINT('Ctrl Pts',(-53.8951885400826,118.821974295598,
422.462296651428));
#271103=CARTESIAN_POINT('Ctrl Pts',(-44.2694929456714,122.306058950682,
420.462296651428));
#271104=CARTESIAN_POINT('Ctrl Pts',(-34.6437973512603,125.790143605767,
418.462296651428));
#271105=CARTESIAN_POINT('Ctrl Pts',(-24.5915791233694,127.725542856289,
416.462296651428));
#271106=CARTESIAN_POINT('Ctrl Pts',(-14.5393608954786,129.660942106811,
414.462296651428));
#271107=CARTESIAN_POINT('Ctrl Pts',(-4.30813900827814,130.,412.462296651428));
#271108=CARTESIAN_POINT('Ctrl Pts',(5.92308287892232,130.339057893189,410.462296651428));
#271109=CARTESIAN_POINT('Ctrl Pts',(16.0813817870906,129.073425698447,408.462296651428));
#271110=CARTESIAN_POINT('Ctrl Pts',(26.2396806952589,127.807793503705,406.462296651428));
#271111=CARTESIAN_POINT('Ctrl Pts',(36.0749255918149,124.968635286058,404.462296651428));
#271112=CARTESIAN_POINT('Ctrl Pts',(45.9101704883709,122.129477068411,402.462296651428));
#271113=CARTESIAN_POINT('Ctrl Pts',(55.1801850026549,117.786702325803,400.462296651428));
#271114=CARTESIAN_POINT('Ctrl Pts',(64.4501995169388,113.443927583196,398.462296651428));
#271115=CARTESIAN_POINT('Ctrl Pts',(72.9267251261949,107.704469842635,396.462296651428));
#271116=CARTESIAN_POINT('Ctrl Pts',(81.4032507354509,101.965012102074,394.462296651428));
#271117=CARTESIAN_POINT('Ctrl Pts',(88.8775672472034,94.9701958612989,392.462296651428));
#271118=CARTESIAN_POINT('Ctrl Pts',(96.3518837589559,87.9753796205243,390.462296651428));
#271119=CARTESIAN_POINT('Ctrl Pts',(102.639948694851,79.8974404698482,388.462296651428));
#271120=CARTESIAN_POINT('Ctrl Pts',(108.928013630747,71.819501319172,386.462296651428));
#271121=CARTESIAN_POINT('Ctrl Pts',(113.874993963172,62.8573449296273,384.462296651428));
#271122=CARTESIAN_POINT('Ctrl Pts',(118.821974295598,53.8951885400826,382.462296651428));
#271123=CARTESIAN_POINT('Ctrl Pts',(122.306058950682,44.2694929456714,380.462296651428));
#271124=CARTESIAN_POINT('Ctrl Pts',(125.790143605767,34.6437973512603,378.462296651428));
#271125=CARTESIAN_POINT('Ctrl Pts',(127.725542856289,24.5915791233694,376.462296651428));
#271126=CARTESIAN_POINT('Ctrl Pts',(129.660942106811,14.5393608954786,374.462296651428));
#271127=CARTESIAN_POINT('Ctrl Pts',(130.,4.30813900827812,372.462296651428));
#271128=CARTESIAN_POINT('Ctrl Pts',(160.,4.30813900827813,532.462296651428));
#271129=CARTESIAN_POINT('Ctrl Pts',(160.339057893189,-8.28413408366083,
530.462296651428));
#271130=CARTESIAN_POINT('Ctrl Pts',(158.704075916301,-20.7744157382975,
528.462296651428));
#271131=CARTESIAN_POINT('Ctrl Pts',(157.069093939413,-33.2646973929343,
526.462296651428));
#271132=CARTESIAN_POINT('Ctrl Pts',(153.500330774912,-45.3454354230633,
524.462296651428));
#271133=CARTESIAN_POINT('Ctrl Pts',(149.931567610412,-57.4261734531924,
522.462296651428));
#271134=CARTESIAN_POINT('Ctrl Pts',(144.516898051455,-68.7998999948413,
520.462296651428));
#271135=CARTESIAN_POINT('Ctrl Pts',(139.102228492497,-80.1736265364901,
518.462296651428));
#271136=CARTESIAN_POINT('Ctrl Pts',(131.974979673883,-90.5602826949691,
516.462296651428));
#271137=CARTESIAN_POINT('Ctrl Pts',(124.847730855269,-100.946938853448,
514.462296651428));
#271138=CARTESIAN_POINT('Ctrl Pts',(116.183399296895,-110.0907706828,512.462296651428));
#271139=CARTESIAN_POINT('Ctrl Pts',(107.519067738521,-119.234602512152,
510.462296651428));
#271140=CARTESIAN_POINT('Ctrl Pts',(97.5309980386224,-126.9104585261,508.462296651428));
#271141=CARTESIAN_POINT('Ctrl Pts',(87.5429283387234,-134.586314540048,
506.462296651428));
#271142=CARTESIAN_POINT('Ctrl Pts',(76.4770599218137,-140.605189688823,
504.462296651428));
#271143=CARTESIAN_POINT('Ctrl Pts',(65.4111915049041,-146.624064837599,
502.462296651428));
#271144=CARTESIAN_POINT('Ctrl Pts',(53.5400027769198,-150.837754439537,
500.462296651428));
#271145=CARTESIAN_POINT('Ctrl Pts',(41.6688140489356,-155.051444041475,
498.462296651428));
#271146=CARTESIAN_POINT('Ctrl Pts',(29.2846130745764,-157.356193074143,
496.462296651428));
#271147=CARTESIAN_POINT('Ctrl Pts',(16.9004121002171,-159.660942106811,
494.462296651428));
#271148=CARTESIAN_POINT('Ctrl Pts',(4.30813900827814,-160.,492.462296651428));
#271149=CARTESIAN_POINT('Ctrl Pts',(-8.28413408366082,-160.339057893189,
490.462296651428));
#271150=CARTESIAN_POINT('Ctrl Pts',(-20.7744157382975,-158.704075916301,
488.462296651428));
#271151=CARTESIAN_POINT('Ctrl Pts',(-33.2646973929342,-157.069093939413,
486.462296651428));
#271152=CARTESIAN_POINT('Ctrl Pts',(-45.3454354230633,-153.500330774912,
484.462296651428));
#271153=CARTESIAN_POINT('Ctrl Pts',(-57.4261734531924,-149.931567610412,
482.462296651428));
#271154=CARTESIAN_POINT('Ctrl Pts',(-68.7998999948413,-144.516898051455,
480.462296651428));
#271155=CARTESIAN_POINT('Ctrl Pts',(-80.1736265364901,-139.102228492497,
478.462296651428));
#271156=CARTESIAN_POINT('Ctrl Pts',(-90.5602826949691,-131.974979673883,
476.462296651428));
#271157=CARTESIAN_POINT('Ctrl Pts',(-100.946938853448,-124.847730855269,
474.462296651428));
#271158=CARTESIAN_POINT('Ctrl Pts',(-110.0907706828,-116.183399296895,472.462296651428));
#271159=CARTESIAN_POINT('Ctrl Pts',(-119.234602512152,-107.519067738521,
470.462296651428));
#271160=CARTESIAN_POINT('Ctrl Pts',(-126.9104585261,-97.5309980386224,468.462296651428));
#271161=CARTESIAN_POINT('Ctrl Pts',(-134.586314540048,-87.5429283387234,
466.462296651428));
#271162=CARTESIAN_POINT('Ctrl Pts',(-140.605189688823,-76.4770599218137,
464.462296651428));
#271163=CARTESIAN_POINT('Ctrl Pts',(-146.624064837599,-65.4111915049041,
462.462296651428));
#271164=CARTESIAN_POINT('Ctrl Pts',(-150.837754439537,-53.5400027769199,
460.462296651428));
#271165=CARTESIAN_POINT('Ctrl Pts',(-155.051444041475,-41.6688140489356,
458.462296651428));
#271166=CARTESIAN_POINT('Ctrl Pts',(-157.356193074143,-29.2846130745764,
456.462296651428));
#271167=CARTESIAN_POINT('Ctrl Pts',(-159.660942106811,-16.9004121002171,
454.462296651429));
#271168=CARTESIAN_POINT('Ctrl Pts',(-160.,-4.30813900827815,452.462296651428));
#271169=CARTESIAN_POINT('Ctrl Pts',(-160.339057893189,8.28413408366081,
450.462296651428));
#271170=CARTESIAN_POINT('Ctrl Pts',(-158.704075916301,20.7744157382975,
448.462296651428));
#271171=CARTESIAN_POINT('Ctrl Pts',(-157.069093939413,33.2646973929342,
446.462296651428));
#271172=CARTESIAN_POINT('Ctrl Pts',(-153.500330774912,45.3454354230633,
444.462296651428));
#271173=CARTESIAN_POINT('Ctrl Pts',(-149.931567610412,57.4261734531924,
442.462296651428));
#271174=CARTESIAN_POINT('Ctrl Pts',(-144.516898051455,68.7998999948413,
440.462296651428));
#271175=CARTESIAN_POINT('Ctrl Pts',(-139.102228492497,80.1736265364901,
438.462296651428));
#271176=CARTESIAN_POINT('Ctrl Pts',(-131.974979673883,90.5602826949691,
436.462296651428));
#271177=CARTESIAN_POINT('Ctrl Pts',(-124.847730855269,100.946938853448,
434.462296651428));
#271178=CARTESIAN_POINT('Ctrl Pts',(-116.183399296895,110.0907706828,432.462296651428));
#271179=CARTESIAN_POINT('Ctrl Pts',(-107.519067738521,119.234602512152,
430.462296651428));
#271180=CARTESIAN_POINT('Ctrl Pts',(-97.5309980386224,126.9104585261,428.462296651428));
#271181=CARTESIAN_POINT('Ctrl Pts',(-87.5429283387233,134.586314540048,
426.462296651428));
#271182=CARTESIAN_POINT('Ctrl Pts',(-76.4770599218137,140.605189688823,
424.462296651428));
#271183=CARTESIAN_POINT('Ctrl Pts',(-65.4111915049042,146.624064837599,
422.462296651428));
#271184=CARTESIAN_POINT('Ctrl Pts',(-53.5400027769199,150.837754439537,
420.462296651428));
#271185=CARTESIAN_POINT('Ctrl Pts',(-41.6688140489356,155.051444041475,
418.462296651428));
#271186=CARTESIAN_POINT('Ctrl Pts',(-29.2846130745764,157.356193074143,
416.462296651428));
#271187=CARTESIAN_POINT('Ctrl Pts',(-16.9004121002172,159.660942106811,
414.462296651428));
#271188=CARTESIAN_POINT('Ctrl Pts',(-4.30813900827816,160.,412.462296651428));
#271189=CARTESIAN_POINT('Ctrl Pts',(8.28413408366087,160.339057893189,410.462296651428));
#271190=CARTESIAN_POINT('Ctrl Pts',(20.7744157382975,158.704075916301,408.462296651428));
#271191=CARTESIAN_POINT('Ctrl Pts',(33.2646973929342,157.069093939413,406.462296651428));
#271192=CARTESIAN_POINT('Ctrl Pts',(45.3454354230633,153.500330774912,404.462296651428));
#271193=CARTESIAN_POINT('Ctrl Pts',(57.4261734531925,149.931567610412,402.462296651428));
#271194=CARTESIAN_POINT('Ctrl Pts',(68.7998999948413,144.516898051455,400.462296651428));
#271195=CARTESIAN_POINT('Ctrl Pts',(80.1736265364901,139.102228492498,398.462296651428));
#271196=CARTESIAN_POINT('Ctrl Pts',(90.560282694969,131.974979673883,396.462296651428));
#271197=CARTESIAN_POINT('Ctrl Pts',(100.946938853448,124.847730855269,394.462296651428));
#271198=CARTESIAN_POINT('Ctrl Pts',(110.0907706828,116.183399296895,392.462296651428));
#271199=CARTESIAN_POINT('Ctrl Pts',(119.234602512152,107.519067738521,390.462296651428));
#271200=CARTESIAN_POINT('Ctrl Pts',(126.9104585261,97.5309980386224,388.462296651428));
#271201=CARTESIAN_POINT('Ctrl Pts',(134.586314540048,87.5429283387233,386.462296651428));
#271202=CARTESIAN_POINT('Ctrl Pts',(140.605189688823,76.4770599218137,384.462296651428));
#271203=CARTESIAN_POINT('Ctrl Pts',(146.624064837599,65.4111915049042,382.462296651428));
#271204=CARTESIAN_POINT('Ctrl Pts',(150.837754439537,53.5400027769199,380.462296651428));
#271205=CARTESIAN_POINT('Ctrl Pts',(155.051444041475,41.6688140489356,378.462296651428));
#271206=CARTESIAN_POINT('Ctrl Pts',(157.356193074143,29.2846130745764,376.462296651428));
#271207=CARTESIAN_POINT('Ctrl Pts',(159.660942106811,16.9004121002172,374.462296651428));
#271208=CARTESIAN_POINT('Ctrl Pts',(160.,4.30813900827813,372.462296651428));
#271209=CARTESIAN_POINT('Ctrl Pts',(159.937609420477,-6.20654127333069,
530.789436448355));
#271210=CARTESIAN_POINT('Ctrl Pts',(159.653854600275,-13.5186762622034,
529.624118246284));
#271211=CARTESIAN_POINT('Ctrl Pts',(158.704075916301,-20.7744157382975,
528.462296651428));
#271212=CARTESIAN_POINT('Ctrl Pts',(157.069093939413,-33.2646973929343,
526.462296651428));
#271213=CARTESIAN_POINT('Ctrl Pts',(153.500330774912,-45.3454354230633,
524.462296651428));
#271214=CARTESIAN_POINT('Ctrl Pts',(149.931567610412,-57.4261734531925,
522.462296651428));
#271215=CARTESIAN_POINT('Ctrl Pts',(144.516898051455,-68.7998999948413,
520.462296651428));
#271216=CARTESIAN_POINT('Ctrl Pts',(139.102228492497,-80.1736265364901,
518.462296651428));
#271217=CARTESIAN_POINT('Ctrl Pts',(131.974979673883,-90.5602826949691,
516.462296651428));
#271218=CARTESIAN_POINT('Ctrl Pts',(124.847730855269,-100.946938853448,
514.462296651428));
#271219=CARTESIAN_POINT('Ctrl Pts',(116.183399296895,-110.0907706828,512.462296651428));
#271220=CARTESIAN_POINT('Ctrl Pts',(107.519067738521,-119.234602512152,
510.462296651428));
#271221=CARTESIAN_POINT('Ctrl Pts',(97.5309980386224,-126.9104585261,508.462296651428));
#271222=CARTESIAN_POINT('Ctrl Pts',(87.5429283387234,-134.586314540048,
506.462296651428));
#271223=CARTESIAN_POINT('Ctrl Pts',(76.4770599218137,-140.605189688823,
504.462296651428));
#271224=CARTESIAN_POINT('Ctrl Pts',(65.4111915049041,-146.624064837599,
502.462296651428));
#271225=CARTESIAN_POINT('Ctrl Pts',(53.5400027769198,-150.837754439537,
500.462296651428));
#271226=CARTESIAN_POINT('Ctrl Pts',(41.6688140489356,-155.051444041475,
498.462296651428));
#271227=CARTESIAN_POINT('Ctrl Pts',(29.2846130745764,-157.356193074143,
496.462296651428));
#271228=CARTESIAN_POINT('Ctrl Pts',(16.9004121002171,-159.660942106811,
494.462296651428));
#271229=CARTESIAN_POINT('Ctrl Pts',(4.30813900827814,-160.,492.462296651428));
#271230=CARTESIAN_POINT('Ctrl Pts',(-8.28413408366082,-160.339057893189,
490.462296651428));
#271231=CARTESIAN_POINT('Ctrl Pts',(-20.7744157382975,-158.704075916301,
488.462296651428));
#271232=CARTESIAN_POINT('Ctrl Pts',(-33.2646973929342,-157.069093939413,
486.462296651428));
#271233=CARTESIAN_POINT('Ctrl Pts',(-45.3454354230633,-153.500330774912,
484.462296651428));
#271234=CARTESIAN_POINT('Ctrl Pts',(-57.4261734531924,-149.931567610412,
482.462296651428));
#271235=CARTESIAN_POINT('Ctrl Pts',(-68.7998999948413,-144.516898051455,
480.462296651428));
#271236=CARTESIAN_POINT('Ctrl Pts',(-80.1736265364901,-139.102228492497,
478.462296651428));
#271237=CARTESIAN_POINT('Ctrl Pts',(-90.5602826949691,-131.974979673883,
476.462296651428));
#271238=CARTESIAN_POINT('Ctrl Pts',(-100.946938853448,-124.847730855269,
474.462296651428));
#271239=CARTESIAN_POINT('Ctrl Pts',(-110.0907706828,-116.183399296895,472.462296651428));
#271240=CARTESIAN_POINT('Ctrl Pts',(-119.234602512152,-107.519067738521,
470.462296651428));
#271241=CARTESIAN_POINT('Ctrl Pts',(-126.9104585261,-97.5309980386224,468.462296651428));
#271242=CARTESIAN_POINT('Ctrl Pts',(-134.586314540048,-87.5429283387234,
466.462296651428));
#271243=CARTESIAN_POINT('Ctrl Pts',(-140.605189688823,-76.4770599218137,
464.462296651428));
#271244=CARTESIAN_POINT('Ctrl Pts',(-146.624064837599,-65.4111915049041,
462.462296651428));
#271245=CARTESIAN_POINT('Ctrl Pts',(-150.837754439537,-53.5400027769199,
460.462296651428));
#271246=CARTESIAN_POINT('Ctrl Pts',(-155.051444041475,-41.6688140489356,
458.462296651428));
#271247=CARTESIAN_POINT('Ctrl Pts',(-157.356193074143,-29.2846130745764,
456.462296651428));
#271248=CARTESIAN_POINT('Ctrl Pts',(-159.660942106811,-16.9004121002171,
454.462296651429));
#271249=CARTESIAN_POINT('Ctrl Pts',(-160.,-4.30813900827815,452.462296651428));
#271250=CARTESIAN_POINT('Ctrl Pts',(-160.339057893189,8.28413408366081,
450.462296651428));
#271251=CARTESIAN_POINT('Ctrl Pts',(-158.704075916301,20.7744157382975,
448.462296651428));
#271252=CARTESIAN_POINT('Ctrl Pts',(-157.069093939413,33.2646973929342,
446.462296651428));
#271253=CARTESIAN_POINT('Ctrl Pts',(-153.500330774912,45.3454354230633,
444.462296651428));
#271254=CARTESIAN_POINT('Ctrl Pts',(-149.931567610412,57.4261734531924,
442.462296651428));
#271255=CARTESIAN_POINT('Ctrl Pts',(-144.516898051455,68.7998999948413,
440.462296651428));
#271256=CARTESIAN_POINT('Ctrl Pts',(-139.102228492497,80.1736265364901,
438.462296651428));
#271257=CARTESIAN_POINT('Ctrl Pts',(-131.974979673883,90.5602826949691,
436.462296651428));
#271258=CARTESIAN_POINT('Ctrl Pts',(-124.847730855269,100.946938853448,
434.462296651428));
#271259=CARTESIAN_POINT('Ctrl Pts',(-116.183399296895,110.0907706828,432.462296651428));
#271260=CARTESIAN_POINT('Ctrl Pts',(-107.519067738521,119.234602512152,
430.462296651428));
#271261=CARTESIAN_POINT('Ctrl Pts',(-97.5309980386224,126.9104585261,428.462296651428));
#271262=CARTESIAN_POINT('Ctrl Pts',(-87.5429283387233,134.586314540048,
426.462296651428));
#271263=CARTESIAN_POINT('Ctrl Pts',(-76.4770599218137,140.605189688823,
424.462296651428));
#271264=CARTESIAN_POINT('Ctrl Pts',(-65.4111915049042,146.624064837599,
422.462296651428));
#271265=CARTESIAN_POINT('Ctrl Pts',(-53.5400027769199,150.837754439537,
420.462296651428));
#271266=CARTESIAN_POINT('Ctrl Pts',(-41.6688140489356,155.051444041475,
418.462296651428));
#271267=CARTESIAN_POINT('Ctrl Pts',(-29.2846130745764,157.356193074143,
416.462296651428));
#271268=CARTESIAN_POINT('Ctrl Pts',(-16.9004121002172,159.660942106811,
414.462296651428));
#271269=CARTESIAN_POINT('Ctrl Pts',(-4.30813900827816,160.,412.462296651428));
#271270=CARTESIAN_POINT('Ctrl Pts',(8.28413408366087,160.339057893189,410.462296651428));
#271271=CARTESIAN_POINT('Ctrl Pts',(20.7744157382975,158.704075916301,408.462296651428));
#271272=CARTESIAN_POINT('Ctrl Pts',(33.2646973929342,157.069093939413,406.462296651428));
#271273=CARTESIAN_POINT('Ctrl Pts',(45.3454354230633,153.500330774912,404.462296651428));
#271274=CARTESIAN_POINT('Ctrl Pts',(57.4261734531925,149.931567610412,402.462296651428));
#271275=CARTESIAN_POINT('Ctrl Pts',(68.7998999948413,144.516898051455,400.462296651428));
#271276=CARTESIAN_POINT('Ctrl Pts',(80.1736265364901,139.102228492498,398.462296651428));
#271277=CARTESIAN_POINT('Ctrl Pts',(90.560282694969,131.974979673883,396.462296651428));
#271278=CARTESIAN_POINT('Ctrl Pts',(100.946938853448,124.847730855269,394.462296651428));
#271279=CARTESIAN_POINT('Ctrl Pts',(110.0907706828,116.183399296895,392.462296651428));
#271280=CARTESIAN_POINT('Ctrl Pts',(119.234602512152,107.519067738521,390.462296651428));
#271281=CARTESIAN_POINT('Ctrl Pts',(126.9104585261,97.5309980386224,388.462296651428));
#271282=CARTESIAN_POINT('Ctrl Pts',(134.586314540048,87.5429283387233,386.462296651428));
#271283=CARTESIAN_POINT('Ctrl Pts',(140.605189688823,76.4770599218137,384.462296651428));
#271284=CARTESIAN_POINT('Ctrl Pts',(146.624064837599,65.4111915049042,382.462296651428));
#271285=CARTESIAN_POINT('Ctrl Pts',(150.837754439537,53.5400027769199,380.462296651428));
#271286=CARTESIAN_POINT('Ctrl Pts',(155.051444041475,41.6688140489356,378.462296651428));
#271287=CARTESIAN_POINT('Ctrl Pts',(157.356193074143,29.2846130745764,376.462296651428));
#271288=CARTESIAN_POINT('Ctrl Pts',(159.394142202012,18.3340187941081,374.693818523023));
#271289=CARTESIAN_POINT('Ctrl Pts',(159.895664541343,7.20669984090294,372.923108716584));
#271290=CARTESIAN_POINT('Ctrl Pts',(160.,-4.30813900827805,537.537703348572));
#271291=CARTESIAN_POINT('Ctrl Pts',(159.660942106811,-16.900412100217,535.537703348572));
#271292=CARTESIAN_POINT('Ctrl Pts',(157.356193074143,-29.2846130745763,
533.537703348572));
#271293=CARTESIAN_POINT('Ctrl Pts',(155.051444041475,-41.6688140489355,
531.537703348572));
#271294=CARTESIAN_POINT('Ctrl Pts',(150.837754439537,-53.5400027769198,
529.537703348572));
#271295=CARTESIAN_POINT('Ctrl Pts',(146.624064837599,-65.411191504904,527.537703348572));
#271296=CARTESIAN_POINT('Ctrl Pts',(140.605189688823,-76.4770599218136,
525.537703348572));
#271297=CARTESIAN_POINT('Ctrl Pts',(134.586314540048,-87.5429283387233,
523.537703348572));
#271298=CARTESIAN_POINT('Ctrl Pts',(126.9104585261,-97.5309980386223,521.537703348572));
#271299=CARTESIAN_POINT('Ctrl Pts',(119.234602512152,-107.519067738521,
519.537703348572));
#271300=CARTESIAN_POINT('Ctrl Pts',(110.0907706828,-116.183399296895,517.537703348572));
#271301=CARTESIAN_POINT('Ctrl Pts',(100.946938853448,-124.847730855269,
515.537703348572));
#271302=CARTESIAN_POINT('Ctrl Pts',(90.5602826949691,-131.974979673883,
513.537703348572));
#271303=CARTESIAN_POINT('Ctrl Pts',(80.1736265364902,-139.102228492497,
511.537703348572));
#271304=CARTESIAN_POINT('Ctrl Pts',(68.7998999948414,-144.516898051454,
509.537703348572));
#271305=CARTESIAN_POINT('Ctrl Pts',(57.4261734531925,-149.931567610412,
507.537703348572));
#271306=CARTESIAN_POINT('Ctrl Pts',(45.3454354230634,-153.500330774912,
505.537703348572));
#271307=CARTESIAN_POINT('Ctrl Pts',(33.2646973929343,-157.069093939413,
503.537703348572));
#271308=CARTESIAN_POINT('Ctrl Pts',(20.7744157382976,-158.704075916301,
501.537703348572));
#271309=CARTESIAN_POINT('Ctrl Pts',(8.28413408366091,-160.339057893189,
499.537703348572));
#271310=CARTESIAN_POINT('Ctrl Pts',(-4.30813900827804,-160.,497.537703348572));
#271311=CARTESIAN_POINT('Ctrl Pts',(-16.900412100217,-159.660942106811,
495.537703348572));
#271312=CARTESIAN_POINT('Ctrl Pts',(-29.2846130745763,-157.356193074143,
493.537703348572));
#271313=CARTESIAN_POINT('Ctrl Pts',(-41.6688140489355,-155.051444041475,
491.537703348572));
#271314=CARTESIAN_POINT('Ctrl Pts',(-53.5400027769198,-150.837754439537,
489.537703348572));
#271315=CARTESIAN_POINT('Ctrl Pts',(-65.411191504904,-146.624064837599,
487.537703348572));
#271316=CARTESIAN_POINT('Ctrl Pts',(-76.4770599218136,-140.605189688823,
485.537703348572));
#271317=CARTESIAN_POINT('Ctrl Pts',(-87.5429283387233,-134.586314540048,
483.537703348572));
#271318=CARTESIAN_POINT('Ctrl Pts',(-97.5309980386223,-126.9104585261,481.537703348572));
#271319=CARTESIAN_POINT('Ctrl Pts',(-107.519067738521,-119.234602512152,
479.537703348572));
#271320=CARTESIAN_POINT('Ctrl Pts',(-116.183399296895,-110.0907706828,477.537703348572));
#271321=CARTESIAN_POINT('Ctrl Pts',(-124.847730855269,-100.946938853448,
475.537703348572));
#271322=CARTESIAN_POINT('Ctrl Pts',(-131.974979673883,-90.5602826949692,
473.537703348572));
#271323=CARTESIAN_POINT('Ctrl Pts',(-139.102228492497,-80.1736265364902,
471.537703348572));
#271324=CARTESIAN_POINT('Ctrl Pts',(-144.516898051454,-68.7998999948414,
469.537703348572));
#271325=CARTESIAN_POINT('Ctrl Pts',(-149.931567610412,-57.4261734531925,
467.537703348572));
#271326=CARTESIAN_POINT('Ctrl Pts',(-153.500330774912,-45.3454354230634,
465.537703348572));
#271327=CARTESIAN_POINT('Ctrl Pts',(-157.069093939413,-33.2646973929344,
463.537703348572));
#271328=CARTESIAN_POINT('Ctrl Pts',(-158.704075916301,-20.7744157382976,
461.537703348572));
#271329=CARTESIAN_POINT('Ctrl Pts',(-160.339057893189,-8.28413408366092,
459.537703348572));
#271330=CARTESIAN_POINT('Ctrl Pts',(-160.,4.30813900827803,457.537703348572));
#271331=CARTESIAN_POINT('Ctrl Pts',(-159.660942106811,16.900412100217,455.537703348572));
#271332=CARTESIAN_POINT('Ctrl Pts',(-157.356193074143,29.2846130745763,
453.537703348572));
#271333=CARTESIAN_POINT('Ctrl Pts',(-155.051444041475,41.6688140489355,
451.537703348572));
#271334=CARTESIAN_POINT('Ctrl Pts',(-150.837754439537,53.5400027769198,
449.537703348572));
#271335=CARTESIAN_POINT('Ctrl Pts',(-146.624064837599,65.411191504904,447.537703348572));
#271336=CARTESIAN_POINT('Ctrl Pts',(-140.605189688823,76.4770599218136,
445.537703348572));
#271337=CARTESIAN_POINT('Ctrl Pts',(-134.586314540048,87.5429283387233,
443.537703348572));
#271338=CARTESIAN_POINT('Ctrl Pts',(-126.9104585261,97.5309980386223,441.537703348572));
#271339=CARTESIAN_POINT('Ctrl Pts',(-119.234602512152,107.519067738521,
439.537703348572));
#271340=CARTESIAN_POINT('Ctrl Pts',(-110.0907706828,116.183399296895,437.537703348572));
#271341=CARTESIAN_POINT('Ctrl Pts',(-100.946938853448,124.847730855269,
435.537703348572));
#271342=CARTESIAN_POINT('Ctrl Pts',(-90.5602826949692,131.974979673883,
433.537703348572));
#271343=CARTESIAN_POINT('Ctrl Pts',(-80.1736265364901,139.102228492497,
431.537703348572));
#271344=CARTESIAN_POINT('Ctrl Pts',(-68.7998999948414,144.516898051454,
429.537703348572));
#271345=CARTESIAN_POINT('Ctrl Pts',(-57.4261734531926,149.931567610412,
427.537703348572));
#271346=CARTESIAN_POINT('Ctrl Pts',(-45.3454354230634,153.500330774912,
425.537703348572));
#271347=CARTESIAN_POINT('Ctrl Pts',(-33.2646973929343,157.069093939413,
423.537703348572));
#271348=CARTESIAN_POINT('Ctrl Pts',(-20.7744157382976,158.704075916301,
421.537703348572));
#271349=CARTESIAN_POINT('Ctrl Pts',(-8.284134083661,160.339057893189,419.537703348572));
#271350=CARTESIAN_POINT('Ctrl Pts',(4.30813900827803,160.,417.537703348572));
#271351=CARTESIAN_POINT('Ctrl Pts',(16.9004121002171,159.660942106811,415.537703348572));
#271352=CARTESIAN_POINT('Ctrl Pts',(29.2846130745762,157.356193074143,413.537703348572));
#271353=CARTESIAN_POINT('Ctrl Pts',(41.6688140489354,155.051444041476,411.537703348572));
#271354=CARTESIAN_POINT('Ctrl Pts',(53.5400027769198,150.837754439537,409.537703348572));
#271355=CARTESIAN_POINT('Ctrl Pts',(65.4111915049041,146.624064837599,407.537703348572));
#271356=CARTESIAN_POINT('Ctrl Pts',(76.4770599218136,140.605189688823,405.537703348572));
#271357=CARTESIAN_POINT('Ctrl Pts',(87.5429283387232,134.586314540048,403.537703348572));
#271358=CARTESIAN_POINT('Ctrl Pts',(97.5309980386223,126.9104585261,401.537703348572));
#271359=CARTESIAN_POINT('Ctrl Pts',(107.519067738521,119.234602512152,399.537703348572));
#271360=CARTESIAN_POINT('Ctrl Pts',(116.183399296895,110.0907706828,397.537703348572));
#271361=CARTESIAN_POINT('Ctrl Pts',(124.847730855269,100.946938853448,395.537703348572));
#271362=CARTESIAN_POINT('Ctrl Pts',(131.974979673883,90.5602826949692,393.537703348572));
#271363=CARTESIAN_POINT('Ctrl Pts',(139.102228492497,80.1736265364902,391.537703348572));
#271364=CARTESIAN_POINT('Ctrl Pts',(144.516898051454,68.7998999948414,389.537703348572));
#271365=CARTESIAN_POINT('Ctrl Pts',(149.931567610412,57.4261734531926,387.537703348572));
#271366=CARTESIAN_POINT('Ctrl Pts',(153.500330774912,45.3454354230634,385.537703348572));
#271367=CARTESIAN_POINT('Ctrl Pts',(157.069093939413,33.2646973929343,383.537703348572));
#271368=CARTESIAN_POINT('Ctrl Pts',(158.704075916301,20.7744157382976,381.537703348572));
#271369=CARTESIAN_POINT('Ctrl Pts',(160.339057893189,8.28413408366101,379.537703348572));
#271370=CARTESIAN_POINT('Ctrl Pts',(160.,-4.30813900827805,377.537703348572));
#271371=CARTESIAN_POINT('Ctrl Pts',(130.,-4.30813900827807,537.537703348572));
#271372=CARTESIAN_POINT('Ctrl Pts',(129.660942106811,-14.5393608954785,
535.537703348572));
#271373=CARTESIAN_POINT('Ctrl Pts',(127.725542856289,-24.5915791233694,
533.537703348572));
#271374=CARTESIAN_POINT('Ctrl Pts',(125.790143605767,-34.6437973512603,
531.537703348572));
#271375=CARTESIAN_POINT('Ctrl Pts',(122.306058950682,-44.2694929456714,
529.537703348572));
#271376=CARTESIAN_POINT('Ctrl Pts',(118.821974295598,-53.8951885400825,
527.537703348572));
#271377=CARTESIAN_POINT('Ctrl Pts',(113.874993963172,-62.8573449296272,
525.537703348572));
#271378=CARTESIAN_POINT('Ctrl Pts',(108.928013630747,-71.819501319172,523.537703348572));
#271379=CARTESIAN_POINT('Ctrl Pts',(102.639948694851,-79.8974404698481,
521.537703348572));
#271380=CARTESIAN_POINT('Ctrl Pts',(96.351883758956,-87.9753796205242,519.537703348572));
#271381=CARTESIAN_POINT('Ctrl Pts',(88.8775672472035,-94.9701958612989,
517.537703348572));
#271382=CARTESIAN_POINT('Ctrl Pts',(81.403250735451,-101.965012102074,515.537703348572));
#271383=CARTESIAN_POINT('Ctrl Pts',(72.9267251261949,-107.704469842635,
513.537703348572));
#271384=CARTESIAN_POINT('Ctrl Pts',(64.4501995169389,-113.443927583196,
511.537703348572));
#271385=CARTESIAN_POINT('Ctrl Pts',(55.1801850026549,-117.786702325803,
509.537703348572));
#271386=CARTESIAN_POINT('Ctrl Pts',(45.910170488371,-122.129477068411,507.537703348572));
#271387=CARTESIAN_POINT('Ctrl Pts',(36.074925591815,-124.968635286058,505.537703348572));
#271388=CARTESIAN_POINT('Ctrl Pts',(26.239680695259,-127.807793503704,503.537703348572));
#271389=CARTESIAN_POINT('Ctrl Pts',(16.0813817870907,-129.073425698447,
501.537703348572));
#271390=CARTESIAN_POINT('Ctrl Pts',(5.92308287892234,-130.339057893189,
499.537703348572));
#271391=CARTESIAN_POINT('Ctrl Pts',(-4.30813900827806,-130.,497.537703348572));
#271392=CARTESIAN_POINT('Ctrl Pts',(-14.5393608954785,-129.660942106811,
495.537703348572));
#271393=CARTESIAN_POINT('Ctrl Pts',(-24.5915791233694,-127.725542856289,
493.537703348572));
#271394=CARTESIAN_POINT('Ctrl Pts',(-34.6437973512603,-125.790143605767,
491.537703348572));
#271395=CARTESIAN_POINT('Ctrl Pts',(-44.2694929456713,-122.306058950682,
489.537703348572));
#271396=CARTESIAN_POINT('Ctrl Pts',(-53.8951885400825,-118.821974295598,
487.537703348572));
#271397=CARTESIAN_POINT('Ctrl Pts',(-62.8573449296272,-113.874993963172,
485.537703348572));
#271398=CARTESIAN_POINT('Ctrl Pts',(-71.819501319172,-108.928013630747,
483.537703348572));
#271399=CARTESIAN_POINT('Ctrl Pts',(-79.8974404698481,-102.639948694851,
481.537703348572));
#271400=CARTESIAN_POINT('Ctrl Pts',(-87.9753796205242,-96.351883758956,
479.537703348572));
#271401=CARTESIAN_POINT('Ctrl Pts',(-94.9701958612989,-88.8775672472035,
477.537703348572));
#271402=CARTESIAN_POINT('Ctrl Pts',(-101.965012102074,-81.403250735451,
475.537703348572));
#271403=CARTESIAN_POINT('Ctrl Pts',(-107.704469842635,-72.9267251261949,
473.537703348572));
#271404=CARTESIAN_POINT('Ctrl Pts',(-113.443927583196,-64.4501995169389,
471.537703348572));
#271405=CARTESIAN_POINT('Ctrl Pts',(-117.786702325803,-55.1801850026549,
469.537703348572));
#271406=CARTESIAN_POINT('Ctrl Pts',(-122.129477068411,-45.910170488371,
467.537703348572));
#271407=CARTESIAN_POINT('Ctrl Pts',(-124.968635286058,-36.074925591815,
465.537703348572));
#271408=CARTESIAN_POINT('Ctrl Pts',(-127.807793503704,-26.239680695259,
463.537703348572));
#271409=CARTESIAN_POINT('Ctrl Pts',(-129.073425698447,-16.0813817870907,
461.537703348572));
#271410=CARTESIAN_POINT('Ctrl Pts',(-130.339057893189,-5.92308287892235,
459.537703348572));
#271411=CARTESIAN_POINT('Ctrl Pts',(-130.,4.30813900827805,457.537703348572));
#271412=CARTESIAN_POINT('Ctrl Pts',(-129.660942106811,14.5393608954784,
455.537703348572));
#271413=CARTESIAN_POINT('Ctrl Pts',(-127.725542856289,24.5915791233693,
453.537703348572));
#271414=CARTESIAN_POINT('Ctrl Pts',(-125.790143605767,34.6437973512602,
451.537703348572));
#271415=CARTESIAN_POINT('Ctrl Pts',(-122.306058950682,44.2694929456713,
449.537703348572));
#271416=CARTESIAN_POINT('Ctrl Pts',(-118.821974295598,53.8951885400825,
447.537703348572));
#271417=CARTESIAN_POINT('Ctrl Pts',(-113.874993963172,62.8573449296272,
445.537703348572));
#271418=CARTESIAN_POINT('Ctrl Pts',(-108.928013630747,71.819501319172,443.537703348572));
#271419=CARTESIAN_POINT('Ctrl Pts',(-102.639948694851,79.8974404698481,
441.537703348572));
#271420=CARTESIAN_POINT('Ctrl Pts',(-96.3518837589561,87.9753796205242,
439.537703348572));
#271421=CARTESIAN_POINT('Ctrl Pts',(-88.8775672472035,94.9701958612989,
437.537703348572));
#271422=CARTESIAN_POINT('Ctrl Pts',(-81.403250735451,101.965012102074,435.537703348572));
#271423=CARTESIAN_POINT('Ctrl Pts',(-72.9267251261949,107.704469842635,
433.537703348572));
#271424=CARTESIAN_POINT('Ctrl Pts',(-64.4501995169389,113.443927583196,
431.537703348572));
#271425=CARTESIAN_POINT('Ctrl Pts',(-55.1801850026549,117.786702325803,
429.537703348572));
#271426=CARTESIAN_POINT('Ctrl Pts',(-45.910170488371,122.129477068411,427.537703348572));
#271427=CARTESIAN_POINT('Ctrl Pts',(-36.074925591815,124.968635286058,425.537703348572));
#271428=CARTESIAN_POINT('Ctrl Pts',(-26.239680695259,127.807793503704,423.537703348572));
#271429=CARTESIAN_POINT('Ctrl Pts',(-16.0813817870907,129.073425698447,
421.537703348572));
#271430=CARTESIAN_POINT('Ctrl Pts',(-5.92308287892242,130.339057893189,
419.537703348572));
#271431=CARTESIAN_POINT('Ctrl Pts',(4.30813900827804,130.,417.537703348572));
#271432=CARTESIAN_POINT('Ctrl Pts',(14.5393608954785,129.660942106811,415.537703348572));
#271433=CARTESIAN_POINT('Ctrl Pts',(24.5915791233693,127.725542856289,413.537703348572));
#271434=CARTESIAN_POINT('Ctrl Pts',(34.6437973512602,125.790143605767,411.537703348572));
#271435=CARTESIAN_POINT('Ctrl Pts',(44.2694929456713,122.306058950682,409.537703348572));
#271436=CARTESIAN_POINT('Ctrl Pts',(53.8951885400825,118.821974295598,407.537703348572));
#271437=CARTESIAN_POINT('Ctrl Pts',(62.8573449296272,113.874993963172,405.537703348572));
#271438=CARTESIAN_POINT('Ctrl Pts',(71.819501319172,108.928013630747,403.537703348572));
#271439=CARTESIAN_POINT('Ctrl Pts',(79.8974404698481,102.639948694851,401.537703348572));
#271440=CARTESIAN_POINT('Ctrl Pts',(87.9753796205242,96.351883758956,399.537703348572));
#271441=CARTESIAN_POINT('Ctrl Pts',(94.9701958612989,88.8775672472035,397.537703348572));
#271442=CARTESIAN_POINT('Ctrl Pts',(101.965012102074,81.403250735451,395.537703348572));
#271443=CARTESIAN_POINT('Ctrl Pts',(107.704469842635,72.926725126195,393.537703348572));
#271444=CARTESIAN_POINT('Ctrl Pts',(113.443927583196,64.4501995169389,391.537703348572));
#271445=CARTESIAN_POINT('Ctrl Pts',(117.786702325803,55.1801850026549,389.537703348572));
#271446=CARTESIAN_POINT('Ctrl Pts',(122.129477068411,45.910170488371,387.537703348572));
#271447=CARTESIAN_POINT('Ctrl Pts',(124.968635286058,36.074925591815,385.537703348572));
#271448=CARTESIAN_POINT('Ctrl Pts',(127.807793503704,26.239680695259,383.537703348572));
#271449=CARTESIAN_POINT('Ctrl Pts',(129.073425698447,16.0813817870907,381.537703348572));
#271450=CARTESIAN_POINT('Ctrl Pts',(130.339057893189,5.92308287892242,379.537703348572));
#271451=CARTESIAN_POINT('Ctrl Pts',(130.,-4.30813900827807,377.537703348572));
#271452=CARTESIAN_POINT('Ctrl Pts',(159.895664541343,-7.20669984090288,
537.076891283416));
#271453=CARTESIAN_POINT('Ctrl Pts',(159.394142202012,-18.334018794108,535.306181476978));
#271454=CARTESIAN_POINT('Ctrl Pts',(157.356193074143,-29.2846130745763,
533.537703348572));
#271455=CARTESIAN_POINT('Ctrl Pts',(155.051444041475,-41.6688140489355,
531.537703348572));
#271456=CARTESIAN_POINT('Ctrl Pts',(150.837754439537,-53.5400027769198,
529.537703348572));
#271457=CARTESIAN_POINT('Ctrl Pts',(146.624064837599,-65.411191504904,527.537703348572));
#271458=CARTESIAN_POINT('Ctrl Pts',(140.605189688823,-76.4770599218136,
525.537703348572));
#271459=CARTESIAN_POINT('Ctrl Pts',(134.586314540048,-87.5429283387233,
523.537703348572));
#271460=CARTESIAN_POINT('Ctrl Pts',(126.9104585261,-97.5309980386223,521.537703348572));
#271461=CARTESIAN_POINT('Ctrl Pts',(119.234602512152,-107.519067738521,
519.537703348572));
#271462=CARTESIAN_POINT('Ctrl Pts',(110.0907706828,-116.183399296895,517.537703348572));
#271463=CARTESIAN_POINT('Ctrl Pts',(100.946938853448,-124.847730855269,
515.537703348572));
#271464=CARTESIAN_POINT('Ctrl Pts',(90.5602826949691,-131.974979673883,
513.537703348572));
#271465=CARTESIAN_POINT('Ctrl Pts',(80.1736265364902,-139.102228492497,
511.537703348572));
#271466=CARTESIAN_POINT('Ctrl Pts',(68.7998999948414,-144.516898051454,
509.537703348572));
#271467=CARTESIAN_POINT('Ctrl Pts',(57.4261734531925,-149.931567610412,
507.537703348572));
#271468=CARTESIAN_POINT('Ctrl Pts',(45.3454354230634,-153.500330774912,
505.537703348572));
#271469=CARTESIAN_POINT('Ctrl Pts',(33.2646973929343,-157.069093939413,
503.537703348572));
#271470=CARTESIAN_POINT('Ctrl Pts',(20.7744157382976,-158.704075916301,
501.537703348572));
#271471=CARTESIAN_POINT('Ctrl Pts',(8.28413408366091,-160.339057893189,
499.537703348572));
#271472=CARTESIAN_POINT('Ctrl Pts',(-4.30813900827804,-160.,497.537703348572));
#271473=CARTESIAN_POINT('Ctrl Pts',(-16.900412100217,-159.660942106811,
495.537703348572));
#271474=CARTESIAN_POINT('Ctrl Pts',(-29.2846130745763,-157.356193074143,
493.537703348572));
#271475=CARTESIAN_POINT('Ctrl Pts',(-41.6688140489355,-155.051444041475,
491.537703348572));
#271476=CARTESIAN_POINT('Ctrl Pts',(-53.5400027769198,-150.837754439537,
489.537703348572));
#271477=CARTESIAN_POINT('Ctrl Pts',(-65.411191504904,-146.624064837599,
487.537703348572));
#271478=CARTESIAN_POINT('Ctrl Pts',(-76.4770599218136,-140.605189688823,
485.537703348572));
#271479=CARTESIAN_POINT('Ctrl Pts',(-87.5429283387233,-134.586314540048,
483.537703348572));
#271480=CARTESIAN_POINT('Ctrl Pts',(-97.5309980386223,-126.9104585261,481.537703348572));
#271481=CARTESIAN_POINT('Ctrl Pts',(-107.519067738521,-119.234602512152,
479.537703348572));
#271482=CARTESIAN_POINT('Ctrl Pts',(-116.183399296895,-110.0907706828,477.537703348572));
#271483=CARTESIAN_POINT('Ctrl Pts',(-124.847730855269,-100.946938853448,
475.537703348572));
#271484=CARTESIAN_POINT('Ctrl Pts',(-131.974979673883,-90.5602826949692,
473.537703348572));
#271485=CARTESIAN_POINT('Ctrl Pts',(-139.102228492497,-80.1736265364902,
471.537703348572));
#271486=CARTESIAN_POINT('Ctrl Pts',(-144.516898051454,-68.7998999948414,
469.537703348572));
#271487=CARTESIAN_POINT('Ctrl Pts',(-149.931567610412,-57.4261734531925,
467.537703348572));
#271488=CARTESIAN_POINT('Ctrl Pts',(-153.500330774912,-45.3454354230634,
465.537703348572));
#271489=CARTESIAN_POINT('Ctrl Pts',(-157.069093939413,-33.2646973929344,
463.537703348572));
#271490=CARTESIAN_POINT('Ctrl Pts',(-158.704075916301,-20.7744157382976,
461.537703348572));
#271491=CARTESIAN_POINT('Ctrl Pts',(-160.339057893189,-8.28413408366092,
459.537703348572));
#271492=CARTESIAN_POINT('Ctrl Pts',(-160.,4.30813900827803,457.537703348572));
#271493=CARTESIAN_POINT('Ctrl Pts',(-159.660942106811,16.900412100217,455.537703348572));
#271494=CARTESIAN_POINT('Ctrl Pts',(-157.356193074143,29.2846130745763,
453.537703348572));
#271495=CARTESIAN_POINT('Ctrl Pts',(-155.051444041475,41.6688140489355,
451.537703348572));
#271496=CARTESIAN_POINT('Ctrl Pts',(-150.837754439537,53.5400027769198,
449.537703348572));
#271497=CARTESIAN_POINT('Ctrl Pts',(-146.624064837599,65.411191504904,447.537703348572));
#271498=CARTESIAN_POINT('Ctrl Pts',(-140.605189688823,76.4770599218136,
445.537703348572));
#271499=CARTESIAN_POINT('Ctrl Pts',(-134.586314540048,87.5429283387233,
443.537703348572));
#271500=CARTESIAN_POINT('Ctrl Pts',(-126.9104585261,97.5309980386223,441.537703348572));
#271501=CARTESIAN_POINT('Ctrl Pts',(-119.234602512152,107.519067738521,
439.537703348572));
#271502=CARTESIAN_POINT('Ctrl Pts',(-110.0907706828,116.183399296895,437.537703348572));
#271503=CARTESIAN_POINT('Ctrl Pts',(-100.946938853448,124.847730855269,
435.537703348572));
#271504=CARTESIAN_POINT('Ctrl Pts',(-90.5602826949692,131.974979673883,
433.537703348572));
#271505=CARTESIAN_POINT('Ctrl Pts',(-80.1736265364902,139.102228492497,
431.537703348572));
#271506=CARTESIAN_POINT('Ctrl Pts',(-68.7998999948414,144.516898051454,
429.537703348572));
#271507=CARTESIAN_POINT('Ctrl Pts',(-57.4261734531926,149.931567610412,
427.537703348572));
#271508=CARTESIAN_POINT('Ctrl Pts',(-45.3454354230634,153.500330774912,
425.537703348572));
#271509=CARTESIAN_POINT('Ctrl Pts',(-33.2646973929343,157.069093939413,
423.537703348572));
#271510=CARTESIAN_POINT('Ctrl Pts',(-20.7744157382976,158.704075916301,
421.537703348572));
#271511=CARTESIAN_POINT('Ctrl Pts',(-8.284134083661,160.339057893189,419.537703348572));
#271512=CARTESIAN_POINT('Ctrl Pts',(4.30813900827803,160.,417.537703348572));
#271513=CARTESIAN_POINT('Ctrl Pts',(16.9004121002171,159.660942106811,415.537703348572));
#271514=CARTESIAN_POINT('Ctrl Pts',(29.2846130745762,157.356193074143,413.537703348572));
#271515=CARTESIAN_POINT('Ctrl Pts',(41.6688140489354,155.051444041476,411.537703348572));
#271516=CARTESIAN_POINT('Ctrl Pts',(53.5400027769198,150.837754439537,409.537703348572));
#271517=CARTESIAN_POINT('Ctrl Pts',(65.4111915049041,146.624064837599,407.537703348572));
#271518=CARTESIAN_POINT('Ctrl Pts',(76.4770599218136,140.605189688823,405.537703348572));
#271519=CARTESIAN_POINT('Ctrl Pts',(87.5429283387232,134.586314540048,403.537703348572));
#271520=CARTESIAN_POINT('Ctrl Pts',(97.5309980386223,126.9104585261,401.537703348572));
#271521=CARTESIAN_POINT('Ctrl Pts',(107.519067738521,119.234602512152,399.537703348572));
#271522=CARTESIAN_POINT('Ctrl Pts',(116.183399296895,110.0907706828,397.537703348572));
#271523=CARTESIAN_POINT('Ctrl Pts',(124.847730855269,100.946938853448,395.537703348572));
#271524=CARTESIAN_POINT('Ctrl Pts',(131.974979673883,90.5602826949692,393.537703348572));
#271525=CARTESIAN_POINT('Ctrl Pts',(139.102228492497,80.1736265364902,391.537703348572));
#271526=CARTESIAN_POINT('Ctrl Pts',(144.516898051454,68.7998999948414,389.537703348572));
#271527=CARTESIAN_POINT('Ctrl Pts',(149.931567610412,57.4261734531926,387.537703348572));
#271528=CARTESIAN_POINT('Ctrl Pts',(153.500330774912,45.3454354230634,385.537703348572));
#271529=CARTESIAN_POINT('Ctrl Pts',(157.069093939413,33.2646973929343,383.537703348572));
#271530=CARTESIAN_POINT('Ctrl Pts',(158.704075916301,20.7744157382976,381.537703348572));
#271531=CARTESIAN_POINT('Ctrl Pts',(159.653854600275,13.5186762622035,380.375881753716));
#271532=CARTESIAN_POINT('Ctrl Pts',(159.937609420477,6.20654127333073,379.210563551645));
#271533=CARTESIAN_POINT('Ctrl Pts',(160.,4.30813900827813,532.462296651428));
#271534=CARTESIAN_POINT('Ctrl Pts',(160.339057893189,-8.28413408366083,
530.462296651428));
#271535=CARTESIAN_POINT('Ctrl Pts',(158.704075916301,-20.7744157382975,
528.462296651428));
#271536=CARTESIAN_POINT('Ctrl Pts',(157.069093939413,-33.2646973929343,
526.462296651428));
#271537=CARTESIAN_POINT('Ctrl Pts',(153.500330774912,-45.3454354230633,
524.462296651428));
#271538=CARTESIAN_POINT('Ctrl Pts',(149.931567610412,-57.4261734531924,
522.462296651428));
#271539=CARTESIAN_POINT('Ctrl Pts',(144.516898051455,-68.7998999948413,
520.462296651428));
#271540=CARTESIAN_POINT('Ctrl Pts',(139.102228492497,-80.1736265364901,
518.462296651428));
#271541=CARTESIAN_POINT('Ctrl Pts',(131.974979673883,-90.5602826949691,
516.462296651428));
#271542=CARTESIAN_POINT('Ctrl Pts',(124.847730855269,-100.946938853448,
514.462296651428));
#271543=CARTESIAN_POINT('Ctrl Pts',(116.183399296895,-110.0907706828,512.462296651428));
#271544=CARTESIAN_POINT('Ctrl Pts',(107.519067738521,-119.234602512152,
510.462296651428));
#271545=CARTESIAN_POINT('Ctrl Pts',(97.5309980386224,-126.9104585261,508.462296651428));
#271546=CARTESIAN_POINT('Ctrl Pts',(87.5429283387234,-134.586314540048,
506.462296651428));
#271547=CARTESIAN_POINT('Ctrl Pts',(76.4770599218137,-140.605189688823,
504.462296651428));
#271548=CARTESIAN_POINT('Ctrl Pts',(65.4111915049041,-146.624064837599,
502.462296651428));
#271549=CARTESIAN_POINT('Ctrl Pts',(53.5400027769198,-150.837754439537,
500.462296651428));
#271550=CARTESIAN_POINT('Ctrl Pts',(41.6688140489356,-155.051444041475,
498.462296651428));
#271551=CARTESIAN_POINT('Ctrl Pts',(29.2846130745764,-157.356193074143,
496.462296651428));
#271552=CARTESIAN_POINT('Ctrl Pts',(16.9004121002171,-159.660942106811,
494.462296651428));
#271553=CARTESIAN_POINT('Ctrl Pts',(4.30813900827814,-160.,492.462296651428));
#271554=CARTESIAN_POINT('Ctrl Pts',(-8.28413408366082,-160.339057893189,
490.462296651428));
#271555=CARTESIAN_POINT('Ctrl Pts',(-20.7744157382975,-158.704075916301,
488.462296651428));
#271556=CARTESIAN_POINT('Ctrl Pts',(-33.2646973929342,-157.069093939413,
486.462296651428));
#271557=CARTESIAN_POINT('Ctrl Pts',(-45.3454354230633,-153.500330774912,
484.462296651428));
#271558=CARTESIAN_POINT('Ctrl Pts',(-57.4261734531924,-149.931567610412,
482.462296651428));
#271559=CARTESIAN_POINT('Ctrl Pts',(-68.7998999948413,-144.516898051455,
480.462296651428));
#271560=CARTESIAN_POINT('Ctrl Pts',(-80.1736265364901,-139.102228492497,
478.462296651428));
#271561=CARTESIAN_POINT('Ctrl Pts',(-90.5602826949691,-131.974979673883,
476.462296651428));
#271562=CARTESIAN_POINT('Ctrl Pts',(-100.946938853448,-124.847730855269,
474.462296651428));
#271563=CARTESIAN_POINT('Ctrl Pts',(-110.0907706828,-116.183399296895,472.462296651428));
#271564=CARTESIAN_POINT('Ctrl Pts',(-119.234602512152,-107.519067738521,
470.462296651428));
#271565=CARTESIAN_POINT('Ctrl Pts',(-126.9104585261,-97.5309980386224,468.462296651428));
#271566=CARTESIAN_POINT('Ctrl Pts',(-134.586314540048,-87.5429283387234,
466.462296651428));
#271567=CARTESIAN_POINT('Ctrl Pts',(-140.605189688823,-76.4770599218137,
464.462296651428));
#271568=CARTESIAN_POINT('Ctrl Pts',(-146.624064837599,-65.4111915049041,
462.462296651428));
#271569=CARTESIAN_POINT('Ctrl Pts',(-150.837754439537,-53.5400027769199,
460.462296651428));
#271570=CARTESIAN_POINT('Ctrl Pts',(-155.051444041475,-41.6688140489356,
458.462296651428));
#271571=CARTESIAN_POINT('Ctrl Pts',(-157.356193074143,-29.2846130745764,
456.462296651428));
#271572=CARTESIAN_POINT('Ctrl Pts',(-159.660942106811,-16.9004121002171,
454.462296651429));
#271573=CARTESIAN_POINT('Ctrl Pts',(-160.,-4.30813900827815,452.462296651428));
#271574=CARTESIAN_POINT('Ctrl Pts',(-160.339057893189,8.28413408366081,
450.462296651428));
#271575=CARTESIAN_POINT('Ctrl Pts',(-158.704075916301,20.7744157382975,
448.462296651428));
#271576=CARTESIAN_POINT('Ctrl Pts',(-157.069093939413,33.2646973929342,
446.462296651428));
#271577=CARTESIAN_POINT('Ctrl Pts',(-153.500330774912,45.3454354230633,
444.462296651428));
#271578=CARTESIAN_POINT('Ctrl Pts',(-149.931567610412,57.4261734531924,
442.462296651428));
#271579=CARTESIAN_POINT('Ctrl Pts',(-144.516898051455,68.7998999948413,
440.462296651428));
#271580=CARTESIAN_POINT('Ctrl Pts',(-139.102228492497,80.1736265364901,
438.462296651428));
#271581=CARTESIAN_POINT('Ctrl Pts',(-131.974979673883,90.5602826949691,
436.462296651428));
#271582=CARTESIAN_POINT('Ctrl Pts',(-124.847730855269,100.946938853448,
434.462296651428));
#271583=CARTESIAN_POINT('Ctrl Pts',(-116.183399296895,110.0907706828,432.462296651428));
#271584=CARTESIAN_POINT('Ctrl Pts',(-107.519067738521,119.234602512152,
430.462296651428));
#271585=CARTESIAN_POINT('Ctrl Pts',(-97.5309980386224,126.9104585261,428.462296651428));
#271586=CARTESIAN_POINT('Ctrl Pts',(-87.5429283387233,134.586314540048,
426.462296651428));
#271587=CARTESIAN_POINT('Ctrl Pts',(-76.4770599218137,140.605189688823,
424.462296651428));
#271588=CARTESIAN_POINT('Ctrl Pts',(-65.4111915049042,146.624064837599,
422.462296651428));
#271589=CARTESIAN_POINT('Ctrl Pts',(-53.5400027769199,150.837754439537,
420.462296651428));
#271590=CARTESIAN_POINT('Ctrl Pts',(-41.6688140489356,155.051444041475,
418.462296651428));
#271591=CARTESIAN_POINT('Ctrl Pts',(-29.2846130745764,157.356193074143,
416.462296651428));
#271592=CARTESIAN_POINT('Ctrl Pts',(-16.9004121002172,159.660942106811,
414.462296651428));
#271593=CARTESIAN_POINT('Ctrl Pts',(-4.30813900827816,160.,412.462296651428));
#271594=CARTESIAN_POINT('Ctrl Pts',(8.28413408366087,160.339057893189,410.462296651428));
#271595=CARTESIAN_POINT('Ctrl Pts',(20.7744157382975,158.704075916301,408.462296651428));
#271596=CARTESIAN_POINT('Ctrl Pts',(33.2646973929342,157.069093939413,406.462296651428));
#271597=CARTESIAN_POINT('Ctrl Pts',(45.3454354230633,153.500330774912,404.462296651428));
#271598=CARTESIAN_POINT('Ctrl Pts',(57.4261734531925,149.931567610412,402.462296651428));
#271599=CARTESIAN_POINT('Ctrl Pts',(68.7998999948413,144.516898051455,400.462296651428));
#271600=CARTESIAN_POINT('Ctrl Pts',(80.1736265364901,139.102228492498,398.462296651428));
#271601=CARTESIAN_POINT('Ctrl Pts',(90.560282694969,131.974979673883,396.462296651428));
#271602=CARTESIAN_POINT('Ctrl Pts',(100.946938853448,124.847730855269,394.462296651428));
#271603=CARTESIAN_POINT('Ctrl Pts',(110.0907706828,116.183399296895,392.462296651428));
#271604=CARTESIAN_POINT('Ctrl Pts',(119.234602512152,107.519067738521,390.462296651428));
#271605=CARTESIAN_POINT('Ctrl Pts',(126.9104585261,97.5309980386224,388.462296651428));
#271606=CARTESIAN_POINT('Ctrl Pts',(134.586314540048,87.5429283387233,386.462296651428));
#271607=CARTESIAN_POINT('Ctrl Pts',(140.605189688823,76.4770599218137,384.462296651428));
#271608=CARTESIAN_POINT('Ctrl Pts',(146.624064837599,65.4111915049042,382.462296651428));
#271609=CARTESIAN_POINT('Ctrl Pts',(150.837754439537,53.5400027769199,380.462296651428));
#271610=CARTESIAN_POINT('Ctrl Pts',(155.051444041475,41.6688140489356,378.462296651428));
#271611=CARTESIAN_POINT('Ctrl Pts',(157.356193074143,29.2846130745764,376.462296651428));
#271612=CARTESIAN_POINT('Ctrl Pts',(159.660942106811,16.9004121002172,374.462296651428));
#271613=CARTESIAN_POINT('Ctrl Pts',(160.,4.30813900827813,372.462296651428));
#271614=CARTESIAN_POINT('Ctrl Pts',(160.,-4.30813900827805,537.537703348572));
#271615=CARTESIAN_POINT('Ctrl Pts',(159.660942106811,-16.900412100217,535.537703348572));
#271616=CARTESIAN_POINT('Ctrl Pts',(157.356193074143,-29.2846130745763,
533.537703348572));
#271617=CARTESIAN_POINT('Ctrl Pts',(155.051444041475,-41.6688140489355,
531.537703348572));
#271618=CARTESIAN_POINT('Ctrl Pts',(150.837754439537,-53.5400027769198,
529.537703348572));
#271619=CARTESIAN_POINT('Ctrl Pts',(146.624064837599,-65.411191504904,527.537703348572));
#271620=CARTESIAN_POINT('Ctrl Pts',(140.605189688823,-76.4770599218136,
525.537703348572));
#271621=CARTESIAN_POINT('Ctrl Pts',(134.586314540048,-87.5429283387233,
523.537703348572));
#271622=CARTESIAN_POINT('Ctrl Pts',(126.9104585261,-97.5309980386223,521.537703348572));
#271623=CARTESIAN_POINT('Ctrl Pts',(119.234602512152,-107.519067738521,
519.537703348572));
#271624=CARTESIAN_POINT('Ctrl Pts',(110.0907706828,-116.183399296895,517.537703348572));
#271625=CARTESIAN_POINT('Ctrl Pts',(100.946938853448,-124.847730855269,
515.537703348572));
#271626=CARTESIAN_POINT('Ctrl Pts',(90.5602826949691,-131.974979673883,
513.537703348572));
#271627=CARTESIAN_POINT('Ctrl Pts',(80.1736265364902,-139.102228492497,
511.537703348572));
#271628=CARTESIAN_POINT('Ctrl Pts',(68.7998999948414,-144.516898051454,
509.537703348572));
#271629=CARTESIAN_POINT('Ctrl Pts',(57.4261734531925,-149.931567610412,
507.537703348572));
#271630=CARTESIAN_POINT('Ctrl Pts',(45.3454354230634,-153.500330774912,
505.537703348572));
#271631=CARTESIAN_POINT('Ctrl Pts',(33.2646973929343,-157.069093939413,
503.537703348572));
#271632=CARTESIAN_POINT('Ctrl Pts',(20.7744157382976,-158.704075916301,
501.537703348572));
#271633=CARTESIAN_POINT('Ctrl Pts',(8.28413408366091,-160.339057893189,
499.537703348572));
#271634=CARTESIAN_POINT('Ctrl Pts',(-4.30813900827804,-160.,497.537703348572));
#271635=CARTESIAN_POINT('Ctrl Pts',(-16.900412100217,-159.660942106811,
495.537703348572));
#271636=CARTESIAN_POINT('Ctrl Pts',(-29.2846130745763,-157.356193074143,
493.537703348572));
#271637=CARTESIAN_POINT('Ctrl Pts',(-41.6688140489355,-155.051444041475,
491.537703348572));
#271638=CARTESIAN_POINT('Ctrl Pts',(-53.5400027769198,-150.837754439537,
489.537703348572));
#271639=CARTESIAN_POINT('Ctrl Pts',(-65.411191504904,-146.624064837599,
487.537703348572));
#271640=CARTESIAN_POINT('Ctrl Pts',(-76.4770599218136,-140.605189688823,
485.537703348572));
#271641=CARTESIAN_POINT('Ctrl Pts',(-87.5429283387233,-134.586314540048,
483.537703348572));
#271642=CARTESIAN_POINT('Ctrl Pts',(-97.5309980386223,-126.9104585261,481.537703348572));
#271643=CARTESIAN_POINT('Ctrl Pts',(-107.519067738521,-119.234602512152,
479.537703348572));
#271644=CARTESIAN_POINT('Ctrl Pts',(-116.183399296895,-110.0907706828,477.537703348572));
#271645=CARTESIAN_POINT('Ctrl Pts',(-124.847730855269,-100.946938853448,
475.537703348572));
#271646=CARTESIAN_POINT('Ctrl Pts',(-131.974979673883,-90.5602826949692,
473.537703348572));
#271647=CARTESIAN_POINT('Ctrl Pts',(-139.102228492497,-80.1736265364902,
471.537703348572));
#271648=CARTESIAN_POINT('Ctrl Pts',(-144.516898051454,-68.7998999948414,
469.537703348572));
#271649=CARTESIAN_POINT('Ctrl Pts',(-149.931567610412,-57.4261734531925,
467.537703348572));
#271650=CARTESIAN_POINT('Ctrl Pts',(-153.500330774912,-45.3454354230634,
465.537703348572));
#271651=CARTESIAN_POINT('Ctrl Pts',(-157.069093939413,-33.2646973929344,
463.537703348572));
#271652=CARTESIAN_POINT('Ctrl Pts',(-158.704075916301,-20.7744157382976,
461.537703348572));
#271653=CARTESIAN_POINT('Ctrl Pts',(-160.339057893189,-8.28413408366092,
459.537703348572));
#271654=CARTESIAN_POINT('Ctrl Pts',(-160.,4.30813900827803,457.537703348572));
#271655=CARTESIAN_POINT('Ctrl Pts',(-159.660942106811,16.900412100217,455.537703348572));
#271656=CARTESIAN_POINT('Ctrl Pts',(-157.356193074143,29.2846130745763,
453.537703348572));
#271657=CARTESIAN_POINT('Ctrl Pts',(-155.051444041475,41.6688140489355,
451.537703348572));
#271658=CARTESIAN_POINT('Ctrl Pts',(-150.837754439537,53.5400027769198,
449.537703348572));
#271659=CARTESIAN_POINT('Ctrl Pts',(-146.624064837599,65.411191504904,447.537703348572));
#271660=CARTESIAN_POINT('Ctrl Pts',(-140.605189688823,76.4770599218136,
445.537703348572));
#271661=CARTESIAN_POINT('Ctrl Pts',(-134.586314540048,87.5429283387233,
443.537703348572));
#271662=CARTESIAN_POINT('Ctrl Pts',(-126.9104585261,97.5309980386223,441.537703348572));
#271663=CARTESIAN_POINT('Ctrl Pts',(-119.234602512152,107.519067738521,
439.537703348572));
#271664=CARTESIAN_POINT('Ctrl Pts',(-110.0907706828,116.183399296895,437.537703348572));
#271665=CARTESIAN_POINT('Ctrl Pts',(-100.946938853448,124.847730855269,
435.537703348572));
#271666=CARTESIAN_POINT('Ctrl Pts',(-90.5602826949692,131.974979673883,
433.537703348572));
#271667=CARTESIAN_POINT('Ctrl Pts',(-80.1736265364901,139.102228492497,
431.537703348572));
#271668=CARTESIAN_POINT('Ctrl Pts',(-68.7998999948414,144.516898051454,
429.537703348572));
#271669=CARTESIAN_POINT('Ctrl Pts',(-57.4261734531926,149.931567610412,
427.537703348572));
#271670=CARTESIAN_POINT('Ctrl Pts',(-45.3454354230634,153.500330774912,
425.537703348572));
#271671=CARTESIAN_POINT('Ctrl Pts',(-33.2646973929343,157.069093939413,
423.537703348572));
#271672=CARTESIAN_POINT('Ctrl Pts',(-20.7744157382976,158.704075916301,
421.537703348572));
#271673=CARTESIAN_POINT('Ctrl Pts',(-8.284134083661,160.339057893189,419.537703348572));
#271674=CARTESIAN_POINT('Ctrl Pts',(4.30813900827803,160.,417.537703348572));
#271675=CARTESIAN_POINT('Ctrl Pts',(16.9004121002171,159.660942106811,415.537703348572));
#271676=CARTESIAN_POINT('Ctrl Pts',(29.2846130745762,157.356193074143,413.537703348572));
#271677=CARTESIAN_POINT('Ctrl Pts',(41.6688140489354,155.051444041476,411.537703348572));
#271678=CARTESIAN_POINT('Ctrl Pts',(53.5400027769198,150.837754439537,409.537703348572));
#271679=CARTESIAN_POINT('Ctrl Pts',(65.4111915049041,146.624064837599,407.537703348572));
#271680=CARTESIAN_POINT('Ctrl Pts',(76.4770599218136,140.605189688823,405.537703348572));
#271681=CARTESIAN_POINT('Ctrl Pts',(87.5429283387232,134.586314540048,403.537703348572));
#271682=CARTESIAN_POINT('Ctrl Pts',(97.5309980386223,126.9104585261,401.537703348572));
#271683=CARTESIAN_POINT('Ctrl Pts',(107.519067738521,119.234602512152,399.537703348572));
#271684=CARTESIAN_POINT('Ctrl Pts',(116.183399296895,110.0907706828,397.537703348572));
#271685=CARTESIAN_POINT('Ctrl Pts',(124.847730855269,100.946938853448,395.537703348572));
#271686=CARTESIAN_POINT('Ctrl Pts',(131.974979673883,90.5602826949692,393.537703348572));
#271687=CARTESIAN_POINT('Ctrl Pts',(139.102228492497,80.1736265364902,391.537703348572));
#271688=CARTESIAN_POINT('Ctrl Pts',(144.516898051454,68.7998999948414,389.537703348572));
#271689=CARTESIAN_POINT('Ctrl Pts',(149.931567610412,57.4261734531926,387.537703348572));
#271690=CARTESIAN_POINT('Ctrl Pts',(153.500330774912,45.3454354230634,385.537703348572));
#271691=CARTESIAN_POINT('Ctrl Pts',(157.069093939413,33.2646973929343,383.537703348572));
#271692=CARTESIAN_POINT('Ctrl Pts',(158.704075916301,20.7744157382976,381.537703348572));
#271693=CARTESIAN_POINT('Ctrl Pts',(160.339057893189,8.28413408366101,379.537703348572));
#271694=CARTESIAN_POINT('Ctrl Pts',(160.,-4.30813900827805,377.537703348572));
#271695=CARTESIAN_POINT('Origin',(160.,3.64291929955129E-14,535.));
#271696=CARTESIAN_POINT('',(160.,4.30813900827813,532.462296651428));
#271697=CARTESIAN_POINT('',(160.,-2.95752061042501E-13,535.));
#271698=CARTESIAN_POINT('',(160.,3.64291929955129E-14,535.));
#271699=CARTESIAN_POINT('',(160.,-4.30813900827846,531.09188778474));
#271700=CARTESIAN_POINT('Ctrl Pts',(160.,-4.30813900827846,531.09188778474));
#271701=CARTESIAN_POINT('Ctrl Pts',(160.,-1.43604209808346,531.54866409354));
#271702=CARTESIAN_POINT('Ctrl Pts',(160.,1.43594781991679,532.006113535419));
#271703=CARTESIAN_POINT('Ctrl Pts',(160.,4.30813900827813,532.462296651428));
#271704=CARTESIAN_POINT('Ctrl Pts',(160.,-2.96429547574917E-13,535.));
#271705=CARTESIAN_POINT('Ctrl Pts',(160.,-0.0199151703857166,534.98194265546));
#271706=CARTESIAN_POINT('Ctrl Pts',(160.,-0.039830432386428,534.96388541196));
#271707=CARTESIAN_POINT('Ctrl Pts',(160.,-0.0597455111566523,534.94582796638));
#271708=CARTESIAN_POINT('Ctrl Pts',(160.,-1.47617978783616,533.66151545298));
#271709=CARTESIAN_POINT('Ctrl Pts',(160.,-2.89215276710073,532.376694251498));
#271710=CARTESIAN_POINT('Ctrl Pts',(160.,-4.30813900827846,531.09188778474));
#271711=CARTESIAN_POINT('',(160.,-4.30813900827805,537.537703348572));
#271712=CARTESIAN_POINT('',(160.,3.64291929955129E-14,535.));
#271713=CARTESIAN_POINT('',(160.,4.30813900825421,538.908112215256));
#271714=CARTESIAN_POINT('Ctrl Pts',(160.,-4.30813900827805,537.537703348572));
#271715=CARTESIAN_POINT('Ctrl Pts',(160.,-1.43594781992483,537.99388646458));
#271716=CARTESIAN_POINT('Ctrl Pts',(160.,1.4360420980673,538.451335906457));
#271717=CARTESIAN_POINT('Ctrl Pts',(160.,4.30813900825421,538.908112215256));
#271718=CARTESIAN_POINT('Ctrl Pts',(160.000000000001,4.30813900825419,538.908112215256));
#271719=CARTESIAN_POINT('Ctrl Pts',(160.,2.89215276709868,537.623305748502));
#271720=CARTESIAN_POINT('Ctrl Pts',(160.,1.47617978787219,536.338484546979));
#271721=CARTESIAN_POINT('Ctrl Pts',(160.,0.0597455111551169,535.054172033622));
#271722=CARTESIAN_POINT('Ctrl Pts',(160.,0.0398304323843582,535.036114588042));
#271723=CARTESIAN_POINT('Ctrl Pts',(160.,0.0199151703848928,535.018057344541));
#271724=CARTESIAN_POINT('Ctrl Pts',(160.,-3.06976666308856E-13,535.));
#271725=CARTESIAN_POINT('Ctrl Pts',(160.,-4.30813900827805,697.537703348572));
#271726=CARTESIAN_POINT('Ctrl Pts',(159.660942106811,-16.900412100217,695.537703348572));
#271727=CARTESIAN_POINT('Ctrl Pts',(157.356193074143,-29.2846130745763,
693.537703348572));
#271728=CARTESIAN_POINT('Ctrl Pts',(155.051444041475,-41.6688140489355,
691.537703348572));
#271729=CARTESIAN_POINT('Ctrl Pts',(150.837754439537,-53.5400027769198,
689.537703348572));
#271730=CARTESIAN_POINT('Ctrl Pts',(146.624064837599,-65.411191504904,687.537703348572));
#271731=CARTESIAN_POINT('Ctrl Pts',(140.605189688823,-76.4770599218136,
685.537703348572));
#271732=CARTESIAN_POINT('Ctrl Pts',(134.586314540048,-87.5429283387233,
683.537703348572));
#271733=CARTESIAN_POINT('Ctrl Pts',(126.9104585261,-97.5309980386223,681.537703348572));
#271734=CARTESIAN_POINT('Ctrl Pts',(119.234602512152,-107.519067738521,
679.537703348572));
#271735=CARTESIAN_POINT('Ctrl Pts',(110.0907706828,-116.183399296895,677.537703348572));
#271736=CARTESIAN_POINT('Ctrl Pts',(100.946938853448,-124.847730855269,
675.537703348572));
#271737=CARTESIAN_POINT('Ctrl Pts',(90.5602826949691,-131.974979673883,
673.537703348572));
#271738=CARTESIAN_POINT('Ctrl Pts',(80.1736265364902,-139.102228492497,
671.537703348572));
#271739=CARTESIAN_POINT('Ctrl Pts',(68.7998999948414,-144.516898051454,
669.537703348572));
#271740=CARTESIAN_POINT('Ctrl Pts',(57.4261734531925,-149.931567610412,
667.537703348572));
#271741=CARTESIAN_POINT('Ctrl Pts',(45.3454354230634,-153.500330774912,
665.537703348572));
#271742=CARTESIAN_POINT('Ctrl Pts',(33.2646973929343,-157.069093939413,
663.537703348572));
#271743=CARTESIAN_POINT('Ctrl Pts',(20.7744157382976,-158.704075916301,
661.537703348572));
#271744=CARTESIAN_POINT('Ctrl Pts',(8.28413408366091,-160.339057893189,
659.537703348572));
#271745=CARTESIAN_POINT('Ctrl Pts',(-4.30813900827804,-160.,657.537703348572));
#271746=CARTESIAN_POINT('Ctrl Pts',(-16.900412100217,-159.660942106811,
655.537703348572));
#271747=CARTESIAN_POINT('Ctrl Pts',(-29.2846130745763,-157.356193074143,
653.537703348572));
#271748=CARTESIAN_POINT('Ctrl Pts',(-41.6688140489355,-155.051444041475,
651.537703348572));
#271749=CARTESIAN_POINT('Ctrl Pts',(-53.5400027769198,-150.837754439537,
649.537703348572));
#271750=CARTESIAN_POINT('Ctrl Pts',(-65.411191504904,-146.624064837599,
647.537703348572));
#271751=CARTESIAN_POINT('Ctrl Pts',(-76.4770599218136,-140.605189688823,
645.537703348572));
#271752=CARTESIAN_POINT('Ctrl Pts',(-87.5429283387233,-134.586314540048,
643.537703348572));
#271753=CARTESIAN_POINT('Ctrl Pts',(-97.5309980386223,-126.9104585261,641.537703348572));
#271754=CARTESIAN_POINT('Ctrl Pts',(-107.519067738521,-119.234602512152,
639.537703348572));
#271755=CARTESIAN_POINT('Ctrl Pts',(-116.183399296895,-110.0907706828,637.537703348572));
#271756=CARTESIAN_POINT('Ctrl Pts',(-124.847730855269,-100.946938853448,
635.537703348572));
#271757=CARTESIAN_POINT('Ctrl Pts',(-131.974979673883,-90.5602826949692,
633.537703348572));
#271758=CARTESIAN_POINT('Ctrl Pts',(-139.102228492497,-80.1736265364902,
631.537703348572));
#271759=CARTESIAN_POINT('Ctrl Pts',(-144.516898051454,-68.7998999948414,
629.537703348572));
#271760=CARTESIAN_POINT('Ctrl Pts',(-149.931567610412,-57.4261734531925,
627.537703348572));
#271761=CARTESIAN_POINT('Ctrl Pts',(-153.500330774912,-45.3454354230634,
625.537703348572));
#271762=CARTESIAN_POINT('Ctrl Pts',(-157.069093939413,-33.2646973929344,
623.537703348572));
#271763=CARTESIAN_POINT('Ctrl Pts',(-158.704075916301,-20.7744157382976,
621.537703348572));
#271764=CARTESIAN_POINT('Ctrl Pts',(-160.339057893189,-8.28413408366092,
619.537703348572));
#271765=CARTESIAN_POINT('Ctrl Pts',(-160.,4.30813900827803,617.537703348572));
#271766=CARTESIAN_POINT('Ctrl Pts',(-159.660942106811,16.900412100217,615.537703348572));
#271767=CARTESIAN_POINT('Ctrl Pts',(-157.356193074143,29.2846130745763,
613.537703348572));
#271768=CARTESIAN_POINT('Ctrl Pts',(-155.051444041475,41.6688140489355,
611.537703348572));
#271769=CARTESIAN_POINT('Ctrl Pts',(-150.837754439537,53.5400027769198,
609.537703348572));
#271770=CARTESIAN_POINT('Ctrl Pts',(-146.624064837599,65.411191504904,607.537703348572));
#271771=CARTESIAN_POINT('Ctrl Pts',(-140.605189688823,76.4770599218136,
605.537703348572));
#271772=CARTESIAN_POINT('Ctrl Pts',(-134.586314540048,87.5429283387233,
603.537703348572));
#271773=CARTESIAN_POINT('Ctrl Pts',(-126.9104585261,97.5309980386223,601.537703348572));
#271774=CARTESIAN_POINT('Ctrl Pts',(-119.234602512152,107.519067738521,
599.537703348572));
#271775=CARTESIAN_POINT('Ctrl Pts',(-110.0907706828,116.183399296895,597.537703348572));
#271776=CARTESIAN_POINT('Ctrl Pts',(-100.946938853448,124.847730855269,
595.537703348572));
#271777=CARTESIAN_POINT('Ctrl Pts',(-90.5602826949692,131.974979673883,
593.537703348572));
#271778=CARTESIAN_POINT('Ctrl Pts',(-80.1736265364901,139.102228492497,
591.537703348572));
#271779=CARTESIAN_POINT('Ctrl Pts',(-68.7998999948414,144.516898051454,
589.537703348572));
#271780=CARTESIAN_POINT('Ctrl Pts',(-57.4261734531926,149.931567610412,
587.537703348572));
#271781=CARTESIAN_POINT('Ctrl Pts',(-45.3454354230634,153.500330774912,
585.537703348572));
#271782=CARTESIAN_POINT('Ctrl Pts',(-33.2646973929343,157.069093939413,
583.537703348572));
#271783=CARTESIAN_POINT('Ctrl Pts',(-20.7744157382976,158.704075916301,
581.537703348572));
#271784=CARTESIAN_POINT('Ctrl Pts',(-8.284134083661,160.339057893189,579.537703348572));
#271785=CARTESIAN_POINT('Ctrl Pts',(4.30813900827803,160.,577.537703348572));
#271786=CARTESIAN_POINT('Ctrl Pts',(16.9004121002171,159.660942106811,575.537703348572));
#271787=CARTESIAN_POINT('Ctrl Pts',(29.2846130745762,157.356193074143,573.537703348572));
#271788=CARTESIAN_POINT('Ctrl Pts',(41.6688140489354,155.051444041476,571.537703348572));
#271789=CARTESIAN_POINT('Ctrl Pts',(53.5400027769198,150.837754439537,569.537703348572));
#271790=CARTESIAN_POINT('Ctrl Pts',(65.4111915049041,146.624064837599,567.537703348572));
#271791=CARTESIAN_POINT('Ctrl Pts',(76.4770599218136,140.605189688823,565.537703348572));
#271792=CARTESIAN_POINT('Ctrl Pts',(87.5429283387232,134.586314540048,563.537703348572));
#271793=CARTESIAN_POINT('Ctrl Pts',(97.5309980386223,126.9104585261,561.537703348572));
#271794=CARTESIAN_POINT('Ctrl Pts',(107.519067738521,119.234602512152,559.537703348572));
#271795=CARTESIAN_POINT('Ctrl Pts',(116.183399296895,110.0907706828,557.537703348572));
#271796=CARTESIAN_POINT('Ctrl Pts',(124.847730855269,100.946938853448,555.537703348572));
#271797=CARTESIAN_POINT('Ctrl Pts',(131.974979673883,90.5602826949692,553.537703348572));
#271798=CARTESIAN_POINT('Ctrl Pts',(139.102228492497,80.1736265364902,551.537703348572));
#271799=CARTESIAN_POINT('Ctrl Pts',(144.516898051454,68.7998999948414,549.537703348572));
#271800=CARTESIAN_POINT('Ctrl Pts',(149.931567610412,57.4261734531926,547.537703348572));
#271801=CARTESIAN_POINT('Ctrl Pts',(153.500330774912,45.3454354230634,545.537703348572));
#271802=CARTESIAN_POINT('Ctrl Pts',(157.069093939413,33.2646973929343,543.537703348572));
#271803=CARTESIAN_POINT('Ctrl Pts',(158.704075916301,20.7744157382976,541.537703348572));
#271804=CARTESIAN_POINT('Ctrl Pts',(160.339057893189,8.28413408366101,539.537703348572));
#271805=CARTESIAN_POINT('Ctrl Pts',(160.,-4.30813900827805,537.537703348572));
#271806=CARTESIAN_POINT('Ctrl Pts',(130.,-4.30813900827807,697.537703348572));
#271807=CARTESIAN_POINT('Ctrl Pts',(129.660942106811,-14.5393608954785,
695.537703348572));
#271808=CARTESIAN_POINT('Ctrl Pts',(127.725542856289,-24.5915791233694,
693.537703348572));
#271809=CARTESIAN_POINT('Ctrl Pts',(125.790143605767,-34.6437973512603,
691.537703348572));
#271810=CARTESIAN_POINT('Ctrl Pts',(122.306058950682,-44.2694929456714,
689.537703348572));
#271811=CARTESIAN_POINT('Ctrl Pts',(118.821974295598,-53.8951885400825,
687.537703348572));
#271812=CARTESIAN_POINT('Ctrl Pts',(113.874993963172,-62.8573449296272,
685.537703348572));
#271813=CARTESIAN_POINT('Ctrl Pts',(108.928013630747,-71.819501319172,683.537703348572));
#271814=CARTESIAN_POINT('Ctrl Pts',(102.639948694851,-79.8974404698481,
681.537703348572));
#271815=CARTESIAN_POINT('Ctrl Pts',(96.351883758956,-87.9753796205242,679.537703348572));
#271816=CARTESIAN_POINT('Ctrl Pts',(88.8775672472035,-94.9701958612989,
677.537703348572));
#271817=CARTESIAN_POINT('Ctrl Pts',(81.403250735451,-101.965012102074,675.537703348572));
#271818=CARTESIAN_POINT('Ctrl Pts',(72.9267251261949,-107.704469842635,
673.537703348572));
#271819=CARTESIAN_POINT('Ctrl Pts',(64.4501995169389,-113.443927583196,
671.537703348572));
#271820=CARTESIAN_POINT('Ctrl Pts',(55.1801850026549,-117.786702325803,
669.537703348572));
#271821=CARTESIAN_POINT('Ctrl Pts',(45.910170488371,-122.129477068411,667.537703348572));
#271822=CARTESIAN_POINT('Ctrl Pts',(36.074925591815,-124.968635286058,665.537703348572));
#271823=CARTESIAN_POINT('Ctrl Pts',(26.239680695259,-127.807793503704,663.537703348572));
#271824=CARTESIAN_POINT('Ctrl Pts',(16.0813817870907,-129.073425698447,
661.537703348572));
#271825=CARTESIAN_POINT('Ctrl Pts',(5.92308287892234,-130.339057893189,
659.537703348572));
#271826=CARTESIAN_POINT('Ctrl Pts',(-4.30813900827806,-130.,657.537703348572));
#271827=CARTESIAN_POINT('Ctrl Pts',(-14.5393608954785,-129.660942106811,
655.537703348572));
#271828=CARTESIAN_POINT('Ctrl Pts',(-24.5915791233694,-127.725542856289,
653.537703348572));
#271829=CARTESIAN_POINT('Ctrl Pts',(-34.6437973512603,-125.790143605767,
651.537703348572));
#271830=CARTESIAN_POINT('Ctrl Pts',(-44.2694929456713,-122.306058950682,
649.537703348572));
#271831=CARTESIAN_POINT('Ctrl Pts',(-53.8951885400825,-118.821974295598,
647.537703348572));
#271832=CARTESIAN_POINT('Ctrl Pts',(-62.8573449296272,-113.874993963172,
645.537703348572));
#271833=CARTESIAN_POINT('Ctrl Pts',(-71.819501319172,-108.928013630747,
643.537703348572));
#271834=CARTESIAN_POINT('Ctrl Pts',(-79.8974404698481,-102.639948694851,
641.537703348572));
#271835=CARTESIAN_POINT('Ctrl Pts',(-87.9753796205242,-96.351883758956,
639.537703348572));
#271836=CARTESIAN_POINT('Ctrl Pts',(-94.9701958612989,-88.8775672472035,
637.537703348572));
#271837=CARTESIAN_POINT('Ctrl Pts',(-101.965012102074,-81.403250735451,
635.537703348572));
#271838=CARTESIAN_POINT('Ctrl Pts',(-107.704469842635,-72.9267251261949,
633.537703348572));
#271839=CARTESIAN_POINT('Ctrl Pts',(-113.443927583196,-64.4501995169389,
631.537703348572));
#271840=CARTESIAN_POINT('Ctrl Pts',(-117.786702325803,-55.1801850026549,
629.537703348572));
#271841=CARTESIAN_POINT('Ctrl Pts',(-122.129477068411,-45.910170488371,
627.537703348572));
#271842=CARTESIAN_POINT('Ctrl Pts',(-124.968635286058,-36.074925591815,
625.537703348572));
#271843=CARTESIAN_POINT('Ctrl Pts',(-127.807793503704,-26.239680695259,
623.537703348572));
#271844=CARTESIAN_POINT('Ctrl Pts',(-129.073425698447,-16.0813817870907,
621.537703348572));
#271845=CARTESIAN_POINT('Ctrl Pts',(-130.339057893189,-5.92308287892235,
619.537703348572));
#271846=CARTESIAN_POINT('Ctrl Pts',(-130.,4.30813900827805,617.537703348572));
#271847=CARTESIAN_POINT('Ctrl Pts',(-129.660942106811,14.5393608954784,
615.537703348572));
#271848=CARTESIAN_POINT('Ctrl Pts',(-127.725542856289,24.5915791233693,
613.537703348572));
#271849=CARTESIAN_POINT('Ctrl Pts',(-125.790143605767,34.6437973512602,
611.537703348572));
#271850=CARTESIAN_POINT('Ctrl Pts',(-122.306058950682,44.2694929456713,
609.537703348572));
#271851=CARTESIAN_POINT('Ctrl Pts',(-118.821974295598,53.8951885400825,
607.537703348572));
#271852=CARTESIAN_POINT('Ctrl Pts',(-113.874993963172,62.8573449296272,
605.537703348572));
#271853=CARTESIAN_POINT('Ctrl Pts',(-108.928013630747,71.819501319172,603.537703348572));
#271854=CARTESIAN_POINT('Ctrl Pts',(-102.639948694851,79.8974404698481,
601.537703348572));
#271855=CARTESIAN_POINT('Ctrl Pts',(-96.3518837589561,87.9753796205242,
599.537703348572));
#271856=CARTESIAN_POINT('Ctrl Pts',(-88.8775672472035,94.9701958612989,
597.537703348572));
#271857=CARTESIAN_POINT('Ctrl Pts',(-81.403250735451,101.965012102074,595.537703348572));
#271858=CARTESIAN_POINT('Ctrl Pts',(-72.9267251261949,107.704469842635,
593.537703348572));
#271859=CARTESIAN_POINT('Ctrl Pts',(-64.4501995169389,113.443927583196,
591.537703348572));
#271860=CARTESIAN_POINT('Ctrl Pts',(-55.1801850026549,117.786702325803,
589.537703348572));
#271861=CARTESIAN_POINT('Ctrl Pts',(-45.910170488371,122.129477068411,587.537703348572));
#271862=CARTESIAN_POINT('Ctrl Pts',(-36.074925591815,124.968635286058,585.537703348572));
#271863=CARTESIAN_POINT('Ctrl Pts',(-26.239680695259,127.807793503704,583.537703348572));
#271864=CARTESIAN_POINT('Ctrl Pts',(-16.0813817870907,129.073425698447,
581.537703348572));
#271865=CARTESIAN_POINT('Ctrl Pts',(-5.92308287892242,130.339057893189,
579.537703348572));
#271866=CARTESIAN_POINT('Ctrl Pts',(4.30813900827804,130.,577.537703348572));
#271867=CARTESIAN_POINT('Ctrl Pts',(14.5393608954785,129.660942106811,575.537703348572));
#271868=CARTESIAN_POINT('Ctrl Pts',(24.5915791233693,127.725542856289,573.537703348572));
#271869=CARTESIAN_POINT('Ctrl Pts',(34.6437973512602,125.790143605767,571.537703348572));
#271870=CARTESIAN_POINT('Ctrl Pts',(44.2694929456713,122.306058950682,569.537703348572));
#271871=CARTESIAN_POINT('Ctrl Pts',(53.8951885400825,118.821974295598,567.537703348572));
#271872=CARTESIAN_POINT('Ctrl Pts',(62.8573449296272,113.874993963172,565.537703348572));
#271873=CARTESIAN_POINT('Ctrl Pts',(71.819501319172,108.928013630747,563.537703348572));
#271874=CARTESIAN_POINT('Ctrl Pts',(79.8974404698481,102.639948694851,561.537703348572));
#271875=CARTESIAN_POINT('Ctrl Pts',(87.9753796205242,96.351883758956,559.537703348572));
#271876=CARTESIAN_POINT('Ctrl Pts',(94.9701958612989,88.8775672472035,557.537703348572));
#271877=CARTESIAN_POINT('Ctrl Pts',(101.965012102074,81.403250735451,555.537703348572));
#271878=CARTESIAN_POINT('Ctrl Pts',(107.704469842635,72.926725126195,553.537703348572));
#271879=CARTESIAN_POINT('Ctrl Pts',(113.443927583196,64.4501995169389,551.537703348572));
#271880=CARTESIAN_POINT('Ctrl Pts',(117.786702325803,55.1801850026549,549.537703348572));
#271881=CARTESIAN_POINT('Ctrl Pts',(122.129477068411,45.910170488371,547.537703348572));
#271882=CARTESIAN_POINT('Ctrl Pts',(124.968635286058,36.074925591815,545.537703348572));
#271883=CARTESIAN_POINT('Ctrl Pts',(127.807793503704,26.239680695259,543.537703348572));
#271884=CARTESIAN_POINT('Ctrl Pts',(129.073425698447,16.0813817870907,541.537703348572));
#271885=CARTESIAN_POINT('Ctrl Pts',(130.339057893189,5.92308287892242,539.537703348572));
#271886=CARTESIAN_POINT('Ctrl Pts',(130.,-4.30813900827807,537.537703348572));
#271887=CARTESIAN_POINT('Origin',(-4.03737035466399,-0.209103844047687,
539.537622607813));
#271888=CARTESIAN_POINT('Ctrl Pts',(160.,4.30813900827813,692.462296651428));
#271889=CARTESIAN_POINT('Ctrl Pts',(160.339057893189,-8.28413408366083,
690.462296651428));
#271890=CARTESIAN_POINT('Ctrl Pts',(158.704075916301,-20.7744157382975,
688.462296651428));
#271891=CARTESIAN_POINT('Ctrl Pts',(157.069093939413,-33.2646973929343,
686.462296651429));
#271892=CARTESIAN_POINT('Ctrl Pts',(153.500330774912,-45.3454354230633,
684.462296651428));
#271893=CARTESIAN_POINT('Ctrl Pts',(149.931567610412,-57.4261734531924,
682.462296651428));
#271894=CARTESIAN_POINT('Ctrl Pts',(144.516898051455,-68.7998999948413,
680.462296651428));
#271895=CARTESIAN_POINT('Ctrl Pts',(139.102228492497,-80.1736265364901,
678.462296651428));
#271896=CARTESIAN_POINT('Ctrl Pts',(131.974979673883,-90.5602826949691,
676.462296651428));
#271897=CARTESIAN_POINT('Ctrl Pts',(124.847730855269,-100.946938853448,
674.462296651428));
#271898=CARTESIAN_POINT('Ctrl Pts',(116.183399296895,-110.0907706828,672.462296651428));
#271899=CARTESIAN_POINT('Ctrl Pts',(107.519067738521,-119.234602512152,
670.462296651428));
#271900=CARTESIAN_POINT('Ctrl Pts',(97.5309980386224,-126.9104585261,668.462296651428));
#271901=CARTESIAN_POINT('Ctrl Pts',(87.5429283387234,-134.586314540048,
666.462296651428));
#271902=CARTESIAN_POINT('Ctrl Pts',(76.4770599218137,-140.605189688823,
664.462296651428));
#271903=CARTESIAN_POINT('Ctrl Pts',(65.4111915049041,-146.624064837599,
662.462296651428));
#271904=CARTESIAN_POINT('Ctrl Pts',(53.5400027769198,-150.837754439537,
660.462296651428));
#271905=CARTESIAN_POINT('Ctrl Pts',(41.6688140489356,-155.051444041475,
658.462296651428));
#271906=CARTESIAN_POINT('Ctrl Pts',(29.2846130745764,-157.356193074143,
656.462296651428));
#271907=CARTESIAN_POINT('Ctrl Pts',(16.9004121002171,-159.660942106811,
654.462296651428));
#271908=CARTESIAN_POINT('Ctrl Pts',(4.30813900827814,-160.,652.462296651428));
#271909=CARTESIAN_POINT('Ctrl Pts',(-8.28413408366082,-160.339057893189,
650.462296651428));
#271910=CARTESIAN_POINT('Ctrl Pts',(-20.7744157382975,-158.704075916301,
648.462296651428));
#271911=CARTESIAN_POINT('Ctrl Pts',(-33.2646973929342,-157.069093939413,
646.462296651428));
#271912=CARTESIAN_POINT('Ctrl Pts',(-45.3454354230633,-153.500330774912,
644.462296651428));
#271913=CARTESIAN_POINT('Ctrl Pts',(-57.4261734531924,-149.931567610412,
642.462296651428));
#271914=CARTESIAN_POINT('Ctrl Pts',(-68.7998999948413,-144.516898051455,
640.462296651428));
#271915=CARTESIAN_POINT('Ctrl Pts',(-80.1736265364901,-139.102228492497,
638.462296651428));
#271916=CARTESIAN_POINT('Ctrl Pts',(-90.5602826949691,-131.974979673883,
636.462296651428));
#271917=CARTESIAN_POINT('Ctrl Pts',(-100.946938853448,-124.847730855269,
634.462296651428));
#271918=CARTESIAN_POINT('Ctrl Pts',(-110.0907706828,-116.183399296895,632.462296651428));
#271919=CARTESIAN_POINT('Ctrl Pts',(-119.234602512152,-107.519067738521,
630.462296651428));
#271920=CARTESIAN_POINT('Ctrl Pts',(-126.9104585261,-97.5309980386224,628.462296651428));
#271921=CARTESIAN_POINT('Ctrl Pts',(-134.586314540048,-87.5429283387234,
626.462296651429));
#271922=CARTESIAN_POINT('Ctrl Pts',(-140.605189688823,-76.4770599218137,
624.462296651428));
#271923=CARTESIAN_POINT('Ctrl Pts',(-146.624064837599,-65.4111915049041,
622.462296651428));
#271924=CARTESIAN_POINT('Ctrl Pts',(-150.837754439537,-53.5400027769199,
620.462296651428));
#271925=CARTESIAN_POINT('Ctrl Pts',(-155.051444041475,-41.6688140489356,
618.462296651428));
#271926=CARTESIAN_POINT('Ctrl Pts',(-157.356193074143,-29.2846130745764,
616.462296651428));
#271927=CARTESIAN_POINT('Ctrl Pts',(-159.660942106811,-16.9004121002171,
614.462296651429));
#271928=CARTESIAN_POINT('Ctrl Pts',(-160.,-4.30813900827815,612.462296651428));
#271929=CARTESIAN_POINT('Ctrl Pts',(-160.339057893189,8.28413408366081,
610.462296651428));
#271930=CARTESIAN_POINT('Ctrl Pts',(-158.704075916301,20.7744157382975,
608.462296651428));
#271931=CARTESIAN_POINT('Ctrl Pts',(-157.069093939413,33.2646973929342,
606.462296651428));
#271932=CARTESIAN_POINT('Ctrl Pts',(-153.500330774912,45.3454354230633,
604.462296651428));
#271933=CARTESIAN_POINT('Ctrl Pts',(-149.931567610412,57.4261734531924,
602.462296651429));
#271934=CARTESIAN_POINT('Ctrl Pts',(-144.516898051455,68.7998999948413,
600.462296651428));
#271935=CARTESIAN_POINT('Ctrl Pts',(-139.102228492497,80.1736265364901,
598.462296651428));
#271936=CARTESIAN_POINT('Ctrl Pts',(-131.974979673883,90.5602826949691,
596.462296651428));
#271937=CARTESIAN_POINT('Ctrl Pts',(-124.847730855269,100.946938853448,
594.462296651428));
#271938=CARTESIAN_POINT('Ctrl Pts',(-116.183399296895,110.0907706828,592.462296651428));
#271939=CARTESIAN_POINT('Ctrl Pts',(-107.519067738521,119.234602512152,
590.462296651428));
#271940=CARTESIAN_POINT('Ctrl Pts',(-97.5309980386224,126.9104585261,588.462296651428));
#271941=CARTESIAN_POINT('Ctrl Pts',(-87.5429283387233,134.586314540048,
586.462296651428));
#271942=CARTESIAN_POINT('Ctrl Pts',(-76.4770599218137,140.605189688823,
584.462296651428));
#271943=CARTESIAN_POINT('Ctrl Pts',(-65.4111915049042,146.624064837599,
582.462296651428));
#271944=CARTESIAN_POINT('Ctrl Pts',(-53.5400027769199,150.837754439537,
580.462296651428));
#271945=CARTESIAN_POINT('Ctrl Pts',(-41.6688140489356,155.051444041475,
578.462296651428));
#271946=CARTESIAN_POINT('Ctrl Pts',(-29.2846130745764,157.356193074143,
576.462296651428));
#271947=CARTESIAN_POINT('Ctrl Pts',(-16.9004121002172,159.660942106811,
574.462296651428));
#271948=CARTESIAN_POINT('Ctrl Pts',(-4.30813900827816,160.,572.462296651428));
#271949=CARTESIAN_POINT('Ctrl Pts',(8.28413408366087,160.339057893189,570.462296651428));
#271950=CARTESIAN_POINT('Ctrl Pts',(20.7744157382975,158.704075916301,568.462296651428));
#271951=CARTESIAN_POINT('Ctrl Pts',(33.2646973929342,157.069093939413,566.462296651428));
#271952=CARTESIAN_POINT('Ctrl Pts',(45.3454354230633,153.500330774912,564.462296651428));
#271953=CARTESIAN_POINT('Ctrl Pts',(57.4261734531925,149.931567610412,562.462296651428));
#271954=CARTESIAN_POINT('Ctrl Pts',(68.7998999948413,144.516898051455,560.462296651428));
#271955=CARTESIAN_POINT('Ctrl Pts',(80.1736265364901,139.102228492498,558.462296651428));
#271956=CARTESIAN_POINT('Ctrl Pts',(90.560282694969,131.974979673883,556.462296651428));
#271957=CARTESIAN_POINT('Ctrl Pts',(100.946938853448,124.847730855269,554.462296651428));
#271958=CARTESIAN_POINT('Ctrl Pts',(110.0907706828,116.183399296895,552.462296651428));
#271959=CARTESIAN_POINT('Ctrl Pts',(119.234602512152,107.519067738521,550.462296651428));
#271960=CARTESIAN_POINT('Ctrl Pts',(126.9104585261,97.5309980386224,548.462296651428));
#271961=CARTESIAN_POINT('Ctrl Pts',(134.586314540048,87.5429283387233,546.462296651428));
#271962=CARTESIAN_POINT('Ctrl Pts',(140.605189688823,76.4770599218137,544.462296651428));
#271963=CARTESIAN_POINT('Ctrl Pts',(146.624064837599,65.4111915049042,542.462296651428));
#271964=CARTESIAN_POINT('Ctrl Pts',(150.837754439537,53.5400027769199,540.462296651428));
#271965=CARTESIAN_POINT('Ctrl Pts',(155.051444041475,41.6688140489356,538.462296651428));
#271966=CARTESIAN_POINT('Ctrl Pts',(157.356193074143,29.2846130745764,536.462296651428));
#271967=CARTESIAN_POINT('Ctrl Pts',(159.660942106811,16.9004121002172,534.462296651428));
#271968=CARTESIAN_POINT('Ctrl Pts',(160.,4.30813900827813,532.462296651428));
#271969=CARTESIAN_POINT('Ctrl Pts',(160.,-4.30813900827805,697.537703348572));
#271970=CARTESIAN_POINT('Ctrl Pts',(159.660942106811,-16.900412100217,695.537703348572));
#271971=CARTESIAN_POINT('Ctrl Pts',(157.356193074143,-29.2846130745763,
693.537703348572));
#271972=CARTESIAN_POINT('Ctrl Pts',(155.051444041475,-41.6688140489355,
691.537703348572));
#271973=CARTESIAN_POINT('Ctrl Pts',(150.837754439537,-53.5400027769198,
689.537703348572));
#271974=CARTESIAN_POINT('Ctrl Pts',(146.624064837599,-65.411191504904,687.537703348572));
#271975=CARTESIAN_POINT('Ctrl Pts',(140.605189688823,-76.4770599218136,
685.537703348572));
#271976=CARTESIAN_POINT('Ctrl Pts',(134.586314540048,-87.5429283387233,
683.537703348572));
#271977=CARTESIAN_POINT('Ctrl Pts',(126.9104585261,-97.5309980386223,681.537703348572));
#271978=CARTESIAN_POINT('Ctrl Pts',(119.234602512152,-107.519067738521,
679.537703348572));
#271979=CARTESIAN_POINT('Ctrl Pts',(110.0907706828,-116.183399296895,677.537703348572));
#271980=CARTESIAN_POINT('Ctrl Pts',(100.946938853448,-124.847730855269,
675.537703348572));
#271981=CARTESIAN_POINT('Ctrl Pts',(90.5602826949691,-131.974979673883,
673.537703348572));
#271982=CARTESIAN_POINT('Ctrl Pts',(80.1736265364902,-139.102228492497,
671.537703348572));
#271983=CARTESIAN_POINT('Ctrl Pts',(68.7998999948414,-144.516898051454,
669.537703348572));
#271984=CARTESIAN_POINT('Ctrl Pts',(57.4261734531925,-149.931567610412,
667.537703348572));
#271985=CARTESIAN_POINT('Ctrl Pts',(45.3454354230634,-153.500330774912,
665.537703348572));
#271986=CARTESIAN_POINT('Ctrl Pts',(33.2646973929343,-157.069093939413,
663.537703348572));
#271987=CARTESIAN_POINT('Ctrl Pts',(20.7744157382976,-158.704075916301,
661.537703348572));
#271988=CARTESIAN_POINT('Ctrl Pts',(8.28413408366091,-160.339057893189,
659.537703348572));
#271989=CARTESIAN_POINT('Ctrl Pts',(-4.30813900827804,-160.,657.537703348572));
#271990=CARTESIAN_POINT('Ctrl Pts',(-16.900412100217,-159.660942106811,
655.537703348572));
#271991=CARTESIAN_POINT('Ctrl Pts',(-29.2846130745763,-157.356193074143,
653.537703348572));
#271992=CARTESIAN_POINT('Ctrl Pts',(-41.6688140489355,-155.051444041475,
651.537703348572));
#271993=CARTESIAN_POINT('Ctrl Pts',(-53.5400027769198,-150.837754439537,
649.537703348572));
#271994=CARTESIAN_POINT('Ctrl Pts',(-65.411191504904,-146.624064837599,
647.537703348572));
#271995=CARTESIAN_POINT('Ctrl Pts',(-76.4770599218136,-140.605189688823,
645.537703348572));
#271996=CARTESIAN_POINT('Ctrl Pts',(-87.5429283387233,-134.586314540048,
643.537703348572));
#271997=CARTESIAN_POINT('Ctrl Pts',(-97.5309980386223,-126.9104585261,641.537703348572));
#271998=CARTESIAN_POINT('Ctrl Pts',(-107.519067738521,-119.234602512152,
639.537703348572));
#271999=CARTESIAN_POINT('Ctrl Pts',(-116.183399296895,-110.0907706828,637.537703348572));
#272000=CARTESIAN_POINT('Ctrl Pts',(-124.847730855269,-100.946938853448,
635.537703348572));
#272001=CARTESIAN_POINT('Ctrl Pts',(-131.974979673883,-90.5602826949692,
633.537703348572));
#272002=CARTESIAN_POINT('Ctrl Pts',(-139.102228492497,-80.1736265364902,
631.537703348572));
#272003=CARTESIAN_POINT('Ctrl Pts',(-144.516898051454,-68.7998999948414,
629.537703348572));
#272004=CARTESIAN_POINT('Ctrl Pts',(-149.931567610412,-57.4261734531925,
627.537703348572));
#272005=CARTESIAN_POINT('Ctrl Pts',(-153.500330774912,-45.3454354230634,
625.537703348572));
#272006=CARTESIAN_POINT('Ctrl Pts',(-157.069093939413,-33.2646973929344,
623.537703348572));
#272007=CARTESIAN_POINT('Ctrl Pts',(-158.704075916301,-20.7744157382976,
621.537703348572));
#272008=CARTESIAN_POINT('Ctrl Pts',(-160.339057893189,-8.28413408366092,
619.537703348572));
#272009=CARTESIAN_POINT('Ctrl Pts',(-160.,4.30813900827803,617.537703348572));
#272010=CARTESIAN_POINT('Ctrl Pts',(-159.660942106811,16.900412100217,615.537703348572));
#272011=CARTESIAN_POINT('Ctrl Pts',(-157.356193074143,29.2846130745763,
613.537703348572));
#272012=CARTESIAN_POINT('Ctrl Pts',(-155.051444041475,41.6688140489355,
611.537703348572));
#272013=CARTESIAN_POINT('Ctrl Pts',(-150.837754439537,53.5400027769198,
609.537703348572));
#272014=CARTESIAN_POINT('Ctrl Pts',(-146.624064837599,65.411191504904,607.537703348572));
#272015=CARTESIAN_POINT('Ctrl Pts',(-140.605189688823,76.4770599218136,
605.537703348572));
#272016=CARTESIAN_POINT('Ctrl Pts',(-134.586314540048,87.5429283387233,
603.537703348572));
#272017=CARTESIAN_POINT('Ctrl Pts',(-126.9104585261,97.5309980386223,601.537703348572));
#272018=CARTESIAN_POINT('Ctrl Pts',(-119.234602512152,107.519067738521,
599.537703348572));
#272019=CARTESIAN_POINT('Ctrl Pts',(-110.0907706828,116.183399296895,597.537703348572));
#272020=CARTESIAN_POINT('Ctrl Pts',(-100.946938853448,124.847730855269,
595.537703348572));
#272021=CARTESIAN_POINT('Ctrl Pts',(-90.5602826949692,131.974979673883,
593.537703348572));
#272022=CARTESIAN_POINT('Ctrl Pts',(-80.1736265364901,139.102228492497,
591.537703348572));
#272023=CARTESIAN_POINT('Ctrl Pts',(-68.7998999948414,144.516898051454,
589.537703348572));
#272024=CARTESIAN_POINT('Ctrl Pts',(-57.4261734531926,149.931567610412,
587.537703348572));
#272025=CARTESIAN_POINT('Ctrl Pts',(-45.3454354230634,153.500330774912,
585.537703348572));
#272026=CARTESIAN_POINT('Ctrl Pts',(-33.2646973929343,157.069093939413,
583.537703348572));
#272027=CARTESIAN_POINT('Ctrl Pts',(-20.7744157382976,158.704075916301,
581.537703348572));
#272028=CARTESIAN_POINT('Ctrl Pts',(-8.284134083661,160.339057893189,579.537703348572));
#272029=CARTESIAN_POINT('Ctrl Pts',(4.30813900827803,160.,577.537703348572));
#272030=CARTESIAN_POINT('Ctrl Pts',(16.9004121002171,159.660942106811,575.537703348572));
#272031=CARTESIAN_POINT('Ctrl Pts',(29.2846130745762,157.356193074143,573.537703348572));
#272032=CARTESIAN_POINT('Ctrl Pts',(41.6688140489354,155.051444041476,571.537703348572));
#272033=CARTESIAN_POINT('Ctrl Pts',(53.5400027769198,150.837754439537,569.537703348572));
#272034=CARTESIAN_POINT('Ctrl Pts',(65.4111915049041,146.624064837599,567.537703348572));
#272035=CARTESIAN_POINT('Ctrl Pts',(76.4770599218136,140.605189688823,565.537703348572));
#272036=CARTESIAN_POINT('Ctrl Pts',(87.5429283387232,134.586314540048,563.537703348572));
#272037=CARTESIAN_POINT('Ctrl Pts',(97.5309980386223,126.9104585261,561.537703348572));
#272038=CARTESIAN_POINT('Ctrl Pts',(107.519067738521,119.234602512152,559.537703348572));
#272039=CARTESIAN_POINT('Ctrl Pts',(116.183399296895,110.0907706828,557.537703348572));
#272040=CARTESIAN_POINT('Ctrl Pts',(124.847730855269,100.946938853448,555.537703348572));
#272041=CARTESIAN_POINT('Ctrl Pts',(131.974979673883,90.5602826949692,553.537703348572));
#272042=CARTESIAN_POINT('Ctrl Pts',(139.102228492497,80.1736265364902,551.537703348572));
#272043=CARTESIAN_POINT('Ctrl Pts',(144.516898051454,68.7998999948414,549.537703348572));
#272044=CARTESIAN_POINT('Ctrl Pts',(149.931567610412,57.4261734531926,547.537703348572));
#272045=CARTESIAN_POINT('Ctrl Pts',(153.500330774912,45.3454354230634,545.537703348572));
#272046=CARTESIAN_POINT('Ctrl Pts',(157.069093939413,33.2646973929343,543.537703348572));
#272047=CARTESIAN_POINT('Ctrl Pts',(158.704075916301,20.7744157382976,541.537703348572));
#272048=CARTESIAN_POINT('Ctrl Pts',(160.339057893189,8.28413408366101,539.537703348572));
#272049=CARTESIAN_POINT('Ctrl Pts',(160.,-4.30813900827805,537.537703348572));
#272050=CARTESIAN_POINT('Ctrl Pts',(130.,4.30813900827812,532.462296651428));
#272051=CARTESIAN_POINT('Ctrl Pts',(130.339057893189,-5.92308287892228,
530.462296651428));
#272052=CARTESIAN_POINT('Ctrl Pts',(129.073425698447,-16.0813817870906,
528.462296651428));
#272053=CARTESIAN_POINT('Ctrl Pts',(127.807793503704,-26.2396806952589,
526.462296651428));
#272054=CARTESIAN_POINT('Ctrl Pts',(124.968635286058,-36.0749255918149,
524.462296651428));
#272055=CARTESIAN_POINT('Ctrl Pts',(122.129477068411,-45.9101704883709,
522.462296651428));
#272056=CARTESIAN_POINT('Ctrl Pts',(117.786702325803,-55.1801850026549,
520.462296651428));
#272057=CARTESIAN_POINT('Ctrl Pts',(113.443927583196,-64.4501995169389,
518.462296651428));
#272058=CARTESIAN_POINT('Ctrl Pts',(107.704469842635,-72.9267251261949,
516.462296651428));
#272059=CARTESIAN_POINT('Ctrl Pts',(101.965012102074,-81.4032507354509,
514.462296651428));
#272060=CARTESIAN_POINT('Ctrl Pts',(94.9701958612989,-88.8775672472035,
512.462296651428));
#272061=CARTESIAN_POINT('Ctrl Pts',(87.9753796205242,-96.351883758956,510.462296651428));
#272062=CARTESIAN_POINT('Ctrl Pts',(79.8974404698481,-102.639948694851,
508.462296651428));
#272063=CARTESIAN_POINT('Ctrl Pts',(71.8195013191721,-108.928013630747,
506.462296651428));
#272064=CARTESIAN_POINT('Ctrl Pts',(62.8573449296273,-113.874993963172,
504.462296651428));
#272065=CARTESIAN_POINT('Ctrl Pts',(53.8951885400825,-118.821974295598,
502.462296651428));
#272066=CARTESIAN_POINT('Ctrl Pts',(44.2694929456714,-122.306058950682,
500.462296651428));
#272067=CARTESIAN_POINT('Ctrl Pts',(34.6437973512603,-125.790143605767,
498.462296651428));
#272068=CARTESIAN_POINT('Ctrl Pts',(24.5915791233694,-127.725542856289,
496.462296651428));
#272069=CARTESIAN_POINT('Ctrl Pts',(14.5393608954785,-129.660942106811,
494.462296651428));
#272070=CARTESIAN_POINT('Ctrl Pts',(4.30813900827813,-130.,492.462296651428));
#272071=CARTESIAN_POINT('Ctrl Pts',(-5.92308287892227,-130.339057893189,
490.462296651428));
#272072=CARTESIAN_POINT('Ctrl Pts',(-16.0813817870906,-129.073425698447,
488.462296651428));
#272073=CARTESIAN_POINT('Ctrl Pts',(-26.2396806952589,-127.807793503705,
486.462296651428));
#272074=CARTESIAN_POINT('Ctrl Pts',(-36.0749255918149,-124.968635286058,
484.462296651428));
#272075=CARTESIAN_POINT('Ctrl Pts',(-45.9101704883709,-122.129477068411,
482.462296651428));
#272076=CARTESIAN_POINT('Ctrl Pts',(-55.1801850026549,-117.786702325803,
480.462296651428));
#272077=CARTESIAN_POINT('Ctrl Pts',(-64.4501995169389,-113.443927583196,
478.462296651428));
#272078=CARTESIAN_POINT('Ctrl Pts',(-72.9267251261949,-107.704469842635,
476.462296651428));
#272079=CARTESIAN_POINT('Ctrl Pts',(-81.4032507354509,-101.965012102074,
474.462296651428));
#272080=CARTESIAN_POINT('Ctrl Pts',(-88.8775672472034,-94.9701958612989,
472.462296651428));
#272081=CARTESIAN_POINT('Ctrl Pts',(-96.351883758956,-87.9753796205242,
470.462296651428));
#272082=CARTESIAN_POINT('Ctrl Pts',(-102.639948694851,-79.8974404698482,
468.462296651428));
#272083=CARTESIAN_POINT('Ctrl Pts',(-108.928013630747,-71.8195013191721,
466.462296651428));
#272084=CARTESIAN_POINT('Ctrl Pts',(-113.874993963172,-62.8573449296273,
464.462296651428));
#272085=CARTESIAN_POINT('Ctrl Pts',(-118.821974295598,-53.8951885400825,
462.462296651428));
#272086=CARTESIAN_POINT('Ctrl Pts',(-122.306058950682,-44.2694929456714,
460.462296651428));
#272087=CARTESIAN_POINT('Ctrl Pts',(-125.790143605767,-34.6437973512603,
458.462296651428));
#272088=CARTESIAN_POINT('Ctrl Pts',(-127.725542856289,-24.5915791233694,
456.462296651428));
#272089=CARTESIAN_POINT('Ctrl Pts',(-129.660942106811,-14.5393608954785,
454.462296651429));
#272090=CARTESIAN_POINT('Ctrl Pts',(-130.,-4.30813900827813,452.462296651428));
#272091=CARTESIAN_POINT('Ctrl Pts',(-130.339057893189,5.92308287892227,
450.462296651428));
#272092=CARTESIAN_POINT('Ctrl Pts',(-129.073425698447,16.0813817870906,
448.462296651428));
#272093=CARTESIAN_POINT('Ctrl Pts',(-127.807793503705,26.2396806952589,
446.462296651428));
#272094=CARTESIAN_POINT('Ctrl Pts',(-124.968635286058,36.0749255918149,
444.462296651428));
#272095=CARTESIAN_POINT('Ctrl Pts',(-122.129477068411,45.9101704883709,
442.462296651428));
#272096=CARTESIAN_POINT('Ctrl Pts',(-117.786702325803,55.1801850026549,
440.462296651428));
#272097=CARTESIAN_POINT('Ctrl Pts',(-113.443927583196,64.4501995169388,
438.462296651428));
#272098=CARTESIAN_POINT('Ctrl Pts',(-107.704469842635,72.9267251261949,
436.462296651428));
#272099=CARTESIAN_POINT('Ctrl Pts',(-101.965012102074,81.4032507354509,
434.462296651428));
#272100=CARTESIAN_POINT('Ctrl Pts',(-94.9701958612989,88.8775672472034,
432.462296651428));
#272101=CARTESIAN_POINT('Ctrl Pts',(-87.9753796205243,96.3518837589559,
430.462296651428));
#272102=CARTESIAN_POINT('Ctrl Pts',(-79.8974404698482,102.639948694851,
428.462296651428));
#272103=CARTESIAN_POINT('Ctrl Pts',(-71.819501319172,108.928013630747,426.462296651428));
#272104=CARTESIAN_POINT('Ctrl Pts',(-62.8573449296273,113.874993963172,
424.462296651428));
#272105=CARTESIAN_POINT('Ctrl Pts',(-53.8951885400826,118.821974295598,
422.462296651428));
#272106=CARTESIAN_POINT('Ctrl Pts',(-44.2694929456714,122.306058950682,
420.462296651428));
#272107=CARTESIAN_POINT('Ctrl Pts',(-34.6437973512603,125.790143605767,
418.462296651428));
#272108=CARTESIAN_POINT('Ctrl Pts',(-24.5915791233694,127.725542856289,
416.462296651428));
#272109=CARTESIAN_POINT('Ctrl Pts',(-14.5393608954786,129.660942106811,
414.462296651428));
#272110=CARTESIAN_POINT('Ctrl Pts',(-4.30813900827814,130.,412.462296651428));
#272111=CARTESIAN_POINT('Ctrl Pts',(5.92308287892232,130.339057893189,410.462296651428));
#272112=CARTESIAN_POINT('Ctrl Pts',(16.0813817870906,129.073425698447,408.462296651428));
#272113=CARTESIAN_POINT('Ctrl Pts',(26.2396806952589,127.807793503705,406.462296651428));
#272114=CARTESIAN_POINT('Ctrl Pts',(36.0749255918149,124.968635286058,404.462296651428));
#272115=CARTESIAN_POINT('Ctrl Pts',(45.9101704883709,122.129477068411,402.462296651428));
#272116=CARTESIAN_POINT('Ctrl Pts',(55.1801850026549,117.786702325803,400.462296651428));
#272117=CARTESIAN_POINT('Ctrl Pts',(64.4501995169388,113.443927583196,398.462296651428));
#272118=CARTESIAN_POINT('Ctrl Pts',(72.9267251261949,107.704469842635,396.462296651428));
#272119=CARTESIAN_POINT('Ctrl Pts',(81.4032507354509,101.965012102074,394.462296651428));
#272120=CARTESIAN_POINT('Ctrl Pts',(88.8775672472034,94.9701958612989,392.462296651428));
#272121=CARTESIAN_POINT('Ctrl Pts',(96.3518837589559,87.9753796205243,390.462296651428));
#272122=CARTESIAN_POINT('Ctrl Pts',(102.639948694851,79.8974404698482,388.462296651428));
#272123=CARTESIAN_POINT('Ctrl Pts',(108.928013630747,71.819501319172,386.462296651428));
#272124=CARTESIAN_POINT('Ctrl Pts',(113.874993963172,62.8573449296273,384.462296651428));
#272125=CARTESIAN_POINT('Ctrl Pts',(118.821974295598,53.8951885400826,382.462296651428));
#272126=CARTESIAN_POINT('Ctrl Pts',(122.306058950682,44.2694929456714,380.462296651428));
#272127=CARTESIAN_POINT('Ctrl Pts',(125.790143605767,34.6437973512603,378.462296651428));
#272128=CARTESIAN_POINT('Ctrl Pts',(127.725542856289,24.5915791233694,376.462296651428));
#272129=CARTESIAN_POINT('Ctrl Pts',(129.660942106811,14.5393608954786,374.462296651428));
#272130=CARTESIAN_POINT('Ctrl Pts',(130.,4.30813900827812,372.462296651428));
#272131=CARTESIAN_POINT('Ctrl Pts',(160.,4.30813900827813,532.462296651428));
#272132=CARTESIAN_POINT('Ctrl Pts',(160.339057893189,-8.28413408366083,
530.462296651428));
#272133=CARTESIAN_POINT('Ctrl Pts',(158.704075916301,-20.7744157382975,
528.462296651428));
#272134=CARTESIAN_POINT('Ctrl Pts',(157.069093939413,-33.2646973929343,
526.462296651428));
#272135=CARTESIAN_POINT('Ctrl Pts',(153.500330774912,-45.3454354230633,
524.462296651428));
#272136=CARTESIAN_POINT('Ctrl Pts',(149.931567610412,-57.4261734531924,
522.462296651428));
#272137=CARTESIAN_POINT('Ctrl Pts',(144.516898051455,-68.7998999948413,
520.462296651428));
#272138=CARTESIAN_POINT('Ctrl Pts',(139.102228492497,-80.1736265364901,
518.462296651428));
#272139=CARTESIAN_POINT('Ctrl Pts',(131.974979673883,-90.5602826949691,
516.462296651428));
#272140=CARTESIAN_POINT('Ctrl Pts',(124.847730855269,-100.946938853448,
514.462296651428));
#272141=CARTESIAN_POINT('Ctrl Pts',(116.183399296895,-110.0907706828,512.462296651428));
#272142=CARTESIAN_POINT('Ctrl Pts',(107.519067738521,-119.234602512152,
510.462296651428));
#272143=CARTESIAN_POINT('Ctrl Pts',(97.5309980386224,-126.9104585261,508.462296651428));
#272144=CARTESIAN_POINT('Ctrl Pts',(87.5429283387234,-134.586314540048,
506.462296651428));
#272145=CARTESIAN_POINT('Ctrl Pts',(76.4770599218137,-140.605189688823,
504.462296651428));
#272146=CARTESIAN_POINT('Ctrl Pts',(65.4111915049041,-146.624064837599,
502.462296651428));
#272147=CARTESIAN_POINT('Ctrl Pts',(53.5400027769198,-150.837754439537,
500.462296651428));
#272148=CARTESIAN_POINT('Ctrl Pts',(41.6688140489356,-155.051444041475,
498.462296651428));
#272149=CARTESIAN_POINT('Ctrl Pts',(29.2846130745764,-157.356193074143,
496.462296651428));
#272150=CARTESIAN_POINT('Ctrl Pts',(16.9004121002171,-159.660942106811,
494.462296651428));
#272151=CARTESIAN_POINT('Ctrl Pts',(4.30813900827814,-160.,492.462296651428));
#272152=CARTESIAN_POINT('Ctrl Pts',(-8.28413408366082,-160.339057893189,
490.462296651428));
#272153=CARTESIAN_POINT('Ctrl Pts',(-20.7744157382975,-158.704075916301,
488.462296651428));
#272154=CARTESIAN_POINT('Ctrl Pts',(-33.2646973929342,-157.069093939413,
486.462296651428));
#272155=CARTESIAN_POINT('Ctrl Pts',(-45.3454354230633,-153.500330774912,
484.462296651428));
#272156=CARTESIAN_POINT('Ctrl Pts',(-57.4261734531924,-149.931567610412,
482.462296651428));
#272157=CARTESIAN_POINT('Ctrl Pts',(-68.7998999948413,-144.516898051455,
480.462296651428));
#272158=CARTESIAN_POINT('Ctrl Pts',(-80.1736265364901,-139.102228492497,
478.462296651428));
#272159=CARTESIAN_POINT('Ctrl Pts',(-90.5602826949691,-131.974979673883,
476.462296651428));
#272160=CARTESIAN_POINT('Ctrl Pts',(-100.946938853448,-124.847730855269,
474.462296651428));
#272161=CARTESIAN_POINT('Ctrl Pts',(-110.0907706828,-116.183399296895,472.462296651428));
#272162=CARTESIAN_POINT('Ctrl Pts',(-119.234602512152,-107.519067738521,
470.462296651428));
#272163=CARTESIAN_POINT('Ctrl Pts',(-126.9104585261,-97.5309980386224,468.462296651428));
#272164=CARTESIAN_POINT('Ctrl Pts',(-134.586314540048,-87.5429283387234,
466.462296651428));
#272165=CARTESIAN_POINT('Ctrl Pts',(-140.605189688823,-76.4770599218137,
464.462296651428));
#272166=CARTESIAN_POINT('Ctrl Pts',(-146.624064837599,-65.4111915049041,
462.462296651428));
#272167=CARTESIAN_POINT('Ctrl Pts',(-150.837754439537,-53.5400027769199,
460.462296651428));
#272168=CARTESIAN_POINT('Ctrl Pts',(-155.051444041475,-41.6688140489356,
458.462296651428));
#272169=CARTESIAN_POINT('Ctrl Pts',(-157.356193074143,-29.2846130745764,
456.462296651428));
#272170=CARTESIAN_POINT('Ctrl Pts',(-159.660942106811,-16.9004121002171,
454.462296651429));
#272171=CARTESIAN_POINT('Ctrl Pts',(-160.,-4.30813900827815,452.462296651428));
#272172=CARTESIAN_POINT('Ctrl Pts',(-160.339057893189,8.28413408366081,
450.462296651428));
#272173=CARTESIAN_POINT('Ctrl Pts',(-158.704075916301,20.7744157382975,
448.462296651428));
#272174=CARTESIAN_POINT('Ctrl Pts',(-157.069093939413,33.2646973929342,
446.462296651428));
#272175=CARTESIAN_POINT('Ctrl Pts',(-153.500330774912,45.3454354230633,
444.462296651428));
#272176=CARTESIAN_POINT('Ctrl Pts',(-149.931567610412,57.4261734531924,
442.462296651428));
#272177=CARTESIAN_POINT('Ctrl Pts',(-144.516898051455,68.7998999948413,
440.462296651428));
#272178=CARTESIAN_POINT('Ctrl Pts',(-139.102228492497,80.1736265364901,
438.462296651428));
#272179=CARTESIAN_POINT('Ctrl Pts',(-131.974979673883,90.5602826949691,
436.462296651428));
#272180=CARTESIAN_POINT('Ctrl Pts',(-124.847730855269,100.946938853448,
434.462296651428));
#272181=CARTESIAN_POINT('Ctrl Pts',(-116.183399296895,110.0907706828,432.462296651428));
#272182=CARTESIAN_POINT('Ctrl Pts',(-107.519067738521,119.234602512152,
430.462296651428));
#272183=CARTESIAN_POINT('Ctrl Pts',(-97.5309980386224,126.9104585261,428.462296651428));
#272184=CARTESIAN_POINT('Ctrl Pts',(-87.5429283387233,134.586314540048,
426.462296651428));
#272185=CARTESIAN_POINT('Ctrl Pts',(-76.4770599218137,140.605189688823,
424.462296651428));
#272186=CARTESIAN_POINT('Ctrl Pts',(-65.4111915049042,146.624064837599,
422.462296651428));
#272187=CARTESIAN_POINT('Ctrl Pts',(-53.5400027769199,150.837754439537,
420.462296651428));
#272188=CARTESIAN_POINT('Ctrl Pts',(-41.6688140489356,155.051444041475,
418.462296651428));
#272189=CARTESIAN_POINT('Ctrl Pts',(-29.2846130745764,157.356193074143,
416.462296651428));
#272190=CARTESIAN_POINT('Ctrl Pts',(-16.9004121002172,159.660942106811,
414.462296651428));
#272191=CARTESIAN_POINT('Ctrl Pts',(-4.30813900827816,160.,412.462296651428));
#272192=CARTESIAN_POINT('Ctrl Pts',(8.28413408366087,160.339057893189,410.462296651428));
#272193=CARTESIAN_POINT('Ctrl Pts',(20.7744157382975,158.704075916301,408.462296651428));
#272194=CARTESIAN_POINT('Ctrl Pts',(33.2646973929342,157.069093939413,406.462296651428));
#272195=CARTESIAN_POINT('Ctrl Pts',(45.3454354230633,153.500330774912,404.462296651428));
#272196=CARTESIAN_POINT('Ctrl Pts',(57.4261734531925,149.931567610412,402.462296651428));
#272197=CARTESIAN_POINT('Ctrl Pts',(68.7998999948413,144.516898051455,400.462296651428));
#272198=CARTESIAN_POINT('Ctrl Pts',(80.1736265364901,139.102228492498,398.462296651428));
#272199=CARTESIAN_POINT('Ctrl Pts',(90.560282694969,131.974979673883,396.462296651428));
#272200=CARTESIAN_POINT('Ctrl Pts',(100.946938853448,124.847730855269,394.462296651428));
#272201=CARTESIAN_POINT('Ctrl Pts',(110.0907706828,116.183399296895,392.462296651428));
#272202=CARTESIAN_POINT('Ctrl Pts',(119.234602512152,107.519067738521,390.462296651428));
#272203=CARTESIAN_POINT('Ctrl Pts',(126.9104585261,97.5309980386224,388.462296651428));
#272204=CARTESIAN_POINT('Ctrl Pts',(134.586314540048,87.5429283387233,386.462296651428));
#272205=CARTESIAN_POINT('Ctrl Pts',(140.605189688823,76.4770599218137,384.462296651428));
#272206=CARTESIAN_POINT('Ctrl Pts',(146.624064837599,65.4111915049042,382.462296651428));
#272207=CARTESIAN_POINT('Ctrl Pts',(150.837754439537,53.5400027769199,380.462296651428));
#272208=CARTESIAN_POINT('Ctrl Pts',(155.051444041475,41.6688140489356,378.462296651428));
#272209=CARTESIAN_POINT('Ctrl Pts',(157.356193074143,29.2846130745764,376.462296651428));
#272210=CARTESIAN_POINT('Ctrl Pts',(159.660942106811,16.9004121002172,374.462296651428));
#272211=CARTESIAN_POINT('Ctrl Pts',(160.,4.30813900827813,372.462296651428));
#272212=CARTESIAN_POINT('Origin',(-4.03737035478777,0.209103844014949,530.462377392398));
#272213=CARTESIAN_POINT('Ctrl Pts',(160.,4.30813900827813,532.462296651428));
#272214=CARTESIAN_POINT('Ctrl Pts',(160.339057893189,-8.28413408366083,
530.462296651428));
#272215=CARTESIAN_POINT('Ctrl Pts',(158.704075916301,-20.7744157382975,
528.462296651428));
#272216=CARTESIAN_POINT('Ctrl Pts',(157.069093939413,-33.2646973929343,
526.462296651428));
#272217=CARTESIAN_POINT('Ctrl Pts',(153.500330774912,-45.3454354230633,
524.462296651428));
#272218=CARTESIAN_POINT('Ctrl Pts',(149.931567610412,-57.4261734531924,
522.462296651428));
#272219=CARTESIAN_POINT('Ctrl Pts',(144.516898051455,-68.7998999948413,
520.462296651428));
#272220=CARTESIAN_POINT('Ctrl Pts',(139.102228492497,-80.1736265364901,
518.462296651428));
#272221=CARTESIAN_POINT('Ctrl Pts',(131.974979673883,-90.5602826949691,
516.462296651428));
#272222=CARTESIAN_POINT('Ctrl Pts',(124.847730855269,-100.946938853448,
514.462296651428));
#272223=CARTESIAN_POINT('Ctrl Pts',(116.183399296895,-110.0907706828,512.462296651428));
#272224=CARTESIAN_POINT('Ctrl Pts',(107.519067738521,-119.234602512152,
510.462296651428));
#272225=CARTESIAN_POINT('Ctrl Pts',(97.5309980386224,-126.9104585261,508.462296651428));
#272226=CARTESIAN_POINT('Ctrl Pts',(87.5429283387234,-134.586314540048,
506.462296651428));
#272227=CARTESIAN_POINT('Ctrl Pts',(76.4770599218137,-140.605189688823,
504.462296651428));
#272228=CARTESIAN_POINT('Ctrl Pts',(65.4111915049041,-146.624064837599,
502.462296651428));
#272229=CARTESIAN_POINT('Ctrl Pts',(53.5400027769198,-150.837754439537,
500.462296651428));
#272230=CARTESIAN_POINT('Ctrl Pts',(41.6688140489356,-155.051444041475,
498.462296651428));
#272231=CARTESIAN_POINT('Ctrl Pts',(29.2846130745764,-157.356193074143,
496.462296651428));
#272232=CARTESIAN_POINT('Ctrl Pts',(16.9004121002171,-159.660942106811,
494.462296651428));
#272233=CARTESIAN_POINT('Ctrl Pts',(4.30813900827814,-160.,492.462296651428));
#272234=CARTESIAN_POINT('Ctrl Pts',(-8.28413408366082,-160.339057893189,
490.462296651428));
#272235=CARTESIAN_POINT('Ctrl Pts',(-20.7744157382975,-158.704075916301,
488.462296651428));
#272236=CARTESIAN_POINT('Ctrl Pts',(-33.2646973929342,-157.069093939413,
486.462296651428));
#272237=CARTESIAN_POINT('Ctrl Pts',(-45.3454354230633,-153.500330774912,
484.462296651428));
#272238=CARTESIAN_POINT('Ctrl Pts',(-57.4261734531924,-149.931567610412,
482.462296651428));
#272239=CARTESIAN_POINT('Ctrl Pts',(-68.7998999948413,-144.516898051455,
480.462296651428));
#272240=CARTESIAN_POINT('Ctrl Pts',(-80.1736265364901,-139.102228492497,
478.462296651428));
#272241=CARTESIAN_POINT('Ctrl Pts',(-90.5602826949691,-131.974979673883,
476.462296651428));
#272242=CARTESIAN_POINT('Ctrl Pts',(-100.946938853448,-124.847730855269,
474.462296651428));
#272243=CARTESIAN_POINT('Ctrl Pts',(-110.0907706828,-116.183399296895,472.462296651428));
#272244=CARTESIAN_POINT('Ctrl Pts',(-119.234602512152,-107.519067738521,
470.462296651428));
#272245=CARTESIAN_POINT('Ctrl Pts',(-126.9104585261,-97.5309980386224,468.462296651428));
#272246=CARTESIAN_POINT('Ctrl Pts',(-134.586314540048,-87.5429283387234,
466.462296651428));
#272247=CARTESIAN_POINT('Ctrl Pts',(-140.605189688823,-76.4770599218137,
464.462296651428));
#272248=CARTESIAN_POINT('Ctrl Pts',(-146.624064837599,-65.4111915049041,
462.462296651428));
#272249=CARTESIAN_POINT('Ctrl Pts',(-150.837754439537,-53.5400027769199,
460.462296651428));
#272250=CARTESIAN_POINT('Ctrl Pts',(-155.051444041475,-41.6688140489356,
458.462296651428));
#272251=CARTESIAN_POINT('Ctrl Pts',(-157.356193074143,-29.2846130745764,
456.462296651428));
#272252=CARTESIAN_POINT('Ctrl Pts',(-159.660942106811,-16.9004121002171,
454.462296651429));
#272253=CARTESIAN_POINT('Ctrl Pts',(-160.,-4.30813900827815,452.462296651428));
#272254=CARTESIAN_POINT('Ctrl Pts',(-160.339057893189,8.28413408366081,
450.462296651428));
#272255=CARTESIAN_POINT('Ctrl Pts',(-158.704075916301,20.7744157382975,
448.462296651428));
#272256=CARTESIAN_POINT('Ctrl Pts',(-157.069093939413,33.2646973929342,
446.462296651428));
#272257=CARTESIAN_POINT('Ctrl Pts',(-153.500330774912,45.3454354230633,
444.462296651428));
#272258=CARTESIAN_POINT('Ctrl Pts',(-149.931567610412,57.4261734531924,
442.462296651428));
#272259=CARTESIAN_POINT('Ctrl Pts',(-144.516898051455,68.7998999948413,
440.462296651428));
#272260=CARTESIAN_POINT('Ctrl Pts',(-139.102228492497,80.1736265364901,
438.462296651428));
#272261=CARTESIAN_POINT('Ctrl Pts',(-131.974979673883,90.5602826949691,
436.462296651428));
#272262=CARTESIAN_POINT('Ctrl Pts',(-124.847730855269,100.946938853448,
434.462296651428));
#272263=CARTESIAN_POINT('Ctrl Pts',(-116.183399296895,110.0907706828,432.462296651428));
#272264=CARTESIAN_POINT('Ctrl Pts',(-107.519067738521,119.234602512152,
430.462296651428));
#272265=CARTESIAN_POINT('Ctrl Pts',(-97.5309980386224,126.9104585261,428.462296651428));
#272266=CARTESIAN_POINT('Ctrl Pts',(-87.5429283387233,134.586314540048,
426.462296651428));
#272267=CARTESIAN_POINT('Ctrl Pts',(-76.4770599218137,140.605189688823,
424.462296651428));
#272268=CARTESIAN_POINT('Ctrl Pts',(-65.4111915049042,146.624064837599,
422.462296651428));
#272269=CARTESIAN_POINT('Ctrl Pts',(-53.5400027769199,150.837754439537,
420.462296651428));
#272270=CARTESIAN_POINT('Ctrl Pts',(-41.6688140489356,155.051444041475,
418.462296651428));
#272271=CARTESIAN_POINT('Ctrl Pts',(-29.2846130745764,157.356193074143,
416.462296651428));
#272272=CARTESIAN_POINT('Ctrl Pts',(-16.9004121002172,159.660942106811,
414.462296651428));
#272273=CARTESIAN_POINT('Ctrl Pts',(-4.30813900827816,160.,412.462296651428));
#272274=CARTESIAN_POINT('Ctrl Pts',(8.28413408366087,160.339057893189,410.462296651428));
#272275=CARTESIAN_POINT('Ctrl Pts',(20.7744157382975,158.704075916301,408.462296651428));
#272276=CARTESIAN_POINT('Ctrl Pts',(33.2646973929342,157.069093939413,406.462296651428));
#272277=CARTESIAN_POINT('Ctrl Pts',(45.3454354230633,153.500330774912,404.462296651428));
#272278=CARTESIAN_POINT('Ctrl Pts',(57.4261734531925,149.931567610412,402.462296651428));
#272279=CARTESIAN_POINT('Ctrl Pts',(68.7998999948413,144.516898051455,400.462296651428));
#272280=CARTESIAN_POINT('Ctrl Pts',(80.1736265364901,139.102228492498,398.462296651428));
#272281=CARTESIAN_POINT('Ctrl Pts',(90.560282694969,131.974979673883,396.462296651428));
#272282=CARTESIAN_POINT('Ctrl Pts',(100.946938853448,124.847730855269,394.462296651428));
#272283=CARTESIAN_POINT('Ctrl Pts',(110.0907706828,116.183399296895,392.462296651428));
#272284=CARTESIAN_POINT('Ctrl Pts',(119.234602512152,107.519067738521,390.462296651428));
#272285=CARTESIAN_POINT('Ctrl Pts',(126.9104585261,97.5309980386224,388.462296651428));
#272286=CARTESIAN_POINT('Ctrl Pts',(134.586314540048,87.5429283387233,386.462296651428));
#272287=CARTESIAN_POINT('Ctrl Pts',(140.605189688823,76.4770599218137,384.462296651428));
#272288=CARTESIAN_POINT('Ctrl Pts',(146.624064837599,65.4111915049042,382.462296651428));
#272289=CARTESIAN_POINT('Ctrl Pts',(150.837754439537,53.5400027769199,380.462296651428));
#272290=CARTESIAN_POINT('Ctrl Pts',(155.051444041475,41.6688140489356,378.462296651428));
#272291=CARTESIAN_POINT('Ctrl Pts',(157.356193074143,29.2846130745764,376.462296651428));
#272292=CARTESIAN_POINT('Ctrl Pts',(159.660942106811,16.9004121002172,374.462296651428));
#272293=CARTESIAN_POINT('Ctrl Pts',(160.,4.30813900827813,372.462296651428));
#272294=CARTESIAN_POINT('Ctrl Pts',(160.,-4.30813900827805,537.537703348572));
#272295=CARTESIAN_POINT('Ctrl Pts',(159.660942106811,-16.900412100217,535.537703348572));
#272296=CARTESIAN_POINT('Ctrl Pts',(157.356193074143,-29.2846130745763,
533.537703348572));
#272297=CARTESIAN_POINT('Ctrl Pts',(155.051444041475,-41.6688140489355,
531.537703348572));
#272298=CARTESIAN_POINT('Ctrl Pts',(150.837754439537,-53.5400027769198,
529.537703348572));
#272299=CARTESIAN_POINT('Ctrl Pts',(146.624064837599,-65.411191504904,527.537703348572));
#272300=CARTESIAN_POINT('Ctrl Pts',(140.605189688823,-76.4770599218136,
525.537703348572));
#272301=CARTESIAN_POINT('Ctrl Pts',(134.586314540048,-87.5429283387233,
523.537703348572));
#272302=CARTESIAN_POINT('Ctrl Pts',(126.9104585261,-97.5309980386223,521.537703348572));
#272303=CARTESIAN_POINT('Ctrl Pts',(119.234602512152,-107.519067738521,
519.537703348572));
#272304=CARTESIAN_POINT('Ctrl Pts',(110.0907706828,-116.183399296895,517.537703348572));
#272305=CARTESIAN_POINT('Ctrl Pts',(100.946938853448,-124.847730855269,
515.537703348572));
#272306=CARTESIAN_POINT('Ctrl Pts',(90.5602826949691,-131.974979673883,
513.537703348572));
#272307=CARTESIAN_POINT('Ctrl Pts',(80.1736265364902,-139.102228492497,
511.537703348572));
#272308=CARTESIAN_POINT('Ctrl Pts',(68.7998999948414,-144.516898051454,
509.537703348572));
#272309=CARTESIAN_POINT('Ctrl Pts',(57.4261734531925,-149.931567610412,
507.537703348572));
#272310=CARTESIAN_POINT('Ctrl Pts',(45.3454354230634,-153.500330774912,
505.537703348572));
#272311=CARTESIAN_POINT('Ctrl Pts',(33.2646973929343,-157.069093939413,
503.537703348572));
#272312=CARTESIAN_POINT('Ctrl Pts',(20.7744157382976,-158.704075916301,
501.537703348572));
#272313=CARTESIAN_POINT('Ctrl Pts',(8.28413408366091,-160.339057893189,
499.537703348572));
#272314=CARTESIAN_POINT('Ctrl Pts',(-4.30813900827804,-160.,497.537703348572));
#272315=CARTESIAN_POINT('Ctrl Pts',(-16.900412100217,-159.660942106811,
495.537703348572));
#272316=CARTESIAN_POINT('Ctrl Pts',(-29.2846130745763,-157.356193074143,
493.537703348572));
#272317=CARTESIAN_POINT('Ctrl Pts',(-41.6688140489355,-155.051444041475,
491.537703348572));
#272318=CARTESIAN_POINT('Ctrl Pts',(-53.5400027769198,-150.837754439537,
489.537703348572));
#272319=CARTESIAN_POINT('Ctrl Pts',(-65.411191504904,-146.624064837599,
487.537703348572));
#272320=CARTESIAN_POINT('Ctrl Pts',(-76.4770599218136,-140.605189688823,
485.537703348572));
#272321=CARTESIAN_POINT('Ctrl Pts',(-87.5429283387233,-134.586314540048,
483.537703348572));
#272322=CARTESIAN_POINT('Ctrl Pts',(-97.5309980386223,-126.9104585261,481.537703348572));
#272323=CARTESIAN_POINT('Ctrl Pts',(-107.519067738521,-119.234602512152,
479.537703348572));
#272324=CARTESIAN_POINT('Ctrl Pts',(-116.183399296895,-110.0907706828,477.537703348572));
#272325=CARTESIAN_POINT('Ctrl Pts',(-124.847730855269,-100.946938853448,
475.537703348572));
#272326=CARTESIAN_POINT('Ctrl Pts',(-131.974979673883,-90.5602826949692,
473.537703348572));
#272327=CARTESIAN_POINT('Ctrl Pts',(-139.102228492497,-80.1736265364902,
471.537703348572));
#272328=CARTESIAN_POINT('Ctrl Pts',(-144.516898051454,-68.7998999948414,
469.537703348572));
#272329=CARTESIAN_POINT('Ctrl Pts',(-149.931567610412,-57.4261734531925,
467.537703348572));
#272330=CARTESIAN_POINT('Ctrl Pts',(-153.500330774912,-45.3454354230634,
465.537703348572));
#272331=CARTESIAN_POINT('Ctrl Pts',(-157.069093939413,-33.2646973929344,
463.537703348572));
#272332=CARTESIAN_POINT('Ctrl Pts',(-158.704075916301,-20.7744157382976,
461.537703348572));
#272333=CARTESIAN_POINT('Ctrl Pts',(-160.339057893189,-8.28413408366092,
459.537703348572));
#272334=CARTESIAN_POINT('Ctrl Pts',(-160.,4.30813900827803,457.537703348572));
#272335=CARTESIAN_POINT('Ctrl Pts',(-159.660942106811,16.900412100217,455.537703348572));
#272336=CARTESIAN_POINT('Ctrl Pts',(-157.356193074143,29.2846130745763,
453.537703348572));
#272337=CARTESIAN_POINT('Ctrl Pts',(-155.051444041475,41.6688140489355,
451.537703348572));
#272338=CARTESIAN_POINT('Ctrl Pts',(-150.837754439537,53.5400027769198,
449.537703348572));
#272339=CARTESIAN_POINT('Ctrl Pts',(-146.624064837599,65.411191504904,447.537703348572));
#272340=CARTESIAN_POINT('Ctrl Pts',(-140.605189688823,76.4770599218136,
445.537703348572));
#272341=CARTESIAN_POINT('Ctrl Pts',(-134.586314540048,87.5429283387233,
443.537703348572));
#272342=CARTESIAN_POINT('Ctrl Pts',(-126.9104585261,97.5309980386223,441.537703348572));
#272343=CARTESIAN_POINT('Ctrl Pts',(-119.234602512152,107.519067738521,
439.537703348572));
#272344=CARTESIAN_POINT('Ctrl Pts',(-110.0907706828,116.183399296895,437.537703348572));
#272345=CARTESIAN_POINT('Ctrl Pts',(-100.946938853448,124.847730855269,
435.537703348572));
#272346=CARTESIAN_POINT('Ctrl Pts',(-90.5602826949692,131.974979673883,
433.537703348572));
#272347=CARTESIAN_POINT('Ctrl Pts',(-80.1736265364901,139.102228492497,
431.537703348572));
#272348=CARTESIAN_POINT('Ctrl Pts',(-68.7998999948414,144.516898051454,
429.537703348572));
#272349=CARTESIAN_POINT('Ctrl Pts',(-57.4261734531926,149.931567610412,
427.537703348572));
#272350=CARTESIAN_POINT('Ctrl Pts',(-45.3454354230634,153.500330774912,
425.537703348572));
#272351=CARTESIAN_POINT('Ctrl Pts',(-33.2646973929343,157.069093939413,
423.537703348572));
#272352=CARTESIAN_POINT('Ctrl Pts',(-20.7744157382976,158.704075916301,
421.537703348572));
#272353=CARTESIAN_POINT('Ctrl Pts',(-8.284134083661,160.339057893189,419.537703348572));
#272354=CARTESIAN_POINT('Ctrl Pts',(4.30813900827803,160.,417.537703348572));
#272355=CARTESIAN_POINT('Ctrl Pts',(16.9004121002171,159.660942106811,415.537703348572));
#272356=CARTESIAN_POINT('Ctrl Pts',(29.2846130745762,157.356193074143,413.537703348572));
#272357=CARTESIAN_POINT('Ctrl Pts',(41.6688140489354,155.051444041476,411.537703348572));
#272358=CARTESIAN_POINT('Ctrl Pts',(53.5400027769198,150.837754439537,409.537703348572));
#272359=CARTESIAN_POINT('Ctrl Pts',(65.4111915049041,146.624064837599,407.537703348572));
#272360=CARTESIAN_POINT('Ctrl Pts',(76.4770599218136,140.605189688823,405.537703348572));
#272361=CARTESIAN_POINT('Ctrl Pts',(87.5429283387232,134.586314540048,403.537703348572));
#272362=CARTESIAN_POINT('Ctrl Pts',(97.5309980386223,126.9104585261,401.537703348572));
#272363=CARTESIAN_POINT('Ctrl Pts',(107.519067738521,119.234602512152,399.537703348572));
#272364=CARTESIAN_POINT('Ctrl Pts',(116.183399296895,110.0907706828,397.537703348572));
#272365=CARTESIAN_POINT('Ctrl Pts',(124.847730855269,100.946938853448,395.537703348572));
#272366=CARTESIAN_POINT('Ctrl Pts',(131.974979673883,90.5602826949692,393.537703348572));
#272367=CARTESIAN_POINT('Ctrl Pts',(139.102228492497,80.1736265364902,391.537703348572));
#272368=CARTESIAN_POINT('Ctrl Pts',(144.516898051454,68.7998999948414,389.537703348572));
#272369=CARTESIAN_POINT('Ctrl Pts',(149.931567610412,57.4261734531926,387.537703348572));
#272370=CARTESIAN_POINT('Ctrl Pts',(153.500330774912,45.3454354230634,385.537703348572));
#272371=CARTESIAN_POINT('Ctrl Pts',(157.069093939413,33.2646973929343,383.537703348572));
#272372=CARTESIAN_POINT('Ctrl Pts',(158.704075916301,20.7744157382976,381.537703348572));
#272373=CARTESIAN_POINT('Ctrl Pts',(160.339057893189,8.28413408366101,379.537703348572));
#272374=CARTESIAN_POINT('Ctrl Pts',(160.,-4.30813900827805,377.537703348572));
#272375=CARTESIAN_POINT('Origin',(160.,3.64291929955129E-14,375.));
#272376=CARTESIAN_POINT('',(160.,-4.30813900827807,377.537703348572));
#272377=CARTESIAN_POINT('',(160.,1.10715726269171E-13,375.));
#272378=CARTESIAN_POINT('',(160.,3.64291929955129E-14,375.));
#272379=CARTESIAN_POINT('',(160.,4.30813900827833,378.90811221526));
#272380=CARTESIAN_POINT('Ctrl Pts',(160.,-4.30813900827807,377.537703348572));
#272381=CARTESIAN_POINT('Ctrl Pts',(160.,-1.43594781992484,377.99388646458));
#272382=CARTESIAN_POINT('Ctrl Pts',(160.,1.43604209806729,378.451335906457));
#272383=CARTESIAN_POINT('Ctrl Pts',(160.,4.30813900827833,378.90811221526));
#272384=CARTESIAN_POINT('Ctrl Pts',(160.,4.30813900827833,378.90811221526));
#272385=CARTESIAN_POINT('Ctrl Pts',(160.,2.8921527671012,377.623305748502));
#272386=CARTESIAN_POINT('Ctrl Pts',(160.,1.4761797878303,376.338484547026));
#272387=CARTESIAN_POINT('Ctrl Pts',(160.,0.0597455111575994,375.05417203362));
#272388=CARTESIAN_POINT('Ctrl Pts',(160.,0.039830432387403,375.036114588039));
#272389=CARTESIAN_POINT('Ctrl Pts',(160.,0.0199151703859646,375.01805734454));
#272390=CARTESIAN_POINT('Ctrl Pts',(160.,1.64868119156836E-13,375.));
#272391=CARTESIAN_POINT('Ctrl Pts',(160.,4.30813900827813,532.462296651428));
#272392=CARTESIAN_POINT('Ctrl Pts',(160.339057893189,-8.28413408366083,
530.462296651428));
#272393=CARTESIAN_POINT('Ctrl Pts',(158.704075916301,-20.7744157382975,
528.462296651428));
#272394=CARTESIAN_POINT('Ctrl Pts',(157.069093939413,-33.2646973929343,
526.462296651428));
#272395=CARTESIAN_POINT('Ctrl Pts',(153.500330774912,-45.3454354230633,
524.462296651428));
#272396=CARTESIAN_POINT('Ctrl Pts',(149.931567610412,-57.4261734531924,
522.462296651428));
#272397=CARTESIAN_POINT('Ctrl Pts',(144.516898051455,-68.7998999948413,
520.462296651428));
#272398=CARTESIAN_POINT('Ctrl Pts',(139.102228492497,-80.1736265364901,
518.462296651428));
#272399=CARTESIAN_POINT('Ctrl Pts',(131.974979673883,-90.5602826949691,
516.462296651428));
#272400=CARTESIAN_POINT('Ctrl Pts',(124.847730855269,-100.946938853448,
514.462296651428));
#272401=CARTESIAN_POINT('Ctrl Pts',(116.183399296895,-110.0907706828,512.462296651428));
#272402=CARTESIAN_POINT('Ctrl Pts',(107.519067738521,-119.234602512152,
510.462296651428));
#272403=CARTESIAN_POINT('Ctrl Pts',(97.5309980386224,-126.9104585261,508.462296651428));
#272404=CARTESIAN_POINT('Ctrl Pts',(87.5429283387234,-134.586314540048,
506.462296651428));
#272405=CARTESIAN_POINT('Ctrl Pts',(76.4770599218137,-140.605189688823,
504.462296651428));
#272406=CARTESIAN_POINT('Ctrl Pts',(65.4111915049041,-146.624064837599,
502.462296651428));
#272407=CARTESIAN_POINT('Ctrl Pts',(53.5400027769198,-150.837754439537,
500.462296651428));
#272408=CARTESIAN_POINT('Ctrl Pts',(41.6688140489356,-155.051444041475,
498.462296651428));
#272409=CARTESIAN_POINT('Ctrl Pts',(29.2846130745764,-157.356193074143,
496.462296651428));
#272410=CARTESIAN_POINT('Ctrl Pts',(16.9004121002171,-159.660942106811,
494.462296651428));
#272411=CARTESIAN_POINT('Ctrl Pts',(4.30813900827814,-160.,492.462296651428));
#272412=CARTESIAN_POINT('Ctrl Pts',(-8.28413408366082,-160.339057893189,
490.462296651428));
#272413=CARTESIAN_POINT('Ctrl Pts',(-20.7744157382975,-158.704075916301,
488.462296651428));
#272414=CARTESIAN_POINT('Ctrl Pts',(-33.2646973929342,-157.069093939413,
486.462296651428));
#272415=CARTESIAN_POINT('Ctrl Pts',(-45.3454354230633,-153.500330774912,
484.462296651428));
#272416=CARTESIAN_POINT('Ctrl Pts',(-57.4261734531924,-149.931567610412,
482.462296651428));
#272417=CARTESIAN_POINT('Ctrl Pts',(-68.7998999948413,-144.516898051455,
480.462296651428));
#272418=CARTESIAN_POINT('Ctrl Pts',(-80.1736265364901,-139.102228492497,
478.462296651428));
#272419=CARTESIAN_POINT('Ctrl Pts',(-90.5602826949691,-131.974979673883,
476.462296651428));
#272420=CARTESIAN_POINT('Ctrl Pts',(-100.946938853448,-124.847730855269,
474.462296651428));
#272421=CARTESIAN_POINT('Ctrl Pts',(-110.0907706828,-116.183399296895,472.462296651428));
#272422=CARTESIAN_POINT('Ctrl Pts',(-119.234602512152,-107.519067738521,
470.462296651428));
#272423=CARTESIAN_POINT('Ctrl Pts',(-126.9104585261,-97.5309980386224,468.462296651428));
#272424=CARTESIAN_POINT('Ctrl Pts',(-134.586314540048,-87.5429283387234,
466.462296651428));
#272425=CARTESIAN_POINT('Ctrl Pts',(-140.605189688823,-76.4770599218137,
464.462296651428));
#272426=CARTESIAN_POINT('Ctrl Pts',(-146.624064837599,-65.4111915049041,
462.462296651428));
#272427=CARTESIAN_POINT('Ctrl Pts',(-150.837754439537,-53.5400027769199,
460.462296651428));
#272428=CARTESIAN_POINT('Ctrl Pts',(-155.051444041475,-41.6688140489356,
458.462296651428));
#272429=CARTESIAN_POINT('Ctrl Pts',(-157.356193074143,-29.2846130745764,
456.462296651428));
#272430=CARTESIAN_POINT('Ctrl Pts',(-159.660942106811,-16.9004121002171,
454.462296651429));
#272431=CARTESIAN_POINT('Ctrl Pts',(-160.,-4.30813900827815,452.462296651428));
#272432=CARTESIAN_POINT('Ctrl Pts',(-160.339057893189,8.28413408366081,
450.462296651428));
#272433=CARTESIAN_POINT('Ctrl Pts',(-158.704075916301,20.7744157382975,
448.462296651428));
#272434=CARTESIAN_POINT('Ctrl Pts',(-157.069093939413,33.2646973929342,
446.462296651428));
#272435=CARTESIAN_POINT('Ctrl Pts',(-153.500330774912,45.3454354230633,
444.462296651428));
#272436=CARTESIAN_POINT('Ctrl Pts',(-149.931567610412,57.4261734531924,
442.462296651428));
#272437=CARTESIAN_POINT('Ctrl Pts',(-144.516898051455,68.7998999948413,
440.462296651428));
#272438=CARTESIAN_POINT('Ctrl Pts',(-139.102228492497,80.1736265364901,
438.462296651428));
#272439=CARTESIAN_POINT('Ctrl Pts',(-131.974979673883,90.5602826949691,
436.462296651428));
#272440=CARTESIAN_POINT('Ctrl Pts',(-124.847730855269,100.946938853448,
434.462296651428));
#272441=CARTESIAN_POINT('Ctrl Pts',(-116.183399296895,110.0907706828,432.462296651428));
#272442=CARTESIAN_POINT('Ctrl Pts',(-107.519067738521,119.234602512152,
430.462296651428));
#272443=CARTESIAN_POINT('Ctrl Pts',(-97.5309980386224,126.9104585261,428.462296651428));
#272444=CARTESIAN_POINT('Ctrl Pts',(-87.5429283387233,134.586314540048,
426.462296651428));
#272445=CARTESIAN_POINT('Ctrl Pts',(-76.4770599218137,140.605189688823,
424.462296651428));
#272446=CARTESIAN_POINT('Ctrl Pts',(-65.4111915049042,146.624064837599,
422.462296651428));
#272447=CARTESIAN_POINT('Ctrl Pts',(-53.5400027769199,150.837754439537,
420.462296651428));
#272448=CARTESIAN_POINT('Ctrl Pts',(-41.6688140489356,155.051444041475,
418.462296651428));
#272449=CARTESIAN_POINT('Ctrl Pts',(-29.2846130745764,157.356193074143,
416.462296651428));
#272450=CARTESIAN_POINT('Ctrl Pts',(-16.9004121002172,159.660942106811,
414.462296651428));
#272451=CARTESIAN_POINT('Ctrl Pts',(-4.30813900827816,160.,412.462296651428));
#272452=CARTESIAN_POINT('Ctrl Pts',(8.28413408366087,160.339057893189,410.462296651428));
#272453=CARTESIAN_POINT('Ctrl Pts',(20.7744157382975,158.704075916301,408.462296651428));
#272454=CARTESIAN_POINT('Ctrl Pts',(33.2646973929342,157.069093939413,406.462296651428));
#272455=CARTESIAN_POINT('Ctrl Pts',(45.3454354230633,153.500330774912,404.462296651428));
#272456=CARTESIAN_POINT('Ctrl Pts',(57.4261734531925,149.931567610412,402.462296651428));
#272457=CARTESIAN_POINT('Ctrl Pts',(68.7998999948413,144.516898051455,400.462296651428));
#272458=CARTESIAN_POINT('Ctrl Pts',(80.1736265364901,139.102228492498,398.462296651428));
#272459=CARTESIAN_POINT('Ctrl Pts',(90.560282694969,131.974979673883,396.462296651428));
#272460=CARTESIAN_POINT('Ctrl Pts',(100.946938853448,124.847730855269,394.462296651428));
#272461=CARTESIAN_POINT('Ctrl Pts',(110.0907706828,116.183399296895,392.462296651428));
#272462=CARTESIAN_POINT('Ctrl Pts',(119.234602512152,107.519067738521,390.462296651428));
#272463=CARTESIAN_POINT('Ctrl Pts',(126.9104585261,97.5309980386224,388.462296651428));
#272464=CARTESIAN_POINT('Ctrl Pts',(134.586314540048,87.5429283387233,386.462296651428));
#272465=CARTESIAN_POINT('Ctrl Pts',(140.605189688823,76.4770599218137,384.462296651428));
#272466=CARTESIAN_POINT('Ctrl Pts',(146.624064837599,65.4111915049042,382.462296651428));
#272467=CARTESIAN_POINT('Ctrl Pts',(150.837754439537,53.5400027769199,380.462296651428));
#272468=CARTESIAN_POINT('Ctrl Pts',(155.051444041475,41.6688140489356,378.462296651428));
#272469=CARTESIAN_POINT('Ctrl Pts',(157.356193074143,29.2846130745764,376.462296651428));
#272470=CARTESIAN_POINT('Ctrl Pts',(159.660942106811,16.9004121002172,374.462296651428));
#272471=CARTESIAN_POINT('Ctrl Pts',(160.,4.30813900827813,372.462296651428));
#272472=CARTESIAN_POINT('Ctrl Pts',(160.,-4.30813900827805,537.537703348572));
#272473=CARTESIAN_POINT('Ctrl Pts',(159.660942106811,-16.900412100217,535.537703348572));
#272474=CARTESIAN_POINT('Ctrl Pts',(157.356193074143,-29.2846130745763,
533.537703348572));
#272475=CARTESIAN_POINT('Ctrl Pts',(155.051444041475,-41.6688140489355,
531.537703348572));
#272476=CARTESIAN_POINT('Ctrl Pts',(150.837754439537,-53.5400027769198,
529.537703348572));
#272477=CARTESIAN_POINT('Ctrl Pts',(146.624064837599,-65.411191504904,527.537703348572));
#272478=CARTESIAN_POINT('Ctrl Pts',(140.605189688823,-76.4770599218136,
525.537703348572));
#272479=CARTESIAN_POINT('Ctrl Pts',(134.586314540048,-87.5429283387233,
523.537703348572));
#272480=CARTESIAN_POINT('Ctrl Pts',(126.9104585261,-97.5309980386223,521.537703348572));
#272481=CARTESIAN_POINT('Ctrl Pts',(119.234602512152,-107.519067738521,
519.537703348572));
#272482=CARTESIAN_POINT('Ctrl Pts',(110.0907706828,-116.183399296895,517.537703348572));
#272483=CARTESIAN_POINT('Ctrl Pts',(100.946938853448,-124.847730855269,
515.537703348572));
#272484=CARTESIAN_POINT('Ctrl Pts',(90.5602826949691,-131.974979673883,
513.537703348572));
#272485=CARTESIAN_POINT('Ctrl Pts',(80.1736265364902,-139.102228492497,
511.537703348572));
#272486=CARTESIAN_POINT('Ctrl Pts',(68.7998999948414,-144.516898051454,
509.537703348572));
#272487=CARTESIAN_POINT('Ctrl Pts',(57.4261734531925,-149.931567610412,
507.537703348572));
#272488=CARTESIAN_POINT('Ctrl Pts',(45.3454354230634,-153.500330774912,
505.537703348572));
#272489=CARTESIAN_POINT('Ctrl Pts',(33.2646973929343,-157.069093939413,
503.537703348572));
#272490=CARTESIAN_POINT('Ctrl Pts',(20.7744157382976,-158.704075916301,
501.537703348572));
#272491=CARTESIAN_POINT('Ctrl Pts',(8.28413408366091,-160.339057893189,
499.537703348572));
#272492=CARTESIAN_POINT('Ctrl Pts',(-4.30813900827804,-160.,497.537703348572));
#272493=CARTESIAN_POINT('Ctrl Pts',(-16.900412100217,-159.660942106811,
495.537703348572));
#272494=CARTESIAN_POINT('Ctrl Pts',(-29.2846130745763,-157.356193074143,
493.537703348572));
#272495=CARTESIAN_POINT('Ctrl Pts',(-41.6688140489355,-155.051444041475,
491.537703348572));
#272496=CARTESIAN_POINT('Ctrl Pts',(-53.5400027769198,-150.837754439537,
489.537703348572));
#272497=CARTESIAN_POINT('Ctrl Pts',(-65.411191504904,-146.624064837599,
487.537703348572));
#272498=CARTESIAN_POINT('Ctrl Pts',(-76.4770599218136,-140.605189688823,
485.537703348572));
#272499=CARTESIAN_POINT('Ctrl Pts',(-87.5429283387233,-134.586314540048,
483.537703348572));
#272500=CARTESIAN_POINT('Ctrl Pts',(-97.5309980386223,-126.9104585261,481.537703348572));
#272501=CARTESIAN_POINT('Ctrl Pts',(-107.519067738521,-119.234602512152,
479.537703348572));
#272502=CARTESIAN_POINT('Ctrl Pts',(-116.183399296895,-110.0907706828,477.537703348572));
#272503=CARTESIAN_POINT('Ctrl Pts',(-124.847730855269,-100.946938853448,
475.537703348572));
#272504=CARTESIAN_POINT('Ctrl Pts',(-131.974979673883,-90.5602826949692,
473.537703348572));
#272505=CARTESIAN_POINT('Ctrl Pts',(-139.102228492497,-80.1736265364902,
471.537703348572));
#272506=CARTESIAN_POINT('Ctrl Pts',(-144.516898051454,-68.7998999948414,
469.537703348572));
#272507=CARTESIAN_POINT('Ctrl Pts',(-149.931567610412,-57.4261734531925,
467.537703348572));
#272508=CARTESIAN_POINT('Ctrl Pts',(-153.500330774912,-45.3454354230634,
465.537703348572));
#272509=CARTESIAN_POINT('Ctrl Pts',(-157.069093939413,-33.2646973929344,
463.537703348572));
#272510=CARTESIAN_POINT('Ctrl Pts',(-158.704075916301,-20.7744157382976,
461.537703348572));
#272511=CARTESIAN_POINT('Ctrl Pts',(-160.339057893189,-8.28413408366092,
459.537703348572));
#272512=CARTESIAN_POINT('Ctrl Pts',(-160.,4.30813900827803,457.537703348572));
#272513=CARTESIAN_POINT('Ctrl Pts',(-159.660942106811,16.900412100217,455.537703348572));
#272514=CARTESIAN_POINT('Ctrl Pts',(-157.356193074143,29.2846130745763,
453.537703348572));
#272515=CARTESIAN_POINT('Ctrl Pts',(-155.051444041475,41.6688140489355,
451.537703348572));
#272516=CARTESIAN_POINT('Ctrl Pts',(-150.837754439537,53.5400027769198,
449.537703348572));
#272517=CARTESIAN_POINT('Ctrl Pts',(-146.624064837599,65.411191504904,447.537703348572));
#272518=CARTESIAN_POINT('Ctrl Pts',(-140.605189688823,76.4770599218136,
445.537703348572));
#272519=CARTESIAN_POINT('Ctrl Pts',(-134.586314540048,87.5429283387233,
443.537703348572));
#272520=CARTESIAN_POINT('Ctrl Pts',(-126.9104585261,97.5309980386223,441.537703348572));
#272521=CARTESIAN_POINT('Ctrl Pts',(-119.234602512152,107.519067738521,
439.537703348572));
#272522=CARTESIAN_POINT('Ctrl Pts',(-110.0907706828,116.183399296895,437.537703348572));
#272523=CARTESIAN_POINT('Ctrl Pts',(-100.946938853448,124.847730855269,
435.537703348572));
#272524=CARTESIAN_POINT('Ctrl Pts',(-90.5602826949692,131.974979673883,
433.537703348572));
#272525=CARTESIAN_POINT('Ctrl Pts',(-80.1736265364901,139.102228492497,
431.537703348572));
#272526=CARTESIAN_POINT('Ctrl Pts',(-68.7998999948414,144.516898051454,
429.537703348572));
#272527=CARTESIAN_POINT('Ctrl Pts',(-57.4261734531926,149.931567610412,
427.537703348572));
#272528=CARTESIAN_POINT('Ctrl Pts',(-45.3454354230634,153.500330774912,
425.537703348572));
#272529=CARTESIAN_POINT('Ctrl Pts',(-33.2646973929343,157.069093939413,
423.537703348572));
#272530=CARTESIAN_POINT('Ctrl Pts',(-20.7744157382976,158.704075916301,
421.537703348572));
#272531=CARTESIAN_POINT('Ctrl Pts',(-8.284134083661,160.339057893189,419.537703348572));
#272532=CARTESIAN_POINT('Ctrl Pts',(4.30813900827803,160.,417.537703348572));
#272533=CARTESIAN_POINT('Ctrl Pts',(16.9004121002171,159.660942106811,415.537703348572));
#272534=CARTESIAN_POINT('Ctrl Pts',(29.2846130745762,157.356193074143,413.537703348572));
#272535=CARTESIAN_POINT('Ctrl Pts',(41.6688140489354,155.051444041476,411.537703348572));
#272536=CARTESIAN_POINT('Ctrl Pts',(53.5400027769198,150.837754439537,409.537703348572));
#272537=CARTESIAN_POINT('Ctrl Pts',(65.4111915049041,146.624064837599,407.537703348572));
#272538=CARTESIAN_POINT('Ctrl Pts',(76.4770599218136,140.605189688823,405.537703348572));
#272539=CARTESIAN_POINT('Ctrl Pts',(87.5429283387232,134.586314540048,403.537703348572));
#272540=CARTESIAN_POINT('Ctrl Pts',(97.5309980386223,126.9104585261,401.537703348572));
#272541=CARTESIAN_POINT('Ctrl Pts',(107.519067738521,119.234602512152,399.537703348572));
#272542=CARTESIAN_POINT('Ctrl Pts',(116.183399296895,110.0907706828,397.537703348572));
#272543=CARTESIAN_POINT('Ctrl Pts',(124.847730855269,100.946938853448,395.537703348572));
#272544=CARTESIAN_POINT('Ctrl Pts',(131.974979673883,90.5602826949692,393.537703348572));
#272545=CARTESIAN_POINT('Ctrl Pts',(139.102228492497,80.1736265364902,391.537703348572));
#272546=CARTESIAN_POINT('Ctrl Pts',(144.516898051454,68.7998999948414,389.537703348572));
#272547=CARTESIAN_POINT('Ctrl Pts',(149.931567610412,57.4261734531926,387.537703348572));
#272548=CARTESIAN_POINT('Ctrl Pts',(153.500330774912,45.3454354230634,385.537703348572));
#272549=CARTESIAN_POINT('Ctrl Pts',(157.069093939413,33.2646973929343,383.537703348572));
#272550=CARTESIAN_POINT('Ctrl Pts',(158.704075916301,20.7744157382976,381.537703348572));
#272551=CARTESIAN_POINT('Ctrl Pts',(160.339057893189,8.28413408366101,379.537703348572));
#272552=CARTESIAN_POINT('Ctrl Pts',(160.,-4.30813900827805,377.537703348572));
#272553=CARTESIAN_POINT('Origin',(-4.03737035478301,-0.209103844006933,
379.537622607614));
#272554=CARTESIAN_POINT('Ctrl Pts',(160.,-4.30813900827805,537.537703348572));
#272555=CARTESIAN_POINT('Ctrl Pts',(159.660942106811,-16.900412100217,535.537703348572));
#272556=CARTESIAN_POINT('Ctrl Pts',(157.356193074143,-29.2846130745763,
533.537703348572));
#272557=CARTESIAN_POINT('Ctrl Pts',(155.051444041475,-41.6688140489355,
531.537703348572));
#272558=CARTESIAN_POINT('Ctrl Pts',(150.837754439537,-53.5400027769198,
529.537703348572));
#272559=CARTESIAN_POINT('Ctrl Pts',(146.624064837599,-65.411191504904,527.537703348572));
#272560=CARTESIAN_POINT('Ctrl Pts',(140.605189688823,-76.4770599218136,
525.537703348572));
#272561=CARTESIAN_POINT('Ctrl Pts',(134.586314540048,-87.5429283387233,
523.537703348572));
#272562=CARTESIAN_POINT('Ctrl Pts',(126.9104585261,-97.5309980386223,521.537703348572));
#272563=CARTESIAN_POINT('Ctrl Pts',(119.234602512152,-107.519067738521,
519.537703348572));
#272564=CARTESIAN_POINT('Ctrl Pts',(110.0907706828,-116.183399296895,517.537703348572));
#272565=CARTESIAN_POINT('Ctrl Pts',(100.946938853448,-124.847730855269,
515.537703348572));
#272566=CARTESIAN_POINT('Ctrl Pts',(90.5602826949691,-131.974979673883,
513.537703348572));
#272567=CARTESIAN_POINT('Ctrl Pts',(80.1736265364902,-139.102228492497,
511.537703348572));
#272568=CARTESIAN_POINT('Ctrl Pts',(68.7998999948414,-144.516898051454,
509.537703348572));
#272569=CARTESIAN_POINT('Ctrl Pts',(57.4261734531925,-149.931567610412,
507.537703348572));
#272570=CARTESIAN_POINT('Ctrl Pts',(45.3454354230634,-153.500330774912,
505.537703348572));
#272571=CARTESIAN_POINT('Ctrl Pts',(33.2646973929343,-157.069093939413,
503.537703348572));
#272572=CARTESIAN_POINT('Ctrl Pts',(20.7744157382976,-158.704075916301,
501.537703348572));
#272573=CARTESIAN_POINT('Ctrl Pts',(8.28413408366091,-160.339057893189,
499.537703348572));
#272574=CARTESIAN_POINT('Ctrl Pts',(-4.30813900827804,-160.,497.537703348572));
#272575=CARTESIAN_POINT('Ctrl Pts',(-16.900412100217,-159.660942106811,
495.537703348572));
#272576=CARTESIAN_POINT('Ctrl Pts',(-29.2846130745763,-157.356193074143,
493.537703348572));
#272577=CARTESIAN_POINT('Ctrl Pts',(-41.6688140489355,-155.051444041475,
491.537703348572));
#272578=CARTESIAN_POINT('Ctrl Pts',(-53.5400027769198,-150.837754439537,
489.537703348572));
#272579=CARTESIAN_POINT('Ctrl Pts',(-65.411191504904,-146.624064837599,
487.537703348572));
#272580=CARTESIAN_POINT('Ctrl Pts',(-76.4770599218136,-140.605189688823,
485.537703348572));
#272581=CARTESIAN_POINT('Ctrl Pts',(-87.5429283387233,-134.586314540048,
483.537703348572));
#272582=CARTESIAN_POINT('Ctrl Pts',(-97.5309980386223,-126.9104585261,481.537703348572));
#272583=CARTESIAN_POINT('Ctrl Pts',(-107.519067738521,-119.234602512152,
479.537703348572));
#272584=CARTESIAN_POINT('Ctrl Pts',(-116.183399296895,-110.0907706828,477.537703348572));
#272585=CARTESIAN_POINT('Ctrl Pts',(-124.847730855269,-100.946938853448,
475.537703348572));
#272586=CARTESIAN_POINT('Ctrl Pts',(-131.974979673883,-90.5602826949692,
473.537703348572));
#272587=CARTESIAN_POINT('Ctrl Pts',(-139.102228492497,-80.1736265364902,
471.537703348572));
#272588=CARTESIAN_POINT('Ctrl Pts',(-144.516898051454,-68.7998999948414,
469.537703348572));
#272589=CARTESIAN_POINT('Ctrl Pts',(-149.931567610412,-57.4261734531925,
467.537703348572));
#272590=CARTESIAN_POINT('Ctrl Pts',(-153.500330774912,-45.3454354230634,
465.537703348572));
#272591=CARTESIAN_POINT('Ctrl Pts',(-157.069093939413,-33.2646973929344,
463.537703348572));
#272592=CARTESIAN_POINT('Ctrl Pts',(-158.704075916301,-20.7744157382976,
461.537703348572));
#272593=CARTESIAN_POINT('Ctrl Pts',(-160.339057893189,-8.28413408366092,
459.537703348572));
#272594=CARTESIAN_POINT('Ctrl Pts',(-160.,4.30813900827803,457.537703348572));
#272595=CARTESIAN_POINT('Ctrl Pts',(-159.660942106811,16.900412100217,455.537703348572));
#272596=CARTESIAN_POINT('Ctrl Pts',(-157.356193074143,29.2846130745763,
453.537703348572));
#272597=CARTESIAN_POINT('Ctrl Pts',(-155.051444041475,41.6688140489355,
451.537703348572));
#272598=CARTESIAN_POINT('Ctrl Pts',(-150.837754439537,53.5400027769198,
449.537703348572));
#272599=CARTESIAN_POINT('Ctrl Pts',(-146.624064837599,65.411191504904,447.537703348572));
#272600=CARTESIAN_POINT('Ctrl Pts',(-140.605189688823,76.4770599218136,
445.537703348572));
#272601=CARTESIAN_POINT('Ctrl Pts',(-134.586314540048,87.5429283387233,
443.537703348572));
#272602=CARTESIAN_POINT('Ctrl Pts',(-126.9104585261,97.5309980386223,441.537703348572));
#272603=CARTESIAN_POINT('Ctrl Pts',(-119.234602512152,107.519067738521,
439.537703348572));
#272604=CARTESIAN_POINT('Ctrl Pts',(-110.0907706828,116.183399296895,437.537703348572));
#272605=CARTESIAN_POINT('Ctrl Pts',(-100.946938853448,124.847730855269,
435.537703348572));
#272606=CARTESIAN_POINT('Ctrl Pts',(-90.5602826949692,131.974979673883,
433.537703348572));
#272607=CARTESIAN_POINT('Ctrl Pts',(-80.1736265364901,139.102228492497,
431.537703348572));
#272608=CARTESIAN_POINT('Ctrl Pts',(-68.7998999948414,144.516898051454,
429.537703348572));
#272609=CARTESIAN_POINT('Ctrl Pts',(-57.4261734531926,149.931567610412,
427.537703348572));
#272610=CARTESIAN_POINT('Ctrl Pts',(-45.3454354230634,153.500330774912,
425.537703348572));
#272611=CARTESIAN_POINT('Ctrl Pts',(-33.2646973929343,157.069093939413,
423.537703348572));
#272612=CARTESIAN_POINT('Ctrl Pts',(-20.7744157382976,158.704075916301,
421.537703348572));
#272613=CARTESIAN_POINT('Ctrl Pts',(-8.284134083661,160.339057893189,419.537703348572));
#272614=CARTESIAN_POINT('Ctrl Pts',(4.30813900827803,160.,417.537703348572));
#272615=CARTESIAN_POINT('Ctrl Pts',(16.9004121002171,159.660942106811,415.537703348572));
#272616=CARTESIAN_POINT('Ctrl Pts',(29.2846130745762,157.356193074143,413.537703348572));
#272617=CARTESIAN_POINT('Ctrl Pts',(41.6688140489354,155.051444041476,411.537703348572));
#272618=CARTESIAN_POINT('Ctrl Pts',(53.5400027769198,150.837754439537,409.537703348572));
#272619=CARTESIAN_POINT('Ctrl Pts',(65.4111915049041,146.624064837599,407.537703348572));
#272620=CARTESIAN_POINT('Ctrl Pts',(76.4770599218136,140.605189688823,405.537703348572));
#272621=CARTESIAN_POINT('Ctrl Pts',(87.5429283387232,134.586314540048,403.537703348572));
#272622=CARTESIAN_POINT('Ctrl Pts',(97.5309980386223,126.9104585261,401.537703348572));
#272623=CARTESIAN_POINT('Ctrl Pts',(107.519067738521,119.234602512152,399.537703348572));
#272624=CARTESIAN_POINT('Ctrl Pts',(116.183399296895,110.0907706828,397.537703348572));
#272625=CARTESIAN_POINT('Ctrl Pts',(124.847730855269,100.946938853448,395.537703348572));
#272626=CARTESIAN_POINT('Ctrl Pts',(131.974979673883,90.5602826949692,393.537703348572));
#272627=CARTESIAN_POINT('Ctrl Pts',(139.102228492497,80.1736265364902,391.537703348572));
#272628=CARTESIAN_POINT('Ctrl Pts',(144.516898051454,68.7998999948414,389.537703348572));
#272629=CARTESIAN_POINT('Ctrl Pts',(149.931567610412,57.4261734531926,387.537703348572));
#272630=CARTESIAN_POINT('Ctrl Pts',(153.500330774912,45.3454354230634,385.537703348572));
#272631=CARTESIAN_POINT('Ctrl Pts',(157.069093939413,33.2646973929343,383.537703348572));
#272632=CARTESIAN_POINT('Ctrl Pts',(158.704075916301,20.7744157382976,381.537703348572));
#272633=CARTESIAN_POINT('Ctrl Pts',(160.339057893189,8.28413408366101,379.537703348572));
#272634=CARTESIAN_POINT('Ctrl Pts',(160.,-4.30813900827805,377.537703348572));
#272635=CARTESIAN_POINT('Ctrl Pts',(130.,-4.30813900827807,537.537703348572));
#272636=CARTESIAN_POINT('Ctrl Pts',(129.660942106811,-14.5393608954785,
535.537703348572));
#272637=CARTESIAN_POINT('Ctrl Pts',(127.725542856289,-24.5915791233694,
533.537703348572));
#272638=CARTESIAN_POINT('Ctrl Pts',(125.790143605767,-34.6437973512603,
531.537703348572));
#272639=CARTESIAN_POINT('Ctrl Pts',(122.306058950682,-44.2694929456714,
529.537703348572));
#272640=CARTESIAN_POINT('Ctrl Pts',(118.821974295598,-53.8951885400825,
527.537703348572));
#272641=CARTESIAN_POINT('Ctrl Pts',(113.874993963172,-62.8573449296272,
525.537703348572));
#272642=CARTESIAN_POINT('Ctrl Pts',(108.928013630747,-71.819501319172,523.537703348572));
#272643=CARTESIAN_POINT('Ctrl Pts',(102.639948694851,-79.8974404698481,
521.537703348572));
#272644=CARTESIAN_POINT('Ctrl Pts',(96.351883758956,-87.9753796205242,519.537703348572));
#272645=CARTESIAN_POINT('Ctrl Pts',(88.8775672472035,-94.9701958612989,
517.537703348572));
#272646=CARTESIAN_POINT('Ctrl Pts',(81.403250735451,-101.965012102074,515.537703348572));
#272647=CARTESIAN_POINT('Ctrl Pts',(72.9267251261949,-107.704469842635,
513.537703348572));
#272648=CARTESIAN_POINT('Ctrl Pts',(64.4501995169389,-113.443927583196,
511.537703348572));
#272649=CARTESIAN_POINT('Ctrl Pts',(55.1801850026549,-117.786702325803,
509.537703348572));
#272650=CARTESIAN_POINT('Ctrl Pts',(45.910170488371,-122.129477068411,507.537703348572));
#272651=CARTESIAN_POINT('Ctrl Pts',(36.074925591815,-124.968635286058,505.537703348572));
#272652=CARTESIAN_POINT('Ctrl Pts',(26.239680695259,-127.807793503704,503.537703348572));
#272653=CARTESIAN_POINT('Ctrl Pts',(16.0813817870907,-129.073425698447,
501.537703348572));
#272654=CARTESIAN_POINT('Ctrl Pts',(5.92308287892234,-130.339057893189,
499.537703348572));
#272655=CARTESIAN_POINT('Ctrl Pts',(-4.30813900827806,-130.,497.537703348572));
#272656=CARTESIAN_POINT('Ctrl Pts',(-14.5393608954785,-129.660942106811,
495.537703348572));
#272657=CARTESIAN_POINT('Ctrl Pts',(-24.5915791233694,-127.725542856289,
493.537703348572));
#272658=CARTESIAN_POINT('Ctrl Pts',(-34.6437973512603,-125.790143605767,
491.537703348572));
#272659=CARTESIAN_POINT('Ctrl Pts',(-44.2694929456713,-122.306058950682,
489.537703348572));
#272660=CARTESIAN_POINT('Ctrl Pts',(-53.8951885400825,-118.821974295598,
487.537703348572));
#272661=CARTESIAN_POINT('Ctrl Pts',(-62.8573449296272,-113.874993963172,
485.537703348572));
#272662=CARTESIAN_POINT('Ctrl Pts',(-71.819501319172,-108.928013630747,
483.537703348572));
#272663=CARTESIAN_POINT('Ctrl Pts',(-79.8974404698481,-102.639948694851,
481.537703348572));
#272664=CARTESIAN_POINT('Ctrl Pts',(-87.9753796205242,-96.351883758956,
479.537703348572));
#272665=CARTESIAN_POINT('Ctrl Pts',(-94.9701958612989,-88.8775672472035,
477.537703348572));
#272666=CARTESIAN_POINT('Ctrl Pts',(-101.965012102074,-81.403250735451,
475.537703348572));
#272667=CARTESIAN_POINT('Ctrl Pts',(-107.704469842635,-72.9267251261949,
473.537703348572));
#272668=CARTESIAN_POINT('Ctrl Pts',(-113.443927583196,-64.4501995169389,
471.537703348572));
#272669=CARTESIAN_POINT('Ctrl Pts',(-117.786702325803,-55.1801850026549,
469.537703348572));
#272670=CARTESIAN_POINT('Ctrl Pts',(-122.129477068411,-45.910170488371,
467.537703348572));
#272671=CARTESIAN_POINT('Ctrl Pts',(-124.968635286058,-36.074925591815,
465.537703348572));
#272672=CARTESIAN_POINT('Ctrl Pts',(-127.807793503704,-26.239680695259,
463.537703348572));
#272673=CARTESIAN_POINT('Ctrl Pts',(-129.073425698447,-16.0813817870907,
461.537703348572));
#272674=CARTESIAN_POINT('Ctrl Pts',(-130.339057893189,-5.92308287892235,
459.537703348572));
#272675=CARTESIAN_POINT('Ctrl Pts',(-130.,4.30813900827805,457.537703348572));
#272676=CARTESIAN_POINT('Ctrl Pts',(-129.660942106811,14.5393608954784,
455.537703348572));
#272677=CARTESIAN_POINT('Ctrl Pts',(-127.725542856289,24.5915791233693,
453.537703348572));
#272678=CARTESIAN_POINT('Ctrl Pts',(-125.790143605767,34.6437973512602,
451.537703348572));
#272679=CARTESIAN_POINT('Ctrl Pts',(-122.306058950682,44.2694929456713,
449.537703348572));
#272680=CARTESIAN_POINT('Ctrl Pts',(-118.821974295598,53.8951885400825,
447.537703348572));
#272681=CARTESIAN_POINT('Ctrl Pts',(-113.874993963172,62.8573449296272,
445.537703348572));
#272682=CARTESIAN_POINT('Ctrl Pts',(-108.928013630747,71.819501319172,443.537703348572));
#272683=CARTESIAN_POINT('Ctrl Pts',(-102.639948694851,79.8974404698481,
441.537703348572));
#272684=CARTESIAN_POINT('Ctrl Pts',(-96.3518837589561,87.9753796205242,
439.537703348572));
#272685=CARTESIAN_POINT('Ctrl Pts',(-88.8775672472035,94.9701958612989,
437.537703348572));
#272686=CARTESIAN_POINT('Ctrl Pts',(-81.403250735451,101.965012102074,435.537703348572));
#272687=CARTESIAN_POINT('Ctrl Pts',(-72.9267251261949,107.704469842635,
433.537703348572));
#272688=CARTESIAN_POINT('Ctrl Pts',(-64.4501995169389,113.443927583196,
431.537703348572));
#272689=CARTESIAN_POINT('Ctrl Pts',(-55.1801850026549,117.786702325803,
429.537703348572));
#272690=CARTESIAN_POINT('Ctrl Pts',(-45.910170488371,122.129477068411,427.537703348572));
#272691=CARTESIAN_POINT('Ctrl Pts',(-36.074925591815,124.968635286058,425.537703348572));
#272692=CARTESIAN_POINT('Ctrl Pts',(-26.239680695259,127.807793503704,423.537703348572));
#272693=CARTESIAN_POINT('Ctrl Pts',(-16.0813817870907,129.073425698447,
421.537703348572));
#272694=CARTESIAN_POINT('Ctrl Pts',(-5.92308287892242,130.339057893189,
419.537703348572));
#272695=CARTESIAN_POINT('Ctrl Pts',(4.30813900827804,130.,417.537703348572));
#272696=CARTESIAN_POINT('Ctrl Pts',(14.5393608954785,129.660942106811,415.537703348572));
#272697=CARTESIAN_POINT('Ctrl Pts',(24.5915791233693,127.725542856289,413.537703348572));
#272698=CARTESIAN_POINT('Ctrl Pts',(34.6437973512602,125.790143605767,411.537703348572));
#272699=CARTESIAN_POINT('Ctrl Pts',(44.2694929456713,122.306058950682,409.537703348572));
#272700=CARTESIAN_POINT('Ctrl Pts',(53.8951885400825,118.821974295598,407.537703348572));
#272701=CARTESIAN_POINT('Ctrl Pts',(62.8573449296272,113.874993963172,405.537703348572));
#272702=CARTESIAN_POINT('Ctrl Pts',(71.819501319172,108.928013630747,403.537703348572));
#272703=CARTESIAN_POINT('Ctrl Pts',(79.8974404698481,102.639948694851,401.537703348572));
#272704=CARTESIAN_POINT('Ctrl Pts',(87.9753796205242,96.351883758956,399.537703348572));
#272705=CARTESIAN_POINT('Ctrl Pts',(94.9701958612989,88.8775672472035,397.537703348572));
#272706=CARTESIAN_POINT('Ctrl Pts',(101.965012102074,81.403250735451,395.537703348572));
#272707=CARTESIAN_POINT('Ctrl Pts',(107.704469842635,72.926725126195,393.537703348572));
#272708=CARTESIAN_POINT('Ctrl Pts',(113.443927583196,64.4501995169389,391.537703348572));
#272709=CARTESIAN_POINT('Ctrl Pts',(117.786702325803,55.1801850026549,389.537703348572));
#272710=CARTESIAN_POINT('Ctrl Pts',(122.129477068411,45.910170488371,387.537703348572));
#272711=CARTESIAN_POINT('Ctrl Pts',(124.968635286058,36.074925591815,385.537703348572));
#272712=CARTESIAN_POINT('Ctrl Pts',(127.807793503704,26.239680695259,383.537703348572));
#272713=CARTESIAN_POINT('Ctrl Pts',(129.073425698447,16.0813817870907,381.537703348572));
#272714=CARTESIAN_POINT('Ctrl Pts',(130.339057893189,5.92308287892242,379.537703348572));
#272715=CARTESIAN_POINT('Ctrl Pts',(130.,-4.30813900827807,377.537703348572));
#272716=CARTESIAN_POINT('Origin',(160.,-1.08084483543429E-12,695.));
#272717=CARTESIAN_POINT('',(160.,4.30813900827813,692.462296651428));
#272718=CARTESIAN_POINT('',(160.,-4.3081390082785,691.09188778474));
#272719=CARTESIAN_POINT('Ctrl Pts',(160.,4.30813900827813,692.462296651428));
#272720=CARTESIAN_POINT('Ctrl Pts',(160.,1.43594781991678,692.006113535419));
#272721=CARTESIAN_POINT('Ctrl Pts',(160.,-1.43604209808348,691.54866409354));
#272722=CARTESIAN_POINT('Ctrl Pts',(160.,-4.3081390082785,691.09188778474));
#272723=CARTESIAN_POINT('',(160.,-2.89658996530608E-13,695.));
#272724=CARTESIAN_POINT('Ctrl Pts',(160.,-4.3081390082785,691.09188778474));
#272725=CARTESIAN_POINT('Ctrl Pts',(160.,-2.89215276710194,692.376694251499));
#272726=CARTESIAN_POINT('Ctrl Pts',(160.,-1.47617978718644,693.661515452264));
#272727=CARTESIAN_POINT('Ctrl Pts',(160.,-0.0597455111855364,694.945827966412));
#272728=CARTESIAN_POINT('Ctrl Pts',(160.,-0.0398304324249309,694.963885412003));
#272729=CARTESIAN_POINT('Ctrl Pts',(160.,-0.0199151703953438,694.981942655471));
#272730=CARTESIAN_POINT('Ctrl Pts',(160.,-3.33066907387547E-13,695.));
#272731=CARTESIAN_POINT('',(160.,3.64291929955129E-14,695.));
#272732=CARTESIAN_POINT('Ctrl Pts',(160.,4.30813900827813,692.462296651428));
#272733=CARTESIAN_POINT('Ctrl Pts',(160.339057893189,-8.28413408366083,
690.462296651428));
#272734=CARTESIAN_POINT('Ctrl Pts',(158.704075916301,-20.7744157382975,
688.462296651428));
#272735=CARTESIAN_POINT('Ctrl Pts',(157.069093939413,-33.2646973929343,
686.462296651429));
#272736=CARTESIAN_POINT('Ctrl Pts',(153.500330774912,-45.3454354230633,
684.462296651428));
#272737=CARTESIAN_POINT('Ctrl Pts',(149.931567610412,-57.4261734531924,
682.462296651428));
#272738=CARTESIAN_POINT('Ctrl Pts',(144.516898051455,-68.7998999948413,
680.462296651428));
#272739=CARTESIAN_POINT('Ctrl Pts',(139.102228492497,-80.1736265364901,
678.462296651428));
#272740=CARTESIAN_POINT('Ctrl Pts',(131.974979673883,-90.5602826949691,
676.462296651428));
#272741=CARTESIAN_POINT('Ctrl Pts',(124.847730855269,-100.946938853448,
674.462296651428));
#272742=CARTESIAN_POINT('Ctrl Pts',(116.183399296895,-110.0907706828,672.462296651428));
#272743=CARTESIAN_POINT('Ctrl Pts',(107.519067738521,-119.234602512152,
670.462296651428));
#272744=CARTESIAN_POINT('Ctrl Pts',(97.5309980386224,-126.9104585261,668.462296651428));
#272745=CARTESIAN_POINT('Ctrl Pts',(87.5429283387234,-134.586314540048,
666.462296651428));
#272746=CARTESIAN_POINT('Ctrl Pts',(76.4770599218137,-140.605189688823,
664.462296651428));
#272747=CARTESIAN_POINT('Ctrl Pts',(65.4111915049041,-146.624064837599,
662.462296651428));
#272748=CARTESIAN_POINT('Ctrl Pts',(53.5400027769198,-150.837754439537,
660.462296651428));
#272749=CARTESIAN_POINT('Ctrl Pts',(41.6688140489356,-155.051444041475,
658.462296651428));
#272750=CARTESIAN_POINT('Ctrl Pts',(29.2846130745764,-157.356193074143,
656.462296651428));
#272751=CARTESIAN_POINT('Ctrl Pts',(16.9004121002171,-159.660942106811,
654.462296651428));
#272752=CARTESIAN_POINT('Ctrl Pts',(4.30813900827814,-160.,652.462296651428));
#272753=CARTESIAN_POINT('Ctrl Pts',(-8.28413408366082,-160.339057893189,
650.462296651428));
#272754=CARTESIAN_POINT('Ctrl Pts',(-20.7744157382975,-158.704075916301,
648.462296651428));
#272755=CARTESIAN_POINT('Ctrl Pts',(-33.2646973929342,-157.069093939413,
646.462296651428));
#272756=CARTESIAN_POINT('Ctrl Pts',(-45.3454354230633,-153.500330774912,
644.462296651428));
#272757=CARTESIAN_POINT('Ctrl Pts',(-57.4261734531924,-149.931567610412,
642.462296651428));
#272758=CARTESIAN_POINT('Ctrl Pts',(-68.7998999948413,-144.516898051455,
640.462296651428));
#272759=CARTESIAN_POINT('Ctrl Pts',(-80.1736265364901,-139.102228492497,
638.462296651428));
#272760=CARTESIAN_POINT('Ctrl Pts',(-90.5602826949691,-131.974979673883,
636.462296651428));
#272761=CARTESIAN_POINT('Ctrl Pts',(-100.946938853448,-124.847730855269,
634.462296651428));
#272762=CARTESIAN_POINT('Ctrl Pts',(-110.0907706828,-116.183399296895,632.462296651428));
#272763=CARTESIAN_POINT('Ctrl Pts',(-119.234602512152,-107.519067738521,
630.462296651428));
#272764=CARTESIAN_POINT('Ctrl Pts',(-126.9104585261,-97.5309980386224,628.462296651428));
#272765=CARTESIAN_POINT('Ctrl Pts',(-134.586314540048,-87.5429283387234,
626.462296651429));
#272766=CARTESIAN_POINT('Ctrl Pts',(-140.605189688823,-76.4770599218137,
624.462296651428));
#272767=CARTESIAN_POINT('Ctrl Pts',(-146.624064837599,-65.4111915049041,
622.462296651428));
#272768=CARTESIAN_POINT('Ctrl Pts',(-150.837754439537,-53.5400027769199,
620.462296651428));
#272769=CARTESIAN_POINT('Ctrl Pts',(-155.051444041475,-41.6688140489356,
618.462296651428));
#272770=CARTESIAN_POINT('Ctrl Pts',(-157.356193074143,-29.2846130745764,
616.462296651428));
#272771=CARTESIAN_POINT('Ctrl Pts',(-159.660942106811,-16.9004121002171,
614.462296651429));
#272772=CARTESIAN_POINT('Ctrl Pts',(-160.,-4.30813900827815,612.462296651428));
#272773=CARTESIAN_POINT('Ctrl Pts',(-160.339057893189,8.28413408366081,
610.462296651428));
#272774=CARTESIAN_POINT('Ctrl Pts',(-158.704075916301,20.7744157382975,
608.462296651428));
#272775=CARTESIAN_POINT('Ctrl Pts',(-157.069093939413,33.2646973929342,
606.462296651428));
#272776=CARTESIAN_POINT('Ctrl Pts',(-153.500330774912,45.3454354230633,
604.462296651428));
#272777=CARTESIAN_POINT('Ctrl Pts',(-149.931567610412,57.4261734531924,
602.462296651429));
#272778=CARTESIAN_POINT('Ctrl Pts',(-144.516898051455,68.7998999948413,
600.462296651428));
#272779=CARTESIAN_POINT('Ctrl Pts',(-139.102228492497,80.1736265364901,
598.462296651428));
#272780=CARTESIAN_POINT('Ctrl Pts',(-131.974979673883,90.5602826949691,
596.462296651428));
#272781=CARTESIAN_POINT('Ctrl Pts',(-124.847730855269,100.946938853448,
594.462296651428));
#272782=CARTESIAN_POINT('Ctrl Pts',(-116.183399296895,110.0907706828,592.462296651428));
#272783=CARTESIAN_POINT('Ctrl Pts',(-107.519067738521,119.234602512152,
590.462296651428));
#272784=CARTESIAN_POINT('Ctrl Pts',(-97.5309980386224,126.9104585261,588.462296651428));
#272785=CARTESIAN_POINT('Ctrl Pts',(-87.5429283387233,134.586314540048,
586.462296651428));
#272786=CARTESIAN_POINT('Ctrl Pts',(-76.4770599218137,140.605189688823,
584.462296651428));
#272787=CARTESIAN_POINT('Ctrl Pts',(-65.4111915049042,146.624064837599,
582.462296651428));
#272788=CARTESIAN_POINT('Ctrl Pts',(-53.5400027769199,150.837754439537,
580.462296651428));
#272789=CARTESIAN_POINT('Ctrl Pts',(-41.6688140489356,155.051444041475,
578.462296651428));
#272790=CARTESIAN_POINT('Ctrl Pts',(-29.2846130745764,157.356193074143,
576.462296651428));
#272791=CARTESIAN_POINT('Ctrl Pts',(-16.9004121002172,159.660942106811,
574.462296651428));
#272792=CARTESIAN_POINT('Ctrl Pts',(-4.30813900827816,160.,572.462296651428));
#272793=CARTESIAN_POINT('Ctrl Pts',(8.28413408366087,160.339057893189,570.462296651428));
#272794=CARTESIAN_POINT('Ctrl Pts',(20.7744157382975,158.704075916301,568.462296651428));
#272795=CARTESIAN_POINT('Ctrl Pts',(33.2646973929342,157.069093939413,566.462296651428));
#272796=CARTESIAN_POINT('Ctrl Pts',(45.3454354230633,153.500330774912,564.462296651428));
#272797=CARTESIAN_POINT('Ctrl Pts',(57.4261734531925,149.931567610412,562.462296651428));
#272798=CARTESIAN_POINT('Ctrl Pts',(68.7998999948413,144.516898051455,560.462296651428));
#272799=CARTESIAN_POINT('Ctrl Pts',(80.1736265364901,139.102228492498,558.462296651428));
#272800=CARTESIAN_POINT('Ctrl Pts',(90.560282694969,131.974979673883,556.462296651428));
#272801=CARTESIAN_POINT('Ctrl Pts',(100.946938853448,124.847730855269,554.462296651428));
#272802=CARTESIAN_POINT('Ctrl Pts',(110.0907706828,116.183399296895,552.462296651428));
#272803=CARTESIAN_POINT('Ctrl Pts',(119.234602512152,107.519067738521,550.462296651428));
#272804=CARTESIAN_POINT('Ctrl Pts',(126.9104585261,97.5309980386224,548.462296651428));
#272805=CARTESIAN_POINT('Ctrl Pts',(134.586314540048,87.5429283387233,546.462296651428));
#272806=CARTESIAN_POINT('Ctrl Pts',(140.605189688823,76.4770599218137,544.462296651428));
#272807=CARTESIAN_POINT('Ctrl Pts',(146.624064837599,65.4111915049042,542.462296651428));
#272808=CARTESIAN_POINT('Ctrl Pts',(150.837754439537,53.5400027769199,540.462296651428));
#272809=CARTESIAN_POINT('Ctrl Pts',(155.051444041475,41.6688140489356,538.462296651428));
#272810=CARTESIAN_POINT('Ctrl Pts',(157.356193074143,29.2846130745764,536.462296651428));
#272811=CARTESIAN_POINT('Ctrl Pts',(159.660942106811,16.9004121002172,534.462296651428));
#272812=CARTESIAN_POINT('Ctrl Pts',(160.,4.30813900827813,532.462296651428));
#272813=CARTESIAN_POINT('Ctrl Pts',(160.,-4.30813900827805,697.537703348572));
#272814=CARTESIAN_POINT('Ctrl Pts',(159.660942106811,-16.900412100217,695.537703348572));
#272815=CARTESIAN_POINT('Ctrl Pts',(157.356193074143,-29.2846130745763,
693.537703348572));
#272816=CARTESIAN_POINT('Ctrl Pts',(155.051444041475,-41.6688140489355,
691.537703348572));
#272817=CARTESIAN_POINT('Ctrl Pts',(150.837754439537,-53.5400027769198,
689.537703348572));
#272818=CARTESIAN_POINT('Ctrl Pts',(146.624064837599,-65.411191504904,687.537703348572));
#272819=CARTESIAN_POINT('Ctrl Pts',(140.605189688823,-76.4770599218136,
685.537703348572));
#272820=CARTESIAN_POINT('Ctrl Pts',(134.586314540048,-87.5429283387233,
683.537703348572));
#272821=CARTESIAN_POINT('Ctrl Pts',(126.9104585261,-97.5309980386223,681.537703348572));
#272822=CARTESIAN_POINT('Ctrl Pts',(119.234602512152,-107.519067738521,
679.537703348572));
#272823=CARTESIAN_POINT('Ctrl Pts',(110.0907706828,-116.183399296895,677.537703348572));
#272824=CARTESIAN_POINT('Ctrl Pts',(100.946938853448,-124.847730855269,
675.537703348572));
#272825=CARTESIAN_POINT('Ctrl Pts',(90.5602826949691,-131.974979673883,
673.537703348572));
#272826=CARTESIAN_POINT('Ctrl Pts',(80.1736265364902,-139.102228492497,
671.537703348572));
#272827=CARTESIAN_POINT('Ctrl Pts',(68.7998999948414,-144.516898051454,
669.537703348572));
#272828=CARTESIAN_POINT('Ctrl Pts',(57.4261734531925,-149.931567610412,
667.537703348572));
#272829=CARTESIAN_POINT('Ctrl Pts',(45.3454354230634,-153.500330774912,
665.537703348572));
#272830=CARTESIAN_POINT('Ctrl Pts',(33.2646973929343,-157.069093939413,
663.537703348572));
#272831=CARTESIAN_POINT('Ctrl Pts',(20.7744157382976,-158.704075916301,
661.537703348572));
#272832=CARTESIAN_POINT('Ctrl Pts',(8.28413408366091,-160.339057893189,
659.537703348572));
#272833=CARTESIAN_POINT('Ctrl Pts',(-4.30813900827804,-160.,657.537703348572));
#272834=CARTESIAN_POINT('Ctrl Pts',(-16.900412100217,-159.660942106811,
655.537703348572));
#272835=CARTESIAN_POINT('Ctrl Pts',(-29.2846130745763,-157.356193074143,
653.537703348572));
#272836=CARTESIAN_POINT('Ctrl Pts',(-41.6688140489355,-155.051444041475,
651.537703348572));
#272837=CARTESIAN_POINT('Ctrl Pts',(-53.5400027769198,-150.837754439537,
649.537703348572));
#272838=CARTESIAN_POINT('Ctrl Pts',(-65.411191504904,-146.624064837599,
647.537703348572));
#272839=CARTESIAN_POINT('Ctrl Pts',(-76.4770599218136,-140.605189688823,
645.537703348572));
#272840=CARTESIAN_POINT('Ctrl Pts',(-87.5429283387233,-134.586314540048,
643.537703348572));
#272841=CARTESIAN_POINT('Ctrl Pts',(-97.5309980386223,-126.9104585261,641.537703348572));
#272842=CARTESIAN_POINT('Ctrl Pts',(-107.519067738521,-119.234602512152,
639.537703348572));
#272843=CARTESIAN_POINT('Ctrl Pts',(-116.183399296895,-110.0907706828,637.537703348572));
#272844=CARTESIAN_POINT('Ctrl Pts',(-124.847730855269,-100.946938853448,
635.537703348572));
#272845=CARTESIAN_POINT('Ctrl Pts',(-131.974979673883,-90.5602826949692,
633.537703348572));
#272846=CARTESIAN_POINT('Ctrl Pts',(-139.102228492497,-80.1736265364902,
631.537703348572));
#272847=CARTESIAN_POINT('Ctrl Pts',(-144.516898051454,-68.7998999948414,
629.537703348572));
#272848=CARTESIAN_POINT('Ctrl Pts',(-149.931567610412,-57.4261734531925,
627.537703348572));
#272849=CARTESIAN_POINT('Ctrl Pts',(-153.500330774912,-45.3454354230634,
625.537703348572));
#272850=CARTESIAN_POINT('Ctrl Pts',(-157.069093939413,-33.2646973929344,
623.537703348572));
#272851=CARTESIAN_POINT('Ctrl Pts',(-158.704075916301,-20.7744157382976,
621.537703348572));
#272852=CARTESIAN_POINT('Ctrl Pts',(-160.339057893189,-8.28413408366092,
619.537703348572));
#272853=CARTESIAN_POINT('Ctrl Pts',(-160.,4.30813900827803,617.537703348572));
#272854=CARTESIAN_POINT('Ctrl Pts',(-159.660942106811,16.900412100217,615.537703348572));
#272855=CARTESIAN_POINT('Ctrl Pts',(-157.356193074143,29.2846130745763,
613.537703348572));
#272856=CARTESIAN_POINT('Ctrl Pts',(-155.051444041475,41.6688140489355,
611.537703348572));
#272857=CARTESIAN_POINT('Ctrl Pts',(-150.837754439537,53.5400027769198,
609.537703348572));
#272858=CARTESIAN_POINT('Ctrl Pts',(-146.624064837599,65.411191504904,607.537703348572));
#272859=CARTESIAN_POINT('Ctrl Pts',(-140.605189688823,76.4770599218136,
605.537703348572));
#272860=CARTESIAN_POINT('Ctrl Pts',(-134.586314540048,87.5429283387233,
603.537703348572));
#272861=CARTESIAN_POINT('Ctrl Pts',(-126.9104585261,97.5309980386223,601.537703348572));
#272862=CARTESIAN_POINT('Ctrl Pts',(-119.234602512152,107.519067738521,
599.537703348572));
#272863=CARTESIAN_POINT('Ctrl Pts',(-110.0907706828,116.183399296895,597.537703348572));
#272864=CARTESIAN_POINT('Ctrl Pts',(-100.946938853448,124.847730855269,
595.537703348572));
#272865=CARTESIAN_POINT('Ctrl Pts',(-90.5602826949692,131.974979673883,
593.537703348572));
#272866=CARTESIAN_POINT('Ctrl Pts',(-80.1736265364901,139.102228492497,
591.537703348572));
#272867=CARTESIAN_POINT('Ctrl Pts',(-68.7998999948414,144.516898051454,
589.537703348572));
#272868=CARTESIAN_POINT('Ctrl Pts',(-57.4261734531926,149.931567610412,
587.537703348572));
#272869=CARTESIAN_POINT('Ctrl Pts',(-45.3454354230634,153.500330774912,
585.537703348572));
#272870=CARTESIAN_POINT('Ctrl Pts',(-33.2646973929343,157.069093939413,
583.537703348572));
#272871=CARTESIAN_POINT('Ctrl Pts',(-20.7744157382976,158.704075916301,
581.537703348572));
#272872=CARTESIAN_POINT('Ctrl Pts',(-8.284134083661,160.339057893189,579.537703348572));
#272873=CARTESIAN_POINT('Ctrl Pts',(4.30813900827803,160.,577.537703348572));
#272874=CARTESIAN_POINT('Ctrl Pts',(16.9004121002171,159.660942106811,575.537703348572));
#272875=CARTESIAN_POINT('Ctrl Pts',(29.2846130745762,157.356193074143,573.537703348572));
#272876=CARTESIAN_POINT('Ctrl Pts',(41.6688140489354,155.051444041476,571.537703348572));
#272877=CARTESIAN_POINT('Ctrl Pts',(53.5400027769198,150.837754439537,569.537703348572));
#272878=CARTESIAN_POINT('Ctrl Pts',(65.4111915049041,146.624064837599,567.537703348572));
#272879=CARTESIAN_POINT('Ctrl Pts',(76.4770599218136,140.605189688823,565.537703348572));
#272880=CARTESIAN_POINT('Ctrl Pts',(87.5429283387232,134.586314540048,563.537703348572));
#272881=CARTESIAN_POINT('Ctrl Pts',(97.5309980386223,126.9104585261,561.537703348572));
#272882=CARTESIAN_POINT('Ctrl Pts',(107.519067738521,119.234602512152,559.537703348572));
#272883=CARTESIAN_POINT('Ctrl Pts',(116.183399296895,110.0907706828,557.537703348572));
#272884=CARTESIAN_POINT('Ctrl Pts',(124.847730855269,100.946938853448,555.537703348572));
#272885=CARTESIAN_POINT('Ctrl Pts',(131.974979673883,90.5602826949692,553.537703348572));
#272886=CARTESIAN_POINT('Ctrl Pts',(139.102228492497,80.1736265364902,551.537703348572));
#272887=CARTESIAN_POINT('Ctrl Pts',(144.516898051454,68.7998999948414,549.537703348572));
#272888=CARTESIAN_POINT('Ctrl Pts',(149.931567610412,57.4261734531926,547.537703348572));
#272889=CARTESIAN_POINT('Ctrl Pts',(153.500330774912,45.3454354230634,545.537703348572));
#272890=CARTESIAN_POINT('Ctrl Pts',(157.069093939413,33.2646973929343,543.537703348572));
#272891=CARTESIAN_POINT('Ctrl Pts',(158.704075916301,20.7744157382976,541.537703348572));
#272892=CARTESIAN_POINT('Ctrl Pts',(160.339057893189,8.28413408366101,539.537703348572));
#272893=CARTESIAN_POINT('Ctrl Pts',(160.,-4.30813900827805,537.537703348572));
#272894=CARTESIAN_POINT('Origin',(-4.03737035479217,0.209103843994654,690.46237739249));
#272895=CARTESIAN_POINT('Ctrl Pts',(130.,4.30813900827812,692.462296651428));
#272896=CARTESIAN_POINT('Ctrl Pts',(130.339057893189,-5.92308287892228,
690.462296651428));
#272897=CARTESIAN_POINT('Ctrl Pts',(129.073425698447,-16.0813817870906,
688.462296651428));
#272898=CARTESIAN_POINT('Ctrl Pts',(127.807793503704,-26.2396806952589,
686.462296651429));
#272899=CARTESIAN_POINT('Ctrl Pts',(124.968635286058,-36.0749255918149,
684.462296651428));
#272900=CARTESIAN_POINT('Ctrl Pts',(122.129477068411,-45.9101704883709,
682.462296651428));
#272901=CARTESIAN_POINT('Ctrl Pts',(117.786702325803,-55.1801850026549,
680.462296651428));
#272902=CARTESIAN_POINT('Ctrl Pts',(113.443927583196,-64.4501995169389,
678.462296651428));
#272903=CARTESIAN_POINT('Ctrl Pts',(107.704469842635,-72.9267251261949,
676.462296651428));
#272904=CARTESIAN_POINT('Ctrl Pts',(101.965012102074,-81.4032507354509,
674.462296651428));
#272905=CARTESIAN_POINT('Ctrl Pts',(94.9701958612989,-88.8775672472035,
672.462296651428));
#272906=CARTESIAN_POINT('Ctrl Pts',(87.9753796205242,-96.351883758956,670.462296651428));
#272907=CARTESIAN_POINT('Ctrl Pts',(79.8974404698481,-102.639948694851,
668.462296651428));
#272908=CARTESIAN_POINT('Ctrl Pts',(71.8195013191721,-108.928013630747,
666.462296651428));
#272909=CARTESIAN_POINT('Ctrl Pts',(62.8573449296273,-113.874993963172,
664.462296651428));
#272910=CARTESIAN_POINT('Ctrl Pts',(53.8951885400825,-118.821974295598,
662.462296651428));
#272911=CARTESIAN_POINT('Ctrl Pts',(44.2694929456714,-122.306058950682,
660.462296651428));
#272912=CARTESIAN_POINT('Ctrl Pts',(34.6437973512603,-125.790143605767,
658.462296651428));
#272913=CARTESIAN_POINT('Ctrl Pts',(24.5915791233694,-127.725542856289,
656.462296651428));
#272914=CARTESIAN_POINT('Ctrl Pts',(14.5393608954785,-129.660942106811,
654.462296651428));
#272915=CARTESIAN_POINT('Ctrl Pts',(4.30813900827813,-130.,652.462296651428));
#272916=CARTESIAN_POINT('Ctrl Pts',(-5.92308287892227,-130.339057893189,
650.462296651428));
#272917=CARTESIAN_POINT('Ctrl Pts',(-16.0813817870906,-129.073425698447,
648.462296651428));
#272918=CARTESIAN_POINT('Ctrl Pts',(-26.2396806952589,-127.807793503705,
646.462296651428));
#272919=CARTESIAN_POINT('Ctrl Pts',(-36.0749255918149,-124.968635286058,
644.462296651428));
#272920=CARTESIAN_POINT('Ctrl Pts',(-45.9101704883709,-122.129477068411,
642.462296651428));
#272921=CARTESIAN_POINT('Ctrl Pts',(-55.1801850026549,-117.786702325803,
640.462296651428));
#272922=CARTESIAN_POINT('Ctrl Pts',(-64.4501995169389,-113.443927583196,
638.462296651428));
#272923=CARTESIAN_POINT('Ctrl Pts',(-72.9267251261949,-107.704469842635,
636.462296651428));
#272924=CARTESIAN_POINT('Ctrl Pts',(-81.4032507354509,-101.965012102074,
634.462296651428));
#272925=CARTESIAN_POINT('Ctrl Pts',(-88.8775672472034,-94.9701958612989,
632.462296651428));
#272926=CARTESIAN_POINT('Ctrl Pts',(-96.351883758956,-87.9753796205242,
630.462296651428));
#272927=CARTESIAN_POINT('Ctrl Pts',(-102.639948694851,-79.8974404698482,
628.462296651428));
#272928=CARTESIAN_POINT('Ctrl Pts',(-108.928013630747,-71.8195013191721,
626.462296651429));
#272929=CARTESIAN_POINT('Ctrl Pts',(-113.874993963172,-62.8573449296273,
624.462296651428));
#272930=CARTESIAN_POINT('Ctrl Pts',(-118.821974295598,-53.8951885400825,
622.462296651428));
#272931=CARTESIAN_POINT('Ctrl Pts',(-122.306058950682,-44.2694929456714,
620.462296651428));
#272932=CARTESIAN_POINT('Ctrl Pts',(-125.790143605767,-34.6437973512603,
618.462296651428));
#272933=CARTESIAN_POINT('Ctrl Pts',(-127.725542856289,-24.5915791233694,
616.462296651428));
#272934=CARTESIAN_POINT('Ctrl Pts',(-129.660942106811,-14.5393608954785,
614.462296651429));
#272935=CARTESIAN_POINT('Ctrl Pts',(-130.,-4.30813900827813,612.462296651428));
#272936=CARTESIAN_POINT('Ctrl Pts',(-130.339057893189,5.92308287892227,
610.462296651428));
#272937=CARTESIAN_POINT('Ctrl Pts',(-129.073425698447,16.0813817870906,
608.462296651428));
#272938=CARTESIAN_POINT('Ctrl Pts',(-127.807793503705,26.2396806952589,
606.462296651428));
#272939=CARTESIAN_POINT('Ctrl Pts',(-124.968635286058,36.0749255918149,
604.462296651428));
#272940=CARTESIAN_POINT('Ctrl Pts',(-122.129477068411,45.9101704883709,
602.462296651429));
#272941=CARTESIAN_POINT('Ctrl Pts',(-117.786702325803,55.1801850026549,
600.462296651428));
#272942=CARTESIAN_POINT('Ctrl Pts',(-113.443927583196,64.4501995169388,
598.462296651428));
#272943=CARTESIAN_POINT('Ctrl Pts',(-107.704469842635,72.9267251261949,
596.462296651428));
#272944=CARTESIAN_POINT('Ctrl Pts',(-101.965012102074,81.4032507354509,
594.462296651428));
#272945=CARTESIAN_POINT('Ctrl Pts',(-94.9701958612989,88.8775672472034,
592.462296651428));
#272946=CARTESIAN_POINT('Ctrl Pts',(-87.9753796205243,96.3518837589559,
590.462296651428));
#272947=CARTESIAN_POINT('Ctrl Pts',(-79.8974404698482,102.639948694851,
588.462296651428));
#272948=CARTESIAN_POINT('Ctrl Pts',(-71.819501319172,108.928013630747,586.462296651428));
#272949=CARTESIAN_POINT('Ctrl Pts',(-62.8573449296273,113.874993963172,
584.462296651428));
#272950=CARTESIAN_POINT('Ctrl Pts',(-53.8951885400826,118.821974295598,
582.462296651428));
#272951=CARTESIAN_POINT('Ctrl Pts',(-44.2694929456714,122.306058950682,
580.462296651428));
#272952=CARTESIAN_POINT('Ctrl Pts',(-34.6437973512603,125.790143605767,
578.462296651428));
#272953=CARTESIAN_POINT('Ctrl Pts',(-24.5915791233694,127.725542856289,
576.462296651428));
#272954=CARTESIAN_POINT('Ctrl Pts',(-14.5393608954786,129.660942106811,
574.462296651428));
#272955=CARTESIAN_POINT('Ctrl Pts',(-4.30813900827814,130.,572.462296651428));
#272956=CARTESIAN_POINT('Ctrl Pts',(5.92308287892232,130.339057893189,570.462296651428));
#272957=CARTESIAN_POINT('Ctrl Pts',(16.0813817870906,129.073425698447,568.462296651428));
#272958=CARTESIAN_POINT('Ctrl Pts',(26.2396806952589,127.807793503705,566.462296651428));
#272959=CARTESIAN_POINT('Ctrl Pts',(36.0749255918149,124.968635286058,564.462296651428));
#272960=CARTESIAN_POINT('Ctrl Pts',(45.9101704883709,122.129477068411,562.462296651428));
#272961=CARTESIAN_POINT('Ctrl Pts',(55.1801850026549,117.786702325803,560.462296651428));
#272962=CARTESIAN_POINT('Ctrl Pts',(64.4501995169388,113.443927583196,558.462296651428));
#272963=CARTESIAN_POINT('Ctrl Pts',(72.9267251261949,107.704469842635,556.462296651428));
#272964=CARTESIAN_POINT('Ctrl Pts',(81.4032507354509,101.965012102074,554.462296651428));
#272965=CARTESIAN_POINT('Ctrl Pts',(88.8775672472034,94.9701958612989,552.462296651428));
#272966=CARTESIAN_POINT('Ctrl Pts',(96.3518837589559,87.9753796205243,550.462296651428));
#272967=CARTESIAN_POINT('Ctrl Pts',(102.639948694851,79.8974404698482,548.462296651428));
#272968=CARTESIAN_POINT('Ctrl Pts',(108.928013630747,71.819501319172,546.462296651428));
#272969=CARTESIAN_POINT('Ctrl Pts',(113.874993963172,62.8573449296273,544.462296651428));
#272970=CARTESIAN_POINT('Ctrl Pts',(118.821974295598,53.8951885400826,542.462296651428));
#272971=CARTESIAN_POINT('Ctrl Pts',(122.306058950682,44.2694929456714,540.462296651428));
#272972=CARTESIAN_POINT('Ctrl Pts',(125.790143605767,34.6437973512603,538.462296651428));
#272973=CARTESIAN_POINT('Ctrl Pts',(127.725542856289,24.5915791233694,536.462296651428));
#272974=CARTESIAN_POINT('Ctrl Pts',(129.660942106811,14.5393608954786,534.462296651428));
#272975=CARTESIAN_POINT('Ctrl Pts',(130.,4.30813900827812,532.462296651428));
#272976=CARTESIAN_POINT('Ctrl Pts',(160.,4.30813900827813,692.462296651428));
#272977=CARTESIAN_POINT('Ctrl Pts',(160.339057893189,-8.28413408366083,
690.462296651428));
#272978=CARTESIAN_POINT('Ctrl Pts',(158.704075916301,-20.7744157382975,
688.462296651428));
#272979=CARTESIAN_POINT('Ctrl Pts',(157.069093939413,-33.2646973929343,
686.462296651429));
#272980=CARTESIAN_POINT('Ctrl Pts',(153.500330774912,-45.3454354230633,
684.462296651428));
#272981=CARTESIAN_POINT('Ctrl Pts',(149.931567610412,-57.4261734531924,
682.462296651428));
#272982=CARTESIAN_POINT('Ctrl Pts',(144.516898051455,-68.7998999948413,
680.462296651428));
#272983=CARTESIAN_POINT('Ctrl Pts',(139.102228492497,-80.1736265364901,
678.462296651428));
#272984=CARTESIAN_POINT('Ctrl Pts',(131.974979673883,-90.5602826949691,
676.462296651428));
#272985=CARTESIAN_POINT('Ctrl Pts',(124.847730855269,-100.946938853448,
674.462296651428));
#272986=CARTESIAN_POINT('Ctrl Pts',(116.183399296895,-110.0907706828,672.462296651428));
#272987=CARTESIAN_POINT('Ctrl Pts',(107.519067738521,-119.234602512152,
670.462296651428));
#272988=CARTESIAN_POINT('Ctrl Pts',(97.5309980386224,-126.9104585261,668.462296651428));
#272989=CARTESIAN_POINT('Ctrl Pts',(87.5429283387234,-134.586314540048,
666.462296651428));
#272990=CARTESIAN_POINT('Ctrl Pts',(76.4770599218137,-140.605189688823,
664.462296651428));
#272991=CARTESIAN_POINT('Ctrl Pts',(65.4111915049041,-146.624064837599,
662.462296651428));
#272992=CARTESIAN_POINT('Ctrl Pts',(53.5400027769198,-150.837754439537,
660.462296651428));
#272993=CARTESIAN_POINT('Ctrl Pts',(41.6688140489356,-155.051444041475,
658.462296651428));
#272994=CARTESIAN_POINT('Ctrl Pts',(29.2846130745764,-157.356193074143,
656.462296651428));
#272995=CARTESIAN_POINT('Ctrl Pts',(16.9004121002171,-159.660942106811,
654.462296651428));
#272996=CARTESIAN_POINT('Ctrl Pts',(4.30813900827814,-160.,652.462296651428));
#272997=CARTESIAN_POINT('Ctrl Pts',(-8.28413408366082,-160.339057893189,
650.462296651428));
#272998=CARTESIAN_POINT('Ctrl Pts',(-20.7744157382975,-158.704075916301,
648.462296651428));
#272999=CARTESIAN_POINT('Ctrl Pts',(-33.2646973929342,-157.069093939413,
646.462296651428));
#273000=CARTESIAN_POINT('Ctrl Pts',(-45.3454354230633,-153.500330774912,
644.462296651428));
#273001=CARTESIAN_POINT('Ctrl Pts',(-57.4261734531924,-149.931567610412,
642.462296651428));
#273002=CARTESIAN_POINT('Ctrl Pts',(-68.7998999948413,-144.516898051455,
640.462296651428));
#273003=CARTESIAN_POINT('Ctrl Pts',(-80.1736265364901,-139.102228492497,
638.462296651428));
#273004=CARTESIAN_POINT('Ctrl Pts',(-90.5602826949691,-131.974979673883,
636.462296651428));
#273005=CARTESIAN_POINT('Ctrl Pts',(-100.946938853448,-124.847730855269,
634.462296651428));
#273006=CARTESIAN_POINT('Ctrl Pts',(-110.0907706828,-116.183399296895,632.462296651428));
#273007=CARTESIAN_POINT('Ctrl Pts',(-119.234602512152,-107.519067738521,
630.462296651428));
#273008=CARTESIAN_POINT('Ctrl Pts',(-126.9104585261,-97.5309980386224,628.462296651428));
#273009=CARTESIAN_POINT('Ctrl Pts',(-134.586314540048,-87.5429283387234,
626.462296651429));
#273010=CARTESIAN_POINT('Ctrl Pts',(-140.605189688823,-76.4770599218137,
624.462296651428));
#273011=CARTESIAN_POINT('Ctrl Pts',(-146.624064837599,-65.4111915049041,
622.462296651428));
#273012=CARTESIAN_POINT('Ctrl Pts',(-150.837754439537,-53.5400027769199,
620.462296651428));
#273013=CARTESIAN_POINT('Ctrl Pts',(-155.051444041475,-41.6688140489356,
618.462296651428));
#273014=CARTESIAN_POINT('Ctrl Pts',(-157.356193074143,-29.2846130745764,
616.462296651428));
#273015=CARTESIAN_POINT('Ctrl Pts',(-159.660942106811,-16.9004121002171,
614.462296651429));
#273016=CARTESIAN_POINT('Ctrl Pts',(-160.,-4.30813900827815,612.462296651428));
#273017=CARTESIAN_POINT('Ctrl Pts',(-160.339057893189,8.28413408366081,
610.462296651428));
#273018=CARTESIAN_POINT('Ctrl Pts',(-158.704075916301,20.7744157382975,
608.462296651428));
#273019=CARTESIAN_POINT('Ctrl Pts',(-157.069093939413,33.2646973929342,
606.462296651428));
#273020=CARTESIAN_POINT('Ctrl Pts',(-153.500330774912,45.3454354230633,
604.462296651428));
#273021=CARTESIAN_POINT('Ctrl Pts',(-149.931567610412,57.4261734531924,
602.462296651429));
#273022=CARTESIAN_POINT('Ctrl Pts',(-144.516898051455,68.7998999948413,
600.462296651428));
#273023=CARTESIAN_POINT('Ctrl Pts',(-139.102228492497,80.1736265364901,
598.462296651428));
#273024=CARTESIAN_POINT('Ctrl Pts',(-131.974979673883,90.5602826949691,
596.462296651428));
#273025=CARTESIAN_POINT('Ctrl Pts',(-124.847730855269,100.946938853448,
594.462296651428));
#273026=CARTESIAN_POINT('Ctrl Pts',(-116.183399296895,110.0907706828,592.462296651428));
#273027=CARTESIAN_POINT('Ctrl Pts',(-107.519067738521,119.234602512152,
590.462296651428));
#273028=CARTESIAN_POINT('Ctrl Pts',(-97.5309980386224,126.9104585261,588.462296651428));
#273029=CARTESIAN_POINT('Ctrl Pts',(-87.5429283387233,134.586314540048,
586.462296651428));
#273030=CARTESIAN_POINT('Ctrl Pts',(-76.4770599218137,140.605189688823,
584.462296651428));
#273031=CARTESIAN_POINT('Ctrl Pts',(-65.4111915049042,146.624064837599,
582.462296651428));
#273032=CARTESIAN_POINT('Ctrl Pts',(-53.5400027769199,150.837754439537,
580.462296651428));
#273033=CARTESIAN_POINT('Ctrl Pts',(-41.6688140489356,155.051444041475,
578.462296651428));
#273034=CARTESIAN_POINT('Ctrl Pts',(-29.2846130745764,157.356193074143,
576.462296651428));
#273035=CARTESIAN_POINT('Ctrl Pts',(-16.9004121002172,159.660942106811,
574.462296651428));
#273036=CARTESIAN_POINT('Ctrl Pts',(-4.30813900827816,160.,572.462296651428));
#273037=CARTESIAN_POINT('Ctrl Pts',(8.28413408366087,160.339057893189,570.462296651428));
#273038=CARTESIAN_POINT('Ctrl Pts',(20.7744157382975,158.704075916301,568.462296651428));
#273039=CARTESIAN_POINT('Ctrl Pts',(33.2646973929342,157.069093939413,566.462296651428));
#273040=CARTESIAN_POINT('Ctrl Pts',(45.3454354230633,153.500330774912,564.462296651428));
#273041=CARTESIAN_POINT('Ctrl Pts',(57.4261734531925,149.931567610412,562.462296651428));
#273042=CARTESIAN_POINT('Ctrl Pts',(68.7998999948413,144.516898051455,560.462296651428));
#273043=CARTESIAN_POINT('Ctrl Pts',(80.1736265364901,139.102228492498,558.462296651428));
#273044=CARTESIAN_POINT('Ctrl Pts',(90.560282694969,131.974979673883,556.462296651428));
#273045=CARTESIAN_POINT('Ctrl Pts',(100.946938853448,124.847730855269,554.462296651428));
#273046=CARTESIAN_POINT('Ctrl Pts',(110.0907706828,116.183399296895,552.462296651428));
#273047=CARTESIAN_POINT('Ctrl Pts',(119.234602512152,107.519067738521,550.462296651428));
#273048=CARTESIAN_POINT('Ctrl Pts',(126.9104585261,97.5309980386224,548.462296651428));
#273049=CARTESIAN_POINT('Ctrl Pts',(134.586314540048,87.5429283387233,546.462296651428));
#273050=CARTESIAN_POINT('Ctrl Pts',(140.605189688823,76.4770599218137,544.462296651428));
#273051=CARTESIAN_POINT('Ctrl Pts',(146.624064837599,65.4111915049042,542.462296651428));
#273052=CARTESIAN_POINT('Ctrl Pts',(150.837754439537,53.5400027769199,540.462296651428));
#273053=CARTESIAN_POINT('Ctrl Pts',(155.051444041475,41.6688140489356,538.462296651428));
#273054=CARTESIAN_POINT('Ctrl Pts',(157.356193074143,29.2846130745764,536.462296651428));
#273055=CARTESIAN_POINT('Ctrl Pts',(159.660942106811,16.9004121002172,534.462296651428));
#273056=CARTESIAN_POINT('Ctrl Pts',(160.,4.30813900827813,532.462296651428));
#273057=CARTESIAN_POINT('Origin',(-160.,3.64291929955129E-14,375.));
#273058=CARTESIAN_POINT('',(-160.,1.3142072080973E-15,375.000000000001));
#273059=CARTESIAN_POINT('',(-160.,-4.30813900827827,378.90811221526));
#273060=CARTESIAN_POINT('Ctrl Pts',(-160.,-7.32747196252603E-14,375.000000000001));
#273061=CARTESIAN_POINT('Ctrl Pts',(-160.,-0.0199151703950658,375.01805734453));
#273062=CARTESIAN_POINT('Ctrl Pts',(-160.,-0.0398304324242802,375.036114587998));
#273063=CARTESIAN_POINT('Ctrl Pts',(-160.,-0.0597455111851762,375.05417203359));
#273064=CARTESIAN_POINT('Ctrl Pts',(-160.,-1.47617978719699,376.338484547725));
#273065=CARTESIAN_POINT('Ctrl Pts',(-160.,-2.89215276710122,377.623305748502));
#273066=CARTESIAN_POINT('Ctrl Pts',(-160.,-4.30813900827827,378.90811221526));
#273067=CARTESIAN_POINT('',(-160.,4.30813900827767,377.537703348572));
#273068=CARTESIAN_POINT('',(-160.,-4.21537804662364E-13,375.));
#273069=CARTESIAN_POINT('Ctrl Pts',(-160.,-4.30813900827827,378.90811221526));
#273070=CARTESIAN_POINT('Ctrl Pts',(-160.,-1.43604209806711,378.451335906458));
#273071=CARTESIAN_POINT('Ctrl Pts',(-160.,1.43594781992473,377.99388646458));
#273072=CARTESIAN_POINT('Ctrl Pts',(-160.,4.30813900827767,377.537703348572));
#273073=CARTESIAN_POINT('Ctrl Pts',(-160.,-4.30813900827851,532.462296651429));
#273074=CARTESIAN_POINT('Ctrl Pts',(-160.339057893189,8.28413408366045,
530.462296651429));
#273075=CARTESIAN_POINT('Ctrl Pts',(-158.704075916301,20.7744157382972,
528.462296651429));
#273076=CARTESIAN_POINT('Ctrl Pts',(-157.069093939413,33.2646973929339,
526.462296651429));
#273077=CARTESIAN_POINT('Ctrl Pts',(-153.500330774912,45.345435423063,524.462296651428));
#273078=CARTESIAN_POINT('Ctrl Pts',(-149.931567610412,57.4261734531921,
522.462296651429));
#273079=CARTESIAN_POINT('Ctrl Pts',(-144.516898051455,68.7998999948409,
520.462296651428));
#273080=CARTESIAN_POINT('Ctrl Pts',(-139.102228492498,80.1736265364898,
518.462296651428));
#273081=CARTESIAN_POINT('Ctrl Pts',(-131.974979673884,90.5602826949688,
516.462296651428));
#273082=CARTESIAN_POINT('Ctrl Pts',(-124.84773085527,100.946938853448,514.462296651429));
#273083=CARTESIAN_POINT('Ctrl Pts',(-116.183399296896,110.0907706828,512.462296651428));
#273084=CARTESIAN_POINT('Ctrl Pts',(-107.519067738522,119.234602512151,
510.462296651429));
#273085=CARTESIAN_POINT('Ctrl Pts',(-97.5309980386227,126.9104585261,508.462296651429));
#273086=CARTESIAN_POINT('Ctrl Pts',(-87.5429283387237,134.586314540048,
506.462296651428));
#273087=CARTESIAN_POINT('Ctrl Pts',(-76.4770599218141,140.605189688823,
504.462296651429));
#273088=CARTESIAN_POINT('Ctrl Pts',(-65.4111915049045,146.624064837598,
502.462296651429));
#273089=CARTESIAN_POINT('Ctrl Pts',(-53.5400027769202,150.837754439537,
500.462296651429));
#273090=CARTESIAN_POINT('Ctrl Pts',(-41.668814048936,155.051444041475,498.462296651429));
#273091=CARTESIAN_POINT('Ctrl Pts',(-29.2846130745767,157.356193074143,
496.462296651429));
#273092=CARTESIAN_POINT('Ctrl Pts',(-16.9004121002175,159.660942106811,
494.462296651429));
#273093=CARTESIAN_POINT('Ctrl Pts',(-4.30813900827852,160.,492.462296651428));
#273094=CARTESIAN_POINT('Ctrl Pts',(8.28413408366043,160.339057893189,490.462296651429));
#273095=CARTESIAN_POINT('Ctrl Pts',(20.7744157382972,158.704075916301,488.462296651429));
#273096=CARTESIAN_POINT('Ctrl Pts',(33.2646973929339,157.069093939413,486.462296651429));
#273097=CARTESIAN_POINT('Ctrl Pts',(45.345435423063,153.500330774912,484.462296651429));
#273098=CARTESIAN_POINT('Ctrl Pts',(57.4261734531921,149.931567610412,482.462296651429));
#273099=CARTESIAN_POINT('Ctrl Pts',(68.7998999948409,144.516898051455,480.462296651428));
#273100=CARTESIAN_POINT('Ctrl Pts',(80.1736265364898,139.102228492498,478.462296651429));
#273101=CARTESIAN_POINT('Ctrl Pts',(90.5602826949688,131.974979673884,476.462296651428));
#273102=CARTESIAN_POINT('Ctrl Pts',(100.946938853448,124.84773085527,474.462296651429));
#273103=CARTESIAN_POINT('Ctrl Pts',(110.0907706828,116.183399296896,472.462296651429));
#273104=CARTESIAN_POINT('Ctrl Pts',(119.234602512151,107.519067738522,470.462296651429));
#273105=CARTESIAN_POINT('Ctrl Pts',(126.9104585261,97.5309980386227,468.462296651429));
#273106=CARTESIAN_POINT('Ctrl Pts',(134.586314540048,87.5429283387237,466.462296651429));
#273107=CARTESIAN_POINT('Ctrl Pts',(140.605189688823,76.4770599218141,464.462296651429));
#273108=CARTESIAN_POINT('Ctrl Pts',(146.624064837598,65.4111915049045,462.462296651429));
#273109=CARTESIAN_POINT('Ctrl Pts',(150.837754439537,53.5400027769202,460.462296651429));
#273110=CARTESIAN_POINT('Ctrl Pts',(155.051444041475,41.668814048936,458.462296651429));
#273111=CARTESIAN_POINT('Ctrl Pts',(157.356193074143,29.2846130745767,456.462296651429));
#273112=CARTESIAN_POINT('Ctrl Pts',(159.660942106811,16.9004121002175,454.462296651429));
#273113=CARTESIAN_POINT('Ctrl Pts',(160.,4.30813900827853,452.462296651429));
#273114=CARTESIAN_POINT('Ctrl Pts',(160.339057893189,-8.28413408366043,
450.462296651429));
#273115=CARTESIAN_POINT('Ctrl Pts',(158.704075916301,-20.7744157382971,
448.462296651429));
#273116=CARTESIAN_POINT('Ctrl Pts',(157.069093939413,-33.2646973929339,
446.462296651429));
#273117=CARTESIAN_POINT('Ctrl Pts',(153.500330774912,-45.345435423063,444.462296651429));
#273118=CARTESIAN_POINT('Ctrl Pts',(149.931567610412,-57.4261734531921,
442.462296651429));
#273119=CARTESIAN_POINT('Ctrl Pts',(144.516898051455,-68.7998999948409,
440.462296651429));
#273120=CARTESIAN_POINT('Ctrl Pts',(139.102228492498,-80.1736265364898,
438.462296651429));
#273121=CARTESIAN_POINT('Ctrl Pts',(131.974979673884,-90.5602826949688,
436.462296651429));
#273122=CARTESIAN_POINT('Ctrl Pts',(124.84773085527,-100.946938853448,434.462296651429));
#273123=CARTESIAN_POINT('Ctrl Pts',(116.183399296896,-110.0907706828,432.462296651429));
#273124=CARTESIAN_POINT('Ctrl Pts',(107.519067738522,-119.234602512151,
430.462296651429));
#273125=CARTESIAN_POINT('Ctrl Pts',(97.5309980386227,-126.9104585261,428.462296651429));
#273126=CARTESIAN_POINT('Ctrl Pts',(87.5429283387236,-134.586314540048,
426.462296651429));
#273127=CARTESIAN_POINT('Ctrl Pts',(76.4770599218141,-140.605189688823,
424.462296651429));
#273128=CARTESIAN_POINT('Ctrl Pts',(65.4111915049046,-146.624064837598,
422.462296651429));
#273129=CARTESIAN_POINT('Ctrl Pts',(53.5400027769202,-150.837754439537,
420.462296651429));
#273130=CARTESIAN_POINT('Ctrl Pts',(41.6688140489359,-155.051444041475,
418.462296651429));
#273131=CARTESIAN_POINT('Ctrl Pts',(29.2846130745768,-157.356193074143,
416.462296651429));
#273132=CARTESIAN_POINT('Ctrl Pts',(16.9004121002176,-159.660942106811,
414.462296651429));
#273133=CARTESIAN_POINT('Ctrl Pts',(4.30813900827854,-160.,412.462296651429));
#273134=CARTESIAN_POINT('Ctrl Pts',(-8.28413408366049,-160.339057893189,
410.462296651429));
#273135=CARTESIAN_POINT('Ctrl Pts',(-20.7744157382971,-158.704075916301,
408.462296651429));
#273136=CARTESIAN_POINT('Ctrl Pts',(-33.2646973929338,-157.069093939413,
406.462296651429));
#273137=CARTESIAN_POINT('Ctrl Pts',(-45.345435423063,-153.500330774912,
404.462296651429));
#273138=CARTESIAN_POINT('Ctrl Pts',(-57.4261734531921,-149.931567610412,
402.462296651429));
#273139=CARTESIAN_POINT('Ctrl Pts',(-68.7998999948409,-144.516898051455,
400.462296651429));
#273140=CARTESIAN_POINT('Ctrl Pts',(-80.1736265364897,-139.102228492498,
398.462296651429));
#273141=CARTESIAN_POINT('Ctrl Pts',(-90.5602826949688,-131.974979673884,
396.462296651429));
#273142=CARTESIAN_POINT('Ctrl Pts',(-100.946938853448,-124.84773085527,
394.462296651429));
#273143=CARTESIAN_POINT('Ctrl Pts',(-110.0907706828,-116.183399296896,392.462296651429));
#273144=CARTESIAN_POINT('Ctrl Pts',(-119.234602512151,-107.519067738522,
390.462296651429));
#273145=CARTESIAN_POINT('Ctrl Pts',(-126.9104585261,-97.5309980386227,388.462296651429));
#273146=CARTESIAN_POINT('Ctrl Pts',(-134.586314540048,-87.5429283387236,
386.462296651429));
#273147=CARTESIAN_POINT('Ctrl Pts',(-140.605189688823,-76.4770599218141,
384.462296651429));
#273148=CARTESIAN_POINT('Ctrl Pts',(-146.624064837598,-65.4111915049046,
382.462296651429));
#273149=CARTESIAN_POINT('Ctrl Pts',(-150.837754439537,-53.5400027769203,
380.462296651429));
#273150=CARTESIAN_POINT('Ctrl Pts',(-155.051444041475,-41.668814048936,
378.462296651429));
#273151=CARTESIAN_POINT('Ctrl Pts',(-157.356193074143,-29.2846130745768,
376.462296651429));
#273152=CARTESIAN_POINT('Ctrl Pts',(-159.660942106811,-16.9004121002176,
374.462296651429));
#273153=CARTESIAN_POINT('Ctrl Pts',(-160.,-4.30813900827851,372.462296651429));
#273154=CARTESIAN_POINT('Ctrl Pts',(-160.,4.30813900827767,537.537703348572));
#273155=CARTESIAN_POINT('Ctrl Pts',(-159.660942106811,16.9004121002166,
535.537703348572));
#273156=CARTESIAN_POINT('Ctrl Pts',(-157.356193074143,29.2846130745759,
533.537703348572));
#273157=CARTESIAN_POINT('Ctrl Pts',(-155.051444041476,41.6688140489352,
531.537703348572));
#273158=CARTESIAN_POINT('Ctrl Pts',(-150.837754439537,53.5400027769194,
529.537703348572));
#273159=CARTESIAN_POINT('Ctrl Pts',(-146.624064837599,65.4111915049037,
527.537703348572));
#273160=CARTESIAN_POINT('Ctrl Pts',(-140.605189688823,76.4770599218133,
525.537703348572));
#273161=CARTESIAN_POINT('Ctrl Pts',(-134.586314540048,87.542928338723,523.537703348572));
#273162=CARTESIAN_POINT('Ctrl Pts',(-126.9104585261,97.530998038622,521.537703348572));
#273163=CARTESIAN_POINT('Ctrl Pts',(-119.234602512152,107.519067738521,
519.537703348572));
#273164=CARTESIAN_POINT('Ctrl Pts',(-110.0907706828,116.183399296895,517.537703348572));
#273165=CARTESIAN_POINT('Ctrl Pts',(-100.946938853448,124.847730855269,
515.537703348572));
#273166=CARTESIAN_POINT('Ctrl Pts',(-90.5602826949695,131.974979673883,
513.537703348572));
#273167=CARTESIAN_POINT('Ctrl Pts',(-80.1736265364906,139.102228492497,
511.537703348572));
#273168=CARTESIAN_POINT('Ctrl Pts',(-68.7998999948417,144.516898051454,
509.537703348572));
#273169=CARTESIAN_POINT('Ctrl Pts',(-57.4261734531929,149.931567610411,
507.537703348572));
#273170=CARTESIAN_POINT('Ctrl Pts',(-45.3454354230638,153.500330774912,
505.537703348572));
#273171=CARTESIAN_POINT('Ctrl Pts',(-33.2646973929347,157.069093939413,
503.537703348572));
#273172=CARTESIAN_POINT('Ctrl Pts',(-20.774415738298,158.704075916301,501.537703348572));
#273173=CARTESIAN_POINT('Ctrl Pts',(-8.28413408366129,160.339057893189,
499.537703348572));
#273174=CARTESIAN_POINT('Ctrl Pts',(4.30813900827766,160.,497.537703348572));
#273175=CARTESIAN_POINT('Ctrl Pts',(16.9004121002166,159.660942106811,495.537703348572));
#273176=CARTESIAN_POINT('Ctrl Pts',(29.2846130745759,157.356193074143,493.537703348572));
#273177=CARTESIAN_POINT('Ctrl Pts',(41.6688140489352,155.051444041476,491.537703348572));
#273178=CARTESIAN_POINT('Ctrl Pts',(53.5400027769194,150.837754439537,489.537703348572));
#273179=CARTESIAN_POINT('Ctrl Pts',(65.4111915049037,146.624064837599,487.537703348572));
#273180=CARTESIAN_POINT('Ctrl Pts',(76.4770599218133,140.605189688823,485.537703348572));
#273181=CARTESIAN_POINT('Ctrl Pts',(87.542928338723,134.586314540048,483.537703348572));
#273182=CARTESIAN_POINT('Ctrl Pts',(97.530998038622,126.9104585261,481.537703348572));
#273183=CARTESIAN_POINT('Ctrl Pts',(107.519067738521,119.234602512152,479.537703348572));
#273184=CARTESIAN_POINT('Ctrl Pts',(116.183399296895,110.0907706828,477.537703348572));
#273185=CARTESIAN_POINT('Ctrl Pts',(124.847730855269,100.946938853448,475.537703348572));
#273186=CARTESIAN_POINT('Ctrl Pts',(131.974979673883,90.5602826949695,473.537703348572));
#273187=CARTESIAN_POINT('Ctrl Pts',(139.102228492497,80.1736265364906,471.537703348572));
#273188=CARTESIAN_POINT('Ctrl Pts',(144.516898051454,68.7998999948417,469.537703348572));
#273189=CARTESIAN_POINT('Ctrl Pts',(149.931567610411,57.4261734531929,467.537703348572));
#273190=CARTESIAN_POINT('Ctrl Pts',(153.500330774912,45.3454354230638,465.537703348572));
#273191=CARTESIAN_POINT('Ctrl Pts',(157.069093939413,33.2646973929347,463.537703348572));
#273192=CARTESIAN_POINT('Ctrl Pts',(158.704075916301,20.774415738298,461.537703348572));
#273193=CARTESIAN_POINT('Ctrl Pts',(160.339057893189,8.28413408366131,459.537703348572));
#273194=CARTESIAN_POINT('Ctrl Pts',(160.,-4.30813900827765,457.537703348572));
#273195=CARTESIAN_POINT('Ctrl Pts',(159.660942106811,-16.9004121002166,
455.537703348572));
#273196=CARTESIAN_POINT('Ctrl Pts',(157.356193074143,-29.2846130745759,
453.537703348572));
#273197=CARTESIAN_POINT('Ctrl Pts',(155.051444041476,-41.6688140489352,
451.537703348572));
#273198=CARTESIAN_POINT('Ctrl Pts',(150.837754439537,-53.5400027769194,
449.537703348572));
#273199=CARTESIAN_POINT('Ctrl Pts',(146.624064837599,-65.4111915049036,
447.537703348572));
#273200=CARTESIAN_POINT('Ctrl Pts',(140.605189688823,-76.4770599218133,
445.537703348572));
#273201=CARTESIAN_POINT('Ctrl Pts',(134.586314540048,-87.5429283387229,
443.537703348572));
#273202=CARTESIAN_POINT('Ctrl Pts',(126.9104585261,-97.530998038622,441.537703348572));
#273203=CARTESIAN_POINT('Ctrl Pts',(119.234602512152,-107.519067738521,
439.537703348572));
#273204=CARTESIAN_POINT('Ctrl Pts',(110.0907706828,-116.183399296895,437.537703348572));
#273205=CARTESIAN_POINT('Ctrl Pts',(100.946938853448,-124.847730855269,
435.537703348572));
#273206=CARTESIAN_POINT('Ctrl Pts',(90.5602826949695,-131.974979673883,
433.537703348572));
#273207=CARTESIAN_POINT('Ctrl Pts',(80.1736265364905,-139.102228492497,
431.537703348572));
#273208=CARTESIAN_POINT('Ctrl Pts',(68.7998999948417,-144.516898051454,
429.537703348572));
#273209=CARTESIAN_POINT('Ctrl Pts',(57.426173453193,-149.931567610411,427.537703348572));
#273210=CARTESIAN_POINT('Ctrl Pts',(45.3454354230638,-153.500330774912,
425.537703348572));
#273211=CARTESIAN_POINT('Ctrl Pts',(33.2646973929347,-157.069093939413,
423.537703348572));
#273212=CARTESIAN_POINT('Ctrl Pts',(20.774415738298,-158.704075916301,421.537703348572));
#273213=CARTESIAN_POINT('Ctrl Pts',(8.28413408366139,-160.339057893189,
419.537703348572));
#273214=CARTESIAN_POINT('Ctrl Pts',(-4.30813900827764,-160.,417.537703348572));
#273215=CARTESIAN_POINT('Ctrl Pts',(-16.9004121002167,-159.660942106811,
415.537703348572));
#273216=CARTESIAN_POINT('Ctrl Pts',(-29.2846130745759,-157.356193074143,
413.537703348572));
#273217=CARTESIAN_POINT('Ctrl Pts',(-41.6688140489351,-155.051444041476,
411.537703348572));
#273218=CARTESIAN_POINT('Ctrl Pts',(-53.5400027769194,-150.837754439537,
409.537703348572));
#273219=CARTESIAN_POINT('Ctrl Pts',(-65.4111915049037,-146.624064837599,
407.537703348572));
#273220=CARTESIAN_POINT('Ctrl Pts',(-76.4770599218133,-140.605189688823,
405.537703348572));
#273221=CARTESIAN_POINT('Ctrl Pts',(-87.5429283387229,-134.586314540048,
403.537703348572));
#273222=CARTESIAN_POINT('Ctrl Pts',(-97.530998038622,-126.9104585261,401.537703348572));
#273223=CARTESIAN_POINT('Ctrl Pts',(-107.519067738521,-119.234602512152,
399.537703348572));
#273224=CARTESIAN_POINT('Ctrl Pts',(-116.183399296895,-110.0907706828,397.537703348572));
#273225=CARTESIAN_POINT('Ctrl Pts',(-124.847730855269,-100.946938853448,
395.537703348572));
#273226=CARTESIAN_POINT('Ctrl Pts',(-131.974979673883,-90.5602826949695,
393.537703348572));
#273227=CARTESIAN_POINT('Ctrl Pts',(-139.102228492497,-80.1736265364905,
391.537703348572));
#273228=CARTESIAN_POINT('Ctrl Pts',(-144.516898051454,-68.7998999948417,
389.537703348572));
#273229=CARTESIAN_POINT('Ctrl Pts',(-149.931567610411,-57.426173453193,
387.537703348572));
#273230=CARTESIAN_POINT('Ctrl Pts',(-153.500330774912,-45.3454354230638,
385.537703348572));
#273231=CARTESIAN_POINT('Ctrl Pts',(-157.069093939413,-33.2646973929347,
383.537703348572));
#273232=CARTESIAN_POINT('Ctrl Pts',(-158.704075916301,-20.774415738298,
381.537703348572));
#273233=CARTESIAN_POINT('Ctrl Pts',(-160.339057893189,-8.2841340836614,
379.537703348572));
#273234=CARTESIAN_POINT('Ctrl Pts',(-160.,4.30813900827767,377.537703348572));
#273235=CARTESIAN_POINT('Origin',(4.03737035481559,0.209103844003473,379.537622607612));
#273236=CARTESIAN_POINT('Ctrl Pts',(-160.,4.30813900827767,537.537703348572));
#273237=CARTESIAN_POINT('Ctrl Pts',(-159.660942106811,16.9004121002166,
535.537703348572));
#273238=CARTESIAN_POINT('Ctrl Pts',(-157.356193074143,29.2846130745759,
533.537703348572));
#273239=CARTESIAN_POINT('Ctrl Pts',(-155.051444041476,41.6688140489352,
531.537703348572));
#273240=CARTESIAN_POINT('Ctrl Pts',(-150.837754439537,53.5400027769194,
529.537703348572));
#273241=CARTESIAN_POINT('Ctrl Pts',(-146.624064837599,65.4111915049037,
527.537703348572));
#273242=CARTESIAN_POINT('Ctrl Pts',(-140.605189688823,76.4770599218133,
525.537703348572));
#273243=CARTESIAN_POINT('Ctrl Pts',(-134.586314540048,87.542928338723,523.537703348572));
#273244=CARTESIAN_POINT('Ctrl Pts',(-126.9104585261,97.530998038622,521.537703348572));
#273245=CARTESIAN_POINT('Ctrl Pts',(-119.234602512152,107.519067738521,
519.537703348572));
#273246=CARTESIAN_POINT('Ctrl Pts',(-110.0907706828,116.183399296895,517.537703348572));
#273247=CARTESIAN_POINT('Ctrl Pts',(-100.946938853448,124.847730855269,
515.537703348572));
#273248=CARTESIAN_POINT('Ctrl Pts',(-90.5602826949695,131.974979673883,
513.537703348572));
#273249=CARTESIAN_POINT('Ctrl Pts',(-80.1736265364906,139.102228492497,
511.537703348572));
#273250=CARTESIAN_POINT('Ctrl Pts',(-68.7998999948417,144.516898051454,
509.537703348572));
#273251=CARTESIAN_POINT('Ctrl Pts',(-57.4261734531929,149.931567610411,
507.537703348572));
#273252=CARTESIAN_POINT('Ctrl Pts',(-45.3454354230638,153.500330774912,
505.537703348572));
#273253=CARTESIAN_POINT('Ctrl Pts',(-33.2646973929347,157.069093939413,
503.537703348572));
#273254=CARTESIAN_POINT('Ctrl Pts',(-20.774415738298,158.704075916301,501.537703348572));
#273255=CARTESIAN_POINT('Ctrl Pts',(-8.28413408366129,160.339057893189,
499.537703348572));
#273256=CARTESIAN_POINT('Ctrl Pts',(4.30813900827766,160.,497.537703348572));
#273257=CARTESIAN_POINT('Ctrl Pts',(16.9004121002166,159.660942106811,495.537703348572));
#273258=CARTESIAN_POINT('Ctrl Pts',(29.2846130745759,157.356193074143,493.537703348572));
#273259=CARTESIAN_POINT('Ctrl Pts',(41.6688140489352,155.051444041476,491.537703348572));
#273260=CARTESIAN_POINT('Ctrl Pts',(53.5400027769194,150.837754439537,489.537703348572));
#273261=CARTESIAN_POINT('Ctrl Pts',(65.4111915049037,146.624064837599,487.537703348572));
#273262=CARTESIAN_POINT('Ctrl Pts',(76.4770599218133,140.605189688823,485.537703348572));
#273263=CARTESIAN_POINT('Ctrl Pts',(87.542928338723,134.586314540048,483.537703348572));
#273264=CARTESIAN_POINT('Ctrl Pts',(97.530998038622,126.9104585261,481.537703348572));
#273265=CARTESIAN_POINT('Ctrl Pts',(107.519067738521,119.234602512152,479.537703348572));
#273266=CARTESIAN_POINT('Ctrl Pts',(116.183399296895,110.0907706828,477.537703348572));
#273267=CARTESIAN_POINT('Ctrl Pts',(124.847730855269,100.946938853448,475.537703348572));
#273268=CARTESIAN_POINT('Ctrl Pts',(131.974979673883,90.5602826949695,473.537703348572));
#273269=CARTESIAN_POINT('Ctrl Pts',(139.102228492497,80.1736265364906,471.537703348572));
#273270=CARTESIAN_POINT('Ctrl Pts',(144.516898051454,68.7998999948417,469.537703348572));
#273271=CARTESIAN_POINT('Ctrl Pts',(149.931567610411,57.4261734531929,467.537703348572));
#273272=CARTESIAN_POINT('Ctrl Pts',(153.500330774912,45.3454354230638,465.537703348572));
#273273=CARTESIAN_POINT('Ctrl Pts',(157.069093939413,33.2646973929347,463.537703348572));
#273274=CARTESIAN_POINT('Ctrl Pts',(158.704075916301,20.774415738298,461.537703348572));
#273275=CARTESIAN_POINT('Ctrl Pts',(160.339057893189,8.28413408366131,459.537703348572));
#273276=CARTESIAN_POINT('Ctrl Pts',(160.,-4.30813900827765,457.537703348572));
#273277=CARTESIAN_POINT('Ctrl Pts',(159.660942106811,-16.9004121002166,
455.537703348572));
#273278=CARTESIAN_POINT('Ctrl Pts',(157.356193074143,-29.2846130745759,
453.537703348572));
#273279=CARTESIAN_POINT('Ctrl Pts',(155.051444041476,-41.6688140489352,
451.537703348572));
#273280=CARTESIAN_POINT('Ctrl Pts',(150.837754439537,-53.5400027769194,
449.537703348572));
#273281=CARTESIAN_POINT('Ctrl Pts',(146.624064837599,-65.4111915049036,
447.537703348572));
#273282=CARTESIAN_POINT('Ctrl Pts',(140.605189688823,-76.4770599218133,
445.537703348572));
#273283=CARTESIAN_POINT('Ctrl Pts',(134.586314540048,-87.5429283387229,
443.537703348572));
#273284=CARTESIAN_POINT('Ctrl Pts',(126.9104585261,-97.530998038622,441.537703348572));
#273285=CARTESIAN_POINT('Ctrl Pts',(119.234602512152,-107.519067738521,
439.537703348572));
#273286=CARTESIAN_POINT('Ctrl Pts',(110.0907706828,-116.183399296895,437.537703348572));
#273287=CARTESIAN_POINT('Ctrl Pts',(100.946938853448,-124.847730855269,
435.537703348572));
#273288=CARTESIAN_POINT('Ctrl Pts',(90.5602826949695,-131.974979673883,
433.537703348572));
#273289=CARTESIAN_POINT('Ctrl Pts',(80.1736265364905,-139.102228492497,
431.537703348572));
#273290=CARTESIAN_POINT('Ctrl Pts',(68.7998999948417,-144.516898051454,
429.537703348572));
#273291=CARTESIAN_POINT('Ctrl Pts',(57.426173453193,-149.931567610411,427.537703348572));
#273292=CARTESIAN_POINT('Ctrl Pts',(45.3454354230638,-153.500330774912,
425.537703348572));
#273293=CARTESIAN_POINT('Ctrl Pts',(33.2646973929347,-157.069093939413,
423.537703348572));
#273294=CARTESIAN_POINT('Ctrl Pts',(20.774415738298,-158.704075916301,421.537703348572));
#273295=CARTESIAN_POINT('Ctrl Pts',(8.28413408366139,-160.339057893189,
419.537703348572));
#273296=CARTESIAN_POINT('Ctrl Pts',(-4.30813900827764,-160.,417.537703348572));
#273297=CARTESIAN_POINT('Ctrl Pts',(-16.9004121002167,-159.660942106811,
415.537703348572));
#273298=CARTESIAN_POINT('Ctrl Pts',(-29.2846130745759,-157.356193074143,
413.537703348572));
#273299=CARTESIAN_POINT('Ctrl Pts',(-41.6688140489351,-155.051444041476,
411.537703348572));
#273300=CARTESIAN_POINT('Ctrl Pts',(-53.5400027769194,-150.837754439537,
409.537703348572));
#273301=CARTESIAN_POINT('Ctrl Pts',(-65.4111915049037,-146.624064837599,
407.537703348572));
#273302=CARTESIAN_POINT('Ctrl Pts',(-76.4770599218133,-140.605189688823,
405.537703348572));
#273303=CARTESIAN_POINT('Ctrl Pts',(-87.5429283387229,-134.586314540048,
403.537703348572));
#273304=CARTESIAN_POINT('Ctrl Pts',(-97.530998038622,-126.9104585261,401.537703348572));
#273305=CARTESIAN_POINT('Ctrl Pts',(-107.519067738521,-119.234602512152,
399.537703348572));
#273306=CARTESIAN_POINT('Ctrl Pts',(-116.183399296895,-110.0907706828,397.537703348572));
#273307=CARTESIAN_POINT('Ctrl Pts',(-124.847730855269,-100.946938853448,
395.537703348572));
#273308=CARTESIAN_POINT('Ctrl Pts',(-131.974979673883,-90.5602826949695,
393.537703348572));
#273309=CARTESIAN_POINT('Ctrl Pts',(-139.102228492497,-80.1736265364905,
391.537703348572));
#273310=CARTESIAN_POINT('Ctrl Pts',(-144.516898051454,-68.7998999948417,
389.537703348572));
#273311=CARTESIAN_POINT('Ctrl Pts',(-149.931567610411,-57.426173453193,
387.537703348572));
#273312=CARTESIAN_POINT('Ctrl Pts',(-153.500330774912,-45.3454354230638,
385.537703348572));
#273313=CARTESIAN_POINT('Ctrl Pts',(-157.069093939413,-33.2646973929347,
383.537703348572));
#273314=CARTESIAN_POINT('Ctrl Pts',(-158.704075916301,-20.774415738298,
381.537703348572));
#273315=CARTESIAN_POINT('Ctrl Pts',(-160.339057893189,-8.2841340836614,
379.537703348572));
#273316=CARTESIAN_POINT('Ctrl Pts',(-160.,4.30813900827767,377.537703348572));
#273317=CARTESIAN_POINT('Ctrl Pts',(-130.,4.30813900827773,537.537703348572));
#273318=CARTESIAN_POINT('Ctrl Pts',(-129.660942106811,14.5393608954781,
535.537703348572));
#273319=CARTESIAN_POINT('Ctrl Pts',(-127.725542856289,24.591579123369,533.537703348572));
#273320=CARTESIAN_POINT('Ctrl Pts',(-125.790143605767,34.6437973512599,
531.537703348572));
#273321=CARTESIAN_POINT('Ctrl Pts',(-122.306058950683,44.269492945671,529.537703348572));
#273322=CARTESIAN_POINT('Ctrl Pts',(-118.821974295598,53.8951885400822,
527.537703348572));
#273323=CARTESIAN_POINT('Ctrl Pts',(-113.874993963172,62.8573449296269,
525.537703348572));
#273324=CARTESIAN_POINT('Ctrl Pts',(-108.928013630747,71.8195013191717,
523.537703348572));
#273325=CARTESIAN_POINT('Ctrl Pts',(-102.639948694852,79.8974404698478,
521.537703348572));
#273326=CARTESIAN_POINT('Ctrl Pts',(-96.3518837589562,87.9753796205239,
519.537703348572));
#273327=CARTESIAN_POINT('Ctrl Pts',(-88.8775672472037,94.9701958612987,
517.537703348572));
#273328=CARTESIAN_POINT('Ctrl Pts',(-81.4032507354512,101.965012102073,
515.537703348572));
#273329=CARTESIAN_POINT('Ctrl Pts',(-72.9267251261952,107.704469842635,
513.537703348572));
#273330=CARTESIAN_POINT('Ctrl Pts',(-64.4501995169392,113.443927583196,
511.537703348572));
#273331=CARTESIAN_POINT('Ctrl Pts',(-55.1801850026552,117.786702325803,
509.537703348572));
#273332=CARTESIAN_POINT('Ctrl Pts',(-45.9101704883713,122.12947706841,507.537703348572));
#273333=CARTESIAN_POINT('Ctrl Pts',(-36.0749255918153,124.968635286057,
505.537703348572));
#273334=CARTESIAN_POINT('Ctrl Pts',(-26.2396806952593,127.807793503704,
503.537703348572));
#273335=CARTESIAN_POINT('Ctrl Pts',(-16.081381787091,129.073425698447,501.537703348572));
#273336=CARTESIAN_POINT('Ctrl Pts',(-5.92308287892268,130.339057893189,
499.537703348572));
#273337=CARTESIAN_POINT('Ctrl Pts',(4.30813900827772,130.,497.537703348572));
#273338=CARTESIAN_POINT('Ctrl Pts',(14.5393608954781,129.660942106811,495.537703348572));
#273339=CARTESIAN_POINT('Ctrl Pts',(24.591579123369,127.725542856289,493.537703348572));
#273340=CARTESIAN_POINT('Ctrl Pts',(34.6437973512599,125.790143605767,491.537703348572));
#273341=CARTESIAN_POINT('Ctrl Pts',(44.269492945671,122.306058950683,489.537703348572));
#273342=CARTESIAN_POINT('Ctrl Pts',(53.8951885400822,118.821974295598,487.537703348572));
#273343=CARTESIAN_POINT('Ctrl Pts',(62.8573449296269,113.874993963172,485.537703348572));
#273344=CARTESIAN_POINT('Ctrl Pts',(71.8195013191717,108.928013630747,483.537703348572));
#273345=CARTESIAN_POINT('Ctrl Pts',(79.8974404698478,102.639948694852,481.537703348572));
#273346=CARTESIAN_POINT('Ctrl Pts',(87.9753796205239,96.3518837589562,479.537703348572));
#273347=CARTESIAN_POINT('Ctrl Pts',(94.9701958612986,88.8775672472037,477.537703348572));
#273348=CARTESIAN_POINT('Ctrl Pts',(101.965012102073,81.4032507354512,475.537703348572));
#273349=CARTESIAN_POINT('Ctrl Pts',(107.704469842635,72.9267251261952,473.537703348572));
#273350=CARTESIAN_POINT('Ctrl Pts',(113.443927583196,64.4501995169392,471.537703348572));
#273351=CARTESIAN_POINT('Ctrl Pts',(117.786702325803,55.1801850026552,469.537703348572));
#273352=CARTESIAN_POINT('Ctrl Pts',(122.12947706841,45.9101704883713,467.537703348572));
#273353=CARTESIAN_POINT('Ctrl Pts',(124.968635286057,36.0749255918153,465.537703348572));
#273354=CARTESIAN_POINT('Ctrl Pts',(127.807793503704,26.2396806952593,463.537703348572));
#273355=CARTESIAN_POINT('Ctrl Pts',(129.073425698447,16.081381787091,461.537703348572));
#273356=CARTESIAN_POINT('Ctrl Pts',(130.339057893189,5.92308287892268,459.537703348572));
#273357=CARTESIAN_POINT('Ctrl Pts',(130.,-4.30813900827772,457.537703348572));
#273358=CARTESIAN_POINT('Ctrl Pts',(129.660942106811,-14.5393608954781,
455.537703348572));
#273359=CARTESIAN_POINT('Ctrl Pts',(127.725542856289,-24.591579123369,453.537703348572));
#273360=CARTESIAN_POINT('Ctrl Pts',(125.790143605767,-34.6437973512599,
451.537703348572));
#273361=CARTESIAN_POINT('Ctrl Pts',(122.306058950683,-44.269492945671,449.537703348572));
#273362=CARTESIAN_POINT('Ctrl Pts',(118.821974295598,-53.8951885400822,
447.537703348572));
#273363=CARTESIAN_POINT('Ctrl Pts',(113.874993963172,-62.8573449296269,
445.537703348572));
#273364=CARTESIAN_POINT('Ctrl Pts',(108.928013630747,-71.8195013191717,
443.537703348572));
#273365=CARTESIAN_POINT('Ctrl Pts',(102.639948694852,-79.8974404698478,
441.537703348572));
#273366=CARTESIAN_POINT('Ctrl Pts',(96.3518837589563,-87.9753796205239,
439.537703348572));
#273367=CARTESIAN_POINT('Ctrl Pts',(88.8775672472037,-94.9701958612986,
437.537703348572));
#273368=CARTESIAN_POINT('Ctrl Pts',(81.4032507354513,-101.965012102073,
435.537703348572));
#273369=CARTESIAN_POINT('Ctrl Pts',(72.9267251261952,-107.704469842635,
433.537703348572));
#273370=CARTESIAN_POINT('Ctrl Pts',(64.4501995169392,-113.443927583196,
431.537703348572));
#273371=CARTESIAN_POINT('Ctrl Pts',(55.1801850026552,-117.786702325803,
429.537703348572));
#273372=CARTESIAN_POINT('Ctrl Pts',(45.9101704883713,-122.12947706841,427.537703348572));
#273373=CARTESIAN_POINT('Ctrl Pts',(36.0749255918153,-124.968635286057,
425.537703348572));
#273374=CARTESIAN_POINT('Ctrl Pts',(26.2396806952593,-127.807793503704,
423.537703348572));
#273375=CARTESIAN_POINT('Ctrl Pts',(16.081381787091,-129.073425698447,421.537703348572));
#273376=CARTESIAN_POINT('Ctrl Pts',(5.92308287892275,-130.339057893189,
419.537703348572));
#273377=CARTESIAN_POINT('Ctrl Pts',(-4.30813900827771,-130.,417.537703348572));
#273378=CARTESIAN_POINT('Ctrl Pts',(-14.5393608954782,-129.660942106811,
415.537703348572));
#273379=CARTESIAN_POINT('Ctrl Pts',(-24.591579123369,-127.725542856289,
413.537703348572));
#273380=CARTESIAN_POINT('Ctrl Pts',(-34.6437973512598,-125.790143605767,
411.537703348572));
#273381=CARTESIAN_POINT('Ctrl Pts',(-44.269492945671,-122.306058950683,
409.537703348572));
#273382=CARTESIAN_POINT('Ctrl Pts',(-53.8951885400822,-118.821974295598,
407.537703348572));
#273383=CARTESIAN_POINT('Ctrl Pts',(-62.8573449296269,-113.874993963172,
405.537703348572));
#273384=CARTESIAN_POINT('Ctrl Pts',(-71.8195013191717,-108.928013630747,
403.537703348572));
#273385=CARTESIAN_POINT('Ctrl Pts',(-79.8974404698478,-102.639948694852,
401.537703348572));
#273386=CARTESIAN_POINT('Ctrl Pts',(-87.975379620524,-96.3518837589562,
399.537703348572));
#273387=CARTESIAN_POINT('Ctrl Pts',(-94.9701958612986,-88.8775672472037,
397.537703348572));
#273388=CARTESIAN_POINT('Ctrl Pts',(-101.965012102073,-81.4032507354513,
395.537703348572));
#273389=CARTESIAN_POINT('Ctrl Pts',(-107.704469842635,-72.9267251261952,
393.537703348572));
#273390=CARTESIAN_POINT('Ctrl Pts',(-113.443927583196,-64.4501995169392,
391.537703348572));
#273391=CARTESIAN_POINT('Ctrl Pts',(-117.786702325803,-55.1801850026553,
389.537703348572));
#273392=CARTESIAN_POINT('Ctrl Pts',(-122.12947706841,-45.9101704883713,
387.537703348572));
#273393=CARTESIAN_POINT('Ctrl Pts',(-124.968635286057,-36.0749255918153,
385.537703348572));
#273394=CARTESIAN_POINT('Ctrl Pts',(-127.807793503704,-26.2396806952593,
383.537703348572));
#273395=CARTESIAN_POINT('Ctrl Pts',(-129.073425698447,-16.081381787091,
381.537703348572));
#273396=CARTESIAN_POINT('Ctrl Pts',(-130.339057893189,-5.92308287892275,
379.537703348572));
#273397=CARTESIAN_POINT('Ctrl Pts',(-130.,4.30813900827773,377.537703348572));
#273398=CARTESIAN_POINT('Origin',(-160.,-1.08084483543429E-12,695.));
#273399=CARTESIAN_POINT('',(-160.,4.68174708145216E-13,695.000000000001));
#273400=CARTESIAN_POINT('',(-160.,4.3081390082779,691.09188778474));
#273401=CARTESIAN_POINT('Ctrl Pts',(-160.,4.68514116391816E-13,695.000000000001));
#273402=CARTESIAN_POINT('Ctrl Pts',(-160.,0.0199151703862232,694.981942655461));
#273403=CARTESIAN_POINT('Ctrl Pts',(-160.,0.0398304323877712,694.963885411962));
#273404=CARTESIAN_POINT('Ctrl Pts',(-160.,0.0597455111577332,694.945827966381));
#273405=CARTESIAN_POINT('Ctrl Pts',(-160.,1.47617978782475,693.661515452968));
#273406=CARTESIAN_POINT('Ctrl Pts',(-160.,2.89215276710192,692.376694251499));
#273407=CARTESIAN_POINT('Ctrl Pts',(-160.,4.30813900827806,691.091887784741));
#273408=CARTESIAN_POINT('',(-160.,-4.30813900827851,692.462296651429));
#273409=CARTESIAN_POINT('',(-160.,-4.21537804662364E-13,695.));
#273410=CARTESIAN_POINT('Ctrl Pts',(-160.,4.3081390082779,691.09188778474));
#273411=CARTESIAN_POINT('Ctrl Pts',(-160.,1.43604209808296,691.548664093541));
#273412=CARTESIAN_POINT('Ctrl Pts',(-160.,-1.43594781991723,692.006113535419));
#273413=CARTESIAN_POINT('Ctrl Pts',(-160.,-4.30813900827851,692.462296651429));
#273414=CARTESIAN_POINT('Ctrl Pts',(-130.,-4.30813900827845,692.462296651428));
#273415=CARTESIAN_POINT('Ctrl Pts',(-130.339057893189,5.92308287892195,
690.462296651428));
#273416=CARTESIAN_POINT('Ctrl Pts',(-129.073425698447,16.0813817870903,
688.462296651428));
#273417=CARTESIAN_POINT('Ctrl Pts',(-127.807793503705,26.2396806952586,
686.462296651429));
#273418=CARTESIAN_POINT('Ctrl Pts',(-124.968635286058,36.0749255918146,
684.462296651428));
#273419=CARTESIAN_POINT('Ctrl Pts',(-122.129477068411,45.9101704883706,
682.462296651429));
#273420=CARTESIAN_POINT('Ctrl Pts',(-117.786702325804,55.1801850026546,
680.462296651428));
#273421=CARTESIAN_POINT('Ctrl Pts',(-113.443927583196,64.4501995169386,
678.462296651428));
#273422=CARTESIAN_POINT('Ctrl Pts',(-107.704469842635,72.9267251261946,
676.462296651429));
#273423=CARTESIAN_POINT('Ctrl Pts',(-101.965012102074,81.4032507354507,
674.462296651429));
#273424=CARTESIAN_POINT('Ctrl Pts',(-94.9701958612992,88.8775672472032,
672.462296651428));
#273425=CARTESIAN_POINT('Ctrl Pts',(-87.9753796205245,96.3518837589558,
670.462296651429));
#273426=CARTESIAN_POINT('Ctrl Pts',(-79.8974404698484,102.639948694851,
668.462296651428));
#273427=CARTESIAN_POINT('Ctrl Pts',(-71.8195013191724,108.928013630747,
666.462296651428));
#273428=CARTESIAN_POINT('Ctrl Pts',(-62.8573449296276,113.874993963172,
664.462296651428));
#273429=CARTESIAN_POINT('Ctrl Pts',(-53.8951885400828,118.821974295598,
662.462296651429));
#273430=CARTESIAN_POINT('Ctrl Pts',(-44.2694929456717,122.306058950682,
660.462296651428));
#273431=CARTESIAN_POINT('Ctrl Pts',(-34.6437973512606,125.790143605767,
658.462296651428));
#273432=CARTESIAN_POINT('Ctrl Pts',(-24.5915791233697,127.725542856289,
656.462296651429));
#273433=CARTESIAN_POINT('Ctrl Pts',(-14.5393608954789,129.660942106811,
654.462296651428));
#273434=CARTESIAN_POINT('Ctrl Pts',(-4.30813900827846,130.,652.462296651428));
#273435=CARTESIAN_POINT('Ctrl Pts',(5.92308287892194,130.339057893189,650.462296651429));
#273436=CARTESIAN_POINT('Ctrl Pts',(16.0813817870903,129.073425698447,648.462296651428));
#273437=CARTESIAN_POINT('Ctrl Pts',(26.2396806952586,127.807793503705,646.462296651428));
#273438=CARTESIAN_POINT('Ctrl Pts',(36.0749255918146,124.968635286058,644.462296651428));
#273439=CARTESIAN_POINT('Ctrl Pts',(45.9101704883706,122.129477068411,642.462296651428));
#273440=CARTESIAN_POINT('Ctrl Pts',(55.1801850026546,117.786702325804,640.462296651428));
#273441=CARTESIAN_POINT('Ctrl Pts',(64.4501995169386,113.443927583196,638.462296651429));
#273442=CARTESIAN_POINT('Ctrl Pts',(72.9267251261946,107.704469842635,636.462296651428));
#273443=CARTESIAN_POINT('Ctrl Pts',(81.4032507354506,101.965012102074,634.462296651428));
#273444=CARTESIAN_POINT('Ctrl Pts',(88.8775672472032,94.9701958612992,632.462296651428));
#273445=CARTESIAN_POINT('Ctrl Pts',(96.3518837589558,87.9753796205245,630.462296651428));
#273446=CARTESIAN_POINT('Ctrl Pts',(102.639948694851,79.8974404698484,628.462296651428));
#273447=CARTESIAN_POINT('Ctrl Pts',(108.928013630747,71.8195013191724,626.462296651429));
#273448=CARTESIAN_POINT('Ctrl Pts',(113.874993963172,62.8573449296276,624.462296651428));
#273449=CARTESIAN_POINT('Ctrl Pts',(118.821974295598,53.8951885400829,622.462296651428));
#273450=CARTESIAN_POINT('Ctrl Pts',(122.306058950682,44.2694929456717,620.462296651428));
#273451=CARTESIAN_POINT('Ctrl Pts',(125.790143605767,34.6437973512606,618.462296651428));
#273452=CARTESIAN_POINT('Ctrl Pts',(127.725542856289,24.5915791233698,616.462296651428));
#273453=CARTESIAN_POINT('Ctrl Pts',(129.660942106811,14.5393608954789,614.462296651429));
#273454=CARTESIAN_POINT('Ctrl Pts',(130.,4.30813900827846,612.462296651428));
#273455=CARTESIAN_POINT('Ctrl Pts',(130.339057893189,-5.92308287892194,
610.462296651428));
#273456=CARTESIAN_POINT('Ctrl Pts',(129.073425698447,-16.0813817870903,
608.462296651428));
#273457=CARTESIAN_POINT('Ctrl Pts',(127.807793503705,-26.2396806952586,
606.462296651428));
#273458=CARTESIAN_POINT('Ctrl Pts',(124.968635286058,-36.0749255918146,
604.462296651428));
#273459=CARTESIAN_POINT('Ctrl Pts',(122.129477068411,-45.9101704883706,
602.462296651429));
#273460=CARTESIAN_POINT('Ctrl Pts',(117.786702325804,-55.1801850026546,
600.462296651428));
#273461=CARTESIAN_POINT('Ctrl Pts',(113.443927583196,-64.4501995169386,
598.462296651428));
#273462=CARTESIAN_POINT('Ctrl Pts',(107.704469842635,-72.9267251261946,
596.462296651428));
#273463=CARTESIAN_POINT('Ctrl Pts',(101.965012102074,-81.4032507354506,
594.462296651428));
#273464=CARTESIAN_POINT('Ctrl Pts',(94.9701958612992,-88.8775672472032,
592.462296651428));
#273465=CARTESIAN_POINT('Ctrl Pts',(87.9753796205246,-96.3518837589557,
590.462296651429));
#273466=CARTESIAN_POINT('Ctrl Pts',(79.8974404698484,-102.639948694851,
588.462296651428));
#273467=CARTESIAN_POINT('Ctrl Pts',(71.8195013191723,-108.928013630747,
586.462296651428));
#273468=CARTESIAN_POINT('Ctrl Pts',(62.8573449296276,-113.874993963172,
584.462296651428));
#273469=CARTESIAN_POINT('Ctrl Pts',(53.8951885400829,-118.821974295598,
582.462296651428));
#273470=CARTESIAN_POINT('Ctrl Pts',(44.2694929456717,-122.306058950682,
580.462296651428));
#273471=CARTESIAN_POINT('Ctrl Pts',(34.6437973512606,-125.790143605767,
578.462296651429));
#273472=CARTESIAN_POINT('Ctrl Pts',(24.5915791233698,-127.725542856289,
576.462296651428));
#273473=CARTESIAN_POINT('Ctrl Pts',(14.5393608954789,-129.660942106811,
574.462296651428));
#273474=CARTESIAN_POINT('Ctrl Pts',(4.30813900827847,-130.,572.462296651428));
#273475=CARTESIAN_POINT('Ctrl Pts',(-5.92308287892199,-130.339057893189,
570.462296651428));
#273476=CARTESIAN_POINT('Ctrl Pts',(-16.0813817870903,-129.073425698447,
568.462296651428));
#273477=CARTESIAN_POINT('Ctrl Pts',(-26.2396806952585,-127.807793503705,
566.462296651429));
#273478=CARTESIAN_POINT('Ctrl Pts',(-36.0749255918146,-124.968635286058,
564.462296651428));
#273479=CARTESIAN_POINT('Ctrl Pts',(-45.9101704883706,-122.129477068411,
562.462296651428));
#273480=CARTESIAN_POINT('Ctrl Pts',(-55.1801850026546,-117.786702325804,
560.462296651428));
#273481=CARTESIAN_POINT('Ctrl Pts',(-64.4501995169385,-113.443927583197,
558.462296651429));
#273482=CARTESIAN_POINT('Ctrl Pts',(-72.9267251261946,-107.704469842635,
556.462296651428));
#273483=CARTESIAN_POINT('Ctrl Pts',(-81.4032507354507,-101.965012102074,
554.462296651429));
#273484=CARTESIAN_POINT('Ctrl Pts',(-88.8775672472032,-94.9701958612992,
552.462296651428));
#273485=CARTESIAN_POINT('Ctrl Pts',(-96.3518837589557,-87.9753796205246,
550.462296651428));
#273486=CARTESIAN_POINT('Ctrl Pts',(-102.639948694851,-79.8974404698484,
548.462296651428));
#273487=CARTESIAN_POINT('Ctrl Pts',(-108.928013630747,-71.8195013191723,
546.462296651429));
#273488=CARTESIAN_POINT('Ctrl Pts',(-113.874993963172,-62.8573449296276,
544.462296651428));
#273489=CARTESIAN_POINT('Ctrl Pts',(-118.821974295598,-53.8951885400829,
542.462296651429));
#273490=CARTESIAN_POINT('Ctrl Pts',(-122.306058950682,-44.2694929456718,
540.462296651428));
#273491=CARTESIAN_POINT('Ctrl Pts',(-125.790143605767,-34.6437973512606,
538.462296651428));
#273492=CARTESIAN_POINT('Ctrl Pts',(-127.725542856289,-24.5915791233698,
536.462296651428));
#273493=CARTESIAN_POINT('Ctrl Pts',(-129.660942106811,-14.5393608954789,
534.462296651429));
#273494=CARTESIAN_POINT('Ctrl Pts',(-130.,-4.30813900827845,532.462296651428));
#273495=CARTESIAN_POINT('Ctrl Pts',(-160.,-4.30813900827851,692.462296651429));
#273496=CARTESIAN_POINT('Ctrl Pts',(-160.339057893189,8.28413408366045,
690.462296651429));
#273497=CARTESIAN_POINT('Ctrl Pts',(-158.704075916301,20.7744157382972,
688.462296651429));
#273498=CARTESIAN_POINT('Ctrl Pts',(-157.069093939413,33.2646973929339,
686.462296651429));
#273499=CARTESIAN_POINT('Ctrl Pts',(-153.500330774912,45.345435423063,684.462296651429));
#273500=CARTESIAN_POINT('Ctrl Pts',(-149.931567610412,57.4261734531921,
682.462296651429));
#273501=CARTESIAN_POINT('Ctrl Pts',(-144.516898051455,68.7998999948409,
680.462296651429));
#273502=CARTESIAN_POINT('Ctrl Pts',(-139.102228492498,80.1736265364898,
678.462296651429));
#273503=CARTESIAN_POINT('Ctrl Pts',(-131.974979673884,90.5602826949688,
676.462296651429));
#273504=CARTESIAN_POINT('Ctrl Pts',(-124.84773085527,100.946938853448,674.462296651429));
#273505=CARTESIAN_POINT('Ctrl Pts',(-116.183399296896,110.0907706828,672.462296651429));
#273506=CARTESIAN_POINT('Ctrl Pts',(-107.519067738522,119.234602512151,
670.462296651429));
#273507=CARTESIAN_POINT('Ctrl Pts',(-97.5309980386227,126.9104585261,668.462296651429));
#273508=CARTESIAN_POINT('Ctrl Pts',(-87.5429283387237,134.586314540048,
666.462296651429));
#273509=CARTESIAN_POINT('Ctrl Pts',(-76.4770599218141,140.605189688823,
664.462296651429));
#273510=CARTESIAN_POINT('Ctrl Pts',(-65.4111915049045,146.624064837598,
662.462296651429));
#273511=CARTESIAN_POINT('Ctrl Pts',(-53.5400027769202,150.837754439537,
660.462296651429));
#273512=CARTESIAN_POINT('Ctrl Pts',(-41.668814048936,155.051444041475,658.462296651429));
#273513=CARTESIAN_POINT('Ctrl Pts',(-29.2846130745767,157.356193074143,
656.462296651429));
#273514=CARTESIAN_POINT('Ctrl Pts',(-16.9004121002175,159.660942106811,
654.462296651428));
#273515=CARTESIAN_POINT('Ctrl Pts',(-4.30813900827852,160.,652.462296651429));
#273516=CARTESIAN_POINT('Ctrl Pts',(8.28413408366043,160.339057893189,650.462296651429));
#273517=CARTESIAN_POINT('Ctrl Pts',(20.7744157382972,158.704075916301,648.462296651428));
#273518=CARTESIAN_POINT('Ctrl Pts',(33.2646973929339,157.069093939413,646.462296651429));
#273519=CARTESIAN_POINT('Ctrl Pts',(45.345435423063,153.500330774912,644.462296651428));
#273520=CARTESIAN_POINT('Ctrl Pts',(57.4261734531921,149.931567610412,642.462296651428));
#273521=CARTESIAN_POINT('Ctrl Pts',(68.7998999948409,144.516898051455,640.462296651428));
#273522=CARTESIAN_POINT('Ctrl Pts',(80.1736265364898,139.102228492498,638.462296651429));
#273523=CARTESIAN_POINT('Ctrl Pts',(90.5602826949688,131.974979673884,636.462296651428));
#273524=CARTESIAN_POINT('Ctrl Pts',(100.946938853448,124.84773085527,634.462296651428));
#273525=CARTESIAN_POINT('Ctrl Pts',(110.0907706828,116.183399296896,632.462296651429));
#273526=CARTESIAN_POINT('Ctrl Pts',(119.234602512151,107.519067738522,630.462296651429));
#273527=CARTESIAN_POINT('Ctrl Pts',(126.9104585261,97.5309980386227,628.462296651429));
#273528=CARTESIAN_POINT('Ctrl Pts',(134.586314540048,87.5429283387237,626.462296651429));
#273529=CARTESIAN_POINT('Ctrl Pts',(140.605189688823,76.4770599218141,624.462296651429));
#273530=CARTESIAN_POINT('Ctrl Pts',(146.624064837598,65.4111915049045,622.462296651429));
#273531=CARTESIAN_POINT('Ctrl Pts',(150.837754439537,53.5400027769202,620.462296651429));
#273532=CARTESIAN_POINT('Ctrl Pts',(155.051444041475,41.668814048936,618.462296651429));
#273533=CARTESIAN_POINT('Ctrl Pts',(157.356193074143,29.2846130745767,616.462296651429));
#273534=CARTESIAN_POINT('Ctrl Pts',(159.660942106811,16.9004121002175,614.462296651429));
#273535=CARTESIAN_POINT('Ctrl Pts',(160.,4.30813900827853,612.462296651429));
#273536=CARTESIAN_POINT('Ctrl Pts',(160.339057893189,-8.28413408366043,
610.462296651429));
#273537=CARTESIAN_POINT('Ctrl Pts',(158.704075916301,-20.7744157382971,
608.462296651429));
#273538=CARTESIAN_POINT('Ctrl Pts',(157.069093939413,-33.2646973929339,
606.462296651429));
#273539=CARTESIAN_POINT('Ctrl Pts',(153.500330774912,-45.345435423063,604.462296651429));
#273540=CARTESIAN_POINT('Ctrl Pts',(149.931567610412,-57.4261734531921,
602.462296651429));
#273541=CARTESIAN_POINT('Ctrl Pts',(144.516898051455,-68.7998999948409,
600.462296651429));
#273542=CARTESIAN_POINT('Ctrl Pts',(139.102228492498,-80.1736265364898,
598.462296651429));
#273543=CARTESIAN_POINT('Ctrl Pts',(131.974979673884,-90.5602826949688,
596.462296651429));
#273544=CARTESIAN_POINT('Ctrl Pts',(124.84773085527,-100.946938853448,594.462296651428));
#273545=CARTESIAN_POINT('Ctrl Pts',(116.183399296896,-110.0907706828,592.462296651429));
#273546=CARTESIAN_POINT('Ctrl Pts',(107.519067738522,-119.234602512151,
590.462296651429));
#273547=CARTESIAN_POINT('Ctrl Pts',(97.5309980386227,-126.9104585261,588.462296651429));
#273548=CARTESIAN_POINT('Ctrl Pts',(87.5429283387236,-134.586314540048,
586.462296651429));
#273549=CARTESIAN_POINT('Ctrl Pts',(76.4770599218141,-140.605189688823,
584.462296651429));
#273550=CARTESIAN_POINT('Ctrl Pts',(65.4111915049046,-146.624064837598,
582.462296651428));
#273551=CARTESIAN_POINT('Ctrl Pts',(53.5400027769202,-150.837754439537,
580.462296651429));
#273552=CARTESIAN_POINT('Ctrl Pts',(41.6688140489359,-155.051444041475,
578.462296651429));
#273553=CARTESIAN_POINT('Ctrl Pts',(29.2846130745768,-157.356193074143,
576.462296651429));
#273554=CARTESIAN_POINT('Ctrl Pts',(16.9004121002176,-159.660942106811,
574.462296651429));
#273555=CARTESIAN_POINT('Ctrl Pts',(4.30813900827854,-160.,572.462296651429));
#273556=CARTESIAN_POINT('Ctrl Pts',(-8.28413408366049,-160.339057893189,
570.462296651428));
#273557=CARTESIAN_POINT('Ctrl Pts',(-20.7744157382971,-158.704075916301,
568.462296651429));
#273558=CARTESIAN_POINT('Ctrl Pts',(-33.2646973929338,-157.069093939413,
566.462296651429));
#273559=CARTESIAN_POINT('Ctrl Pts',(-45.345435423063,-153.500330774912,
564.462296651429));
#273560=CARTESIAN_POINT('Ctrl Pts',(-57.4261734531921,-149.931567610412,
562.462296651429));
#273561=CARTESIAN_POINT('Ctrl Pts',(-68.7998999948409,-144.516898051455,
560.462296651429));
#273562=CARTESIAN_POINT('Ctrl Pts',(-80.1736265364897,-139.102228492498,
558.462296651429));
#273563=CARTESIAN_POINT('Ctrl Pts',(-90.5602826949688,-131.974979673884,
556.462296651429));
#273564=CARTESIAN_POINT('Ctrl Pts',(-100.946938853448,-124.84773085527,
554.462296651429));
#273565=CARTESIAN_POINT('Ctrl Pts',(-110.0907706828,-116.183399296896,552.462296651429));
#273566=CARTESIAN_POINT('Ctrl Pts',(-119.234602512151,-107.519067738522,
550.462296651429));
#273567=CARTESIAN_POINT('Ctrl Pts',(-126.9104585261,-97.5309980386227,548.462296651429));
#273568=CARTESIAN_POINT('Ctrl Pts',(-134.586314540048,-87.5429283387236,
546.462296651429));
#273569=CARTESIAN_POINT('Ctrl Pts',(-140.605189688823,-76.4770599218141,
544.462296651429));
#273570=CARTESIAN_POINT('Ctrl Pts',(-146.624064837598,-65.4111915049046,
542.462296651429));
#273571=CARTESIAN_POINT('Ctrl Pts',(-150.837754439537,-53.5400027769203,
540.462296651429));
#273572=CARTESIAN_POINT('Ctrl Pts',(-155.051444041475,-41.668814048936,
538.462296651429));
#273573=CARTESIAN_POINT('Ctrl Pts',(-157.356193074143,-29.2846130745768,
536.462296651429));
#273574=CARTESIAN_POINT('Ctrl Pts',(-159.660942106811,-16.9004121002176,
534.462296651429));
#273575=CARTESIAN_POINT('Ctrl Pts',(-160.,-4.30813900827851,532.462296651429));
#273576=CARTESIAN_POINT('Origin',(4.03737035478159,-0.209103844020683,690.462377392296));
#273577=CARTESIAN_POINT('Ctrl Pts',(-160.,-4.30813900827851,692.462296651429));
#273578=CARTESIAN_POINT('Ctrl Pts',(-160.339057893189,8.28413408366045,
690.462296651429));
#273579=CARTESIAN_POINT('Ctrl Pts',(-158.704075916301,20.7744157382972,
688.462296651429));
#273580=CARTESIAN_POINT('Ctrl Pts',(-157.069093939413,33.2646973929339,
686.462296651429));
#273581=CARTESIAN_POINT('Ctrl Pts',(-153.500330774912,45.345435423063,684.462296651429));
#273582=CARTESIAN_POINT('Ctrl Pts',(-149.931567610412,57.4261734531921,
682.462296651429));
#273583=CARTESIAN_POINT('Ctrl Pts',(-144.516898051455,68.7998999948409,
680.462296651429));
#273584=CARTESIAN_POINT('Ctrl Pts',(-139.102228492498,80.1736265364898,
678.462296651429));
#273585=CARTESIAN_POINT('Ctrl Pts',(-131.974979673884,90.5602826949688,
676.462296651429));
#273586=CARTESIAN_POINT('Ctrl Pts',(-124.84773085527,100.946938853448,674.462296651429));
#273587=CARTESIAN_POINT('Ctrl Pts',(-116.183399296896,110.0907706828,672.462296651429));
#273588=CARTESIAN_POINT('Ctrl Pts',(-107.519067738522,119.234602512151,
670.462296651429));
#273589=CARTESIAN_POINT('Ctrl Pts',(-97.5309980386227,126.9104585261,668.462296651429));
#273590=CARTESIAN_POINT('Ctrl Pts',(-87.5429283387237,134.586314540048,
666.462296651429));
#273591=CARTESIAN_POINT('Ctrl Pts',(-76.4770599218141,140.605189688823,
664.462296651429));
#273592=CARTESIAN_POINT('Ctrl Pts',(-65.4111915049045,146.624064837598,
662.462296651429));
#273593=CARTESIAN_POINT('Ctrl Pts',(-53.5400027769202,150.837754439537,
660.462296651429));
#273594=CARTESIAN_POINT('Ctrl Pts',(-41.668814048936,155.051444041475,658.462296651429));
#273595=CARTESIAN_POINT('Ctrl Pts',(-29.2846130745767,157.356193074143,
656.462296651429));
#273596=CARTESIAN_POINT('Ctrl Pts',(-16.9004121002175,159.660942106811,
654.462296651428));
#273597=CARTESIAN_POINT('Ctrl Pts',(-4.30813900827852,160.,652.462296651429));
#273598=CARTESIAN_POINT('Ctrl Pts',(8.28413408366043,160.339057893189,650.462296651429));
#273599=CARTESIAN_POINT('Ctrl Pts',(20.7744157382972,158.704075916301,648.462296651428));
#273600=CARTESIAN_POINT('Ctrl Pts',(33.2646973929339,157.069093939413,646.462296651429));
#273601=CARTESIAN_POINT('Ctrl Pts',(45.345435423063,153.500330774912,644.462296651428));
#273602=CARTESIAN_POINT('Ctrl Pts',(57.4261734531921,149.931567610412,642.462296651428));
#273603=CARTESIAN_POINT('Ctrl Pts',(68.7998999948409,144.516898051455,640.462296651428));
#273604=CARTESIAN_POINT('Ctrl Pts',(80.1736265364898,139.102228492498,638.462296651429));
#273605=CARTESIAN_POINT('Ctrl Pts',(90.5602826949688,131.974979673884,636.462296651428));
#273606=CARTESIAN_POINT('Ctrl Pts',(100.946938853448,124.84773085527,634.462296651428));
#273607=CARTESIAN_POINT('Ctrl Pts',(110.0907706828,116.183399296896,632.462296651429));
#273608=CARTESIAN_POINT('Ctrl Pts',(119.234602512151,107.519067738522,630.462296651429));
#273609=CARTESIAN_POINT('Ctrl Pts',(126.9104585261,97.5309980386227,628.462296651429));
#273610=CARTESIAN_POINT('Ctrl Pts',(134.586314540048,87.5429283387237,626.462296651429));
#273611=CARTESIAN_POINT('Ctrl Pts',(140.605189688823,76.4770599218141,624.462296651429));
#273612=CARTESIAN_POINT('Ctrl Pts',(146.624064837598,65.4111915049045,622.462296651429));
#273613=CARTESIAN_POINT('Ctrl Pts',(150.837754439537,53.5400027769202,620.462296651429));
#273614=CARTESIAN_POINT('Ctrl Pts',(155.051444041475,41.668814048936,618.462296651429));
#273615=CARTESIAN_POINT('Ctrl Pts',(157.356193074143,29.2846130745767,616.462296651429));
#273616=CARTESIAN_POINT('Ctrl Pts',(159.660942106811,16.9004121002175,614.462296651429));
#273617=CARTESIAN_POINT('Ctrl Pts',(160.,4.30813900827853,612.462296651429));
#273618=CARTESIAN_POINT('Ctrl Pts',(160.339057893189,-8.28413408366043,
610.462296651429));
#273619=CARTESIAN_POINT('Ctrl Pts',(158.704075916301,-20.7744157382971,
608.462296651429));
#273620=CARTESIAN_POINT('Ctrl Pts',(157.069093939413,-33.2646973929339,
606.462296651429));
#273621=CARTESIAN_POINT('Ctrl Pts',(153.500330774912,-45.345435423063,604.462296651429));
#273622=CARTESIAN_POINT('Ctrl Pts',(149.931567610412,-57.4261734531921,
602.462296651429));
#273623=CARTESIAN_POINT('Ctrl Pts',(144.516898051455,-68.7998999948409,
600.462296651429));
#273624=CARTESIAN_POINT('Ctrl Pts',(139.102228492498,-80.1736265364898,
598.462296651429));
#273625=CARTESIAN_POINT('Ctrl Pts',(131.974979673884,-90.5602826949688,
596.462296651429));
#273626=CARTESIAN_POINT('Ctrl Pts',(124.84773085527,-100.946938853448,594.462296651428));
#273627=CARTESIAN_POINT('Ctrl Pts',(116.183399296896,-110.0907706828,592.462296651429));
#273628=CARTESIAN_POINT('Ctrl Pts',(107.519067738522,-119.234602512151,
590.462296651429));
#273629=CARTESIAN_POINT('Ctrl Pts',(97.5309980386227,-126.9104585261,588.462296651429));
#273630=CARTESIAN_POINT('Ctrl Pts',(87.5429283387236,-134.586314540048,
586.462296651429));
#273631=CARTESIAN_POINT('Ctrl Pts',(76.4770599218141,-140.605189688823,
584.462296651429));
#273632=CARTESIAN_POINT('Ctrl Pts',(65.4111915049046,-146.624064837598,
582.462296651428));
#273633=CARTESIAN_POINT('Ctrl Pts',(53.5400027769202,-150.837754439537,
580.462296651429));
#273634=CARTESIAN_POINT('Ctrl Pts',(41.6688140489359,-155.051444041475,
578.462296651429));
#273635=CARTESIAN_POINT('Ctrl Pts',(29.2846130745768,-157.356193074143,
576.462296651429));
#273636=CARTESIAN_POINT('Ctrl Pts',(16.9004121002176,-159.660942106811,
574.462296651429));
#273637=CARTESIAN_POINT('Ctrl Pts',(4.30813900827854,-160.,572.462296651429));
#273638=CARTESIAN_POINT('Ctrl Pts',(-8.28413408366049,-160.339057893189,
570.462296651428));
#273639=CARTESIAN_POINT('Ctrl Pts',(-20.7744157382971,-158.704075916301,
568.462296651429));
#273640=CARTESIAN_POINT('Ctrl Pts',(-33.2646973929338,-157.069093939413,
566.462296651429));
#273641=CARTESIAN_POINT('Ctrl Pts',(-45.345435423063,-153.500330774912,
564.462296651429));
#273642=CARTESIAN_POINT('Ctrl Pts',(-57.4261734531921,-149.931567610412,
562.462296651429));
#273643=CARTESIAN_POINT('Ctrl Pts',(-68.7998999948409,-144.516898051455,
560.462296651429));
#273644=CARTESIAN_POINT('Ctrl Pts',(-80.1736265364897,-139.102228492498,
558.462296651429));
#273645=CARTESIAN_POINT('Ctrl Pts',(-90.5602826949688,-131.974979673884,
556.462296651429));
#273646=CARTESIAN_POINT('Ctrl Pts',(-100.946938853448,-124.84773085527,
554.462296651429));
#273647=CARTESIAN_POINT('Ctrl Pts',(-110.0907706828,-116.183399296896,552.462296651429));
#273648=CARTESIAN_POINT('Ctrl Pts',(-119.234602512151,-107.519067738522,
550.462296651429));
#273649=CARTESIAN_POINT('Ctrl Pts',(-126.9104585261,-97.5309980386227,548.462296651429));
#273650=CARTESIAN_POINT('Ctrl Pts',(-134.586314540048,-87.5429283387236,
546.462296651429));
#273651=CARTESIAN_POINT('Ctrl Pts',(-140.605189688823,-76.4770599218141,
544.462296651429));
#273652=CARTESIAN_POINT('Ctrl Pts',(-146.624064837598,-65.4111915049046,
542.462296651429));
#273653=CARTESIAN_POINT('Ctrl Pts',(-150.837754439537,-53.5400027769203,
540.462296651429));
#273654=CARTESIAN_POINT('Ctrl Pts',(-155.051444041475,-41.668814048936,
538.462296651429));
#273655=CARTESIAN_POINT('Ctrl Pts',(-157.356193074143,-29.2846130745768,
536.462296651429));
#273656=CARTESIAN_POINT('Ctrl Pts',(-159.660942106811,-16.9004121002176,
534.462296651429));
#273657=CARTESIAN_POINT('Ctrl Pts',(-160.,-4.30813900827851,532.462296651429));
#273658=CARTESIAN_POINT('Ctrl Pts',(-160.,4.30813900827767,697.537703348572));
#273659=CARTESIAN_POINT('Ctrl Pts',(-159.660942106811,16.9004121002166,
695.537703348572));
#273660=CARTESIAN_POINT('Ctrl Pts',(-157.356193074143,29.2846130745759,
693.537703348572));
#273661=CARTESIAN_POINT('Ctrl Pts',(-155.051444041476,41.6688140489352,
691.537703348572));
#273662=CARTESIAN_POINT('Ctrl Pts',(-150.837754439537,53.5400027769194,
689.537703348572));
#273663=CARTESIAN_POINT('Ctrl Pts',(-146.624064837599,65.4111915049037,
687.537703348572));
#273664=CARTESIAN_POINT('Ctrl Pts',(-140.605189688823,76.4770599218133,
685.537703348572));
#273665=CARTESIAN_POINT('Ctrl Pts',(-134.586314540048,87.542928338723,683.537703348572));
#273666=CARTESIAN_POINT('Ctrl Pts',(-126.9104585261,97.530998038622,681.537703348572));
#273667=CARTESIAN_POINT('Ctrl Pts',(-119.234602512152,107.519067738521,
679.537703348572));
#273668=CARTESIAN_POINT('Ctrl Pts',(-110.0907706828,116.183399296895,677.537703348572));
#273669=CARTESIAN_POINT('Ctrl Pts',(-100.946938853448,124.847730855269,
675.537703348572));
#273670=CARTESIAN_POINT('Ctrl Pts',(-90.5602826949695,131.974979673883,
673.537703348572));
#273671=CARTESIAN_POINT('Ctrl Pts',(-80.1736265364906,139.102228492497,
671.537703348572));
#273672=CARTESIAN_POINT('Ctrl Pts',(-68.7998999948417,144.516898051454,
669.537703348572));
#273673=CARTESIAN_POINT('Ctrl Pts',(-57.4261734531929,149.931567610411,
667.537703348572));
#273674=CARTESIAN_POINT('Ctrl Pts',(-45.3454354230638,153.500330774912,
665.537703348572));
#273675=CARTESIAN_POINT('Ctrl Pts',(-33.2646973929347,157.069093939413,
663.537703348572));
#273676=CARTESIAN_POINT('Ctrl Pts',(-20.774415738298,158.704075916301,661.537703348572));
#273677=CARTESIAN_POINT('Ctrl Pts',(-8.28413408366129,160.339057893189,
659.537703348572));
#273678=CARTESIAN_POINT('Ctrl Pts',(4.30813900827766,160.,657.537703348572));
#273679=CARTESIAN_POINT('Ctrl Pts',(16.9004121002166,159.660942106811,655.537703348572));
#273680=CARTESIAN_POINT('Ctrl Pts',(29.2846130745759,157.356193074143,653.537703348572));
#273681=CARTESIAN_POINT('Ctrl Pts',(41.6688140489352,155.051444041476,651.537703348572));
#273682=CARTESIAN_POINT('Ctrl Pts',(53.5400027769194,150.837754439537,649.537703348572));
#273683=CARTESIAN_POINT('Ctrl Pts',(65.4111915049037,146.624064837599,647.537703348572));
#273684=CARTESIAN_POINT('Ctrl Pts',(76.4770599218133,140.605189688823,645.537703348572));
#273685=CARTESIAN_POINT('Ctrl Pts',(87.542928338723,134.586314540048,643.537703348572));
#273686=CARTESIAN_POINT('Ctrl Pts',(97.530998038622,126.9104585261,641.537703348572));
#273687=CARTESIAN_POINT('Ctrl Pts',(107.519067738521,119.234602512152,639.537703348572));
#273688=CARTESIAN_POINT('Ctrl Pts',(116.183399296895,110.0907706828,637.537703348572));
#273689=CARTESIAN_POINT('Ctrl Pts',(124.847730855269,100.946938853448,635.537703348572));
#273690=CARTESIAN_POINT('Ctrl Pts',(131.974979673883,90.5602826949695,633.537703348572));
#273691=CARTESIAN_POINT('Ctrl Pts',(139.102228492497,80.1736265364906,631.537703348572));
#273692=CARTESIAN_POINT('Ctrl Pts',(144.516898051454,68.7998999948417,629.537703348572));
#273693=CARTESIAN_POINT('Ctrl Pts',(149.931567610411,57.4261734531929,627.537703348572));
#273694=CARTESIAN_POINT('Ctrl Pts',(153.500330774912,45.3454354230638,625.537703348572));
#273695=CARTESIAN_POINT('Ctrl Pts',(157.069093939413,33.2646973929347,623.537703348572));
#273696=CARTESIAN_POINT('Ctrl Pts',(158.704075916301,20.774415738298,621.537703348572));
#273697=CARTESIAN_POINT('Ctrl Pts',(160.339057893189,8.28413408366131,619.537703348572));
#273698=CARTESIAN_POINT('Ctrl Pts',(160.,-4.30813900827765,617.537703348572));
#273699=CARTESIAN_POINT('Ctrl Pts',(159.660942106811,-16.9004121002166,
615.537703348572));
#273700=CARTESIAN_POINT('Ctrl Pts',(157.356193074143,-29.2846130745759,
613.537703348572));
#273701=CARTESIAN_POINT('Ctrl Pts',(155.051444041476,-41.6688140489352,
611.537703348572));
#273702=CARTESIAN_POINT('Ctrl Pts',(150.837754439537,-53.5400027769194,
609.537703348572));
#273703=CARTESIAN_POINT('Ctrl Pts',(146.624064837599,-65.4111915049036,
607.537703348572));
#273704=CARTESIAN_POINT('Ctrl Pts',(140.605189688823,-76.4770599218133,
605.537703348572));
#273705=CARTESIAN_POINT('Ctrl Pts',(134.586314540048,-87.5429283387229,
603.537703348572));
#273706=CARTESIAN_POINT('Ctrl Pts',(126.9104585261,-97.530998038622,601.537703348572));
#273707=CARTESIAN_POINT('Ctrl Pts',(119.234602512152,-107.519067738521,
599.537703348572));
#273708=CARTESIAN_POINT('Ctrl Pts',(110.0907706828,-116.183399296895,597.537703348572));
#273709=CARTESIAN_POINT('Ctrl Pts',(100.946938853448,-124.847730855269,
595.537703348572));
#273710=CARTESIAN_POINT('Ctrl Pts',(90.5602826949695,-131.974979673883,
593.537703348572));
#273711=CARTESIAN_POINT('Ctrl Pts',(80.1736265364905,-139.102228492497,
591.537703348572));
#273712=CARTESIAN_POINT('Ctrl Pts',(68.7998999948417,-144.516898051454,
589.537703348572));
#273713=CARTESIAN_POINT('Ctrl Pts',(57.426173453193,-149.931567610411,587.537703348572));
#273714=CARTESIAN_POINT('Ctrl Pts',(45.3454354230638,-153.500330774912,
585.537703348572));
#273715=CARTESIAN_POINT('Ctrl Pts',(33.2646973929347,-157.069093939413,
583.537703348572));
#273716=CARTESIAN_POINT('Ctrl Pts',(20.774415738298,-158.704075916301,581.537703348572));
#273717=CARTESIAN_POINT('Ctrl Pts',(8.28413408366139,-160.339057893189,
579.537703348572));
#273718=CARTESIAN_POINT('Ctrl Pts',(-4.30813900827764,-160.,577.537703348572));
#273719=CARTESIAN_POINT('Ctrl Pts',(-16.9004121002167,-159.660942106811,
575.537703348572));
#273720=CARTESIAN_POINT('Ctrl Pts',(-29.2846130745759,-157.356193074143,
573.537703348572));
#273721=CARTESIAN_POINT('Ctrl Pts',(-41.6688140489351,-155.051444041476,
571.537703348572));
#273722=CARTESIAN_POINT('Ctrl Pts',(-53.5400027769194,-150.837754439537,
569.537703348572));
#273723=CARTESIAN_POINT('Ctrl Pts',(-65.4111915049037,-146.624064837599,
567.537703348572));
#273724=CARTESIAN_POINT('Ctrl Pts',(-76.4770599218133,-140.605189688823,
565.537703348572));
#273725=CARTESIAN_POINT('Ctrl Pts',(-87.5429283387229,-134.586314540048,
563.537703348572));
#273726=CARTESIAN_POINT('Ctrl Pts',(-97.530998038622,-126.9104585261,561.537703348572));
#273727=CARTESIAN_POINT('Ctrl Pts',(-107.519067738521,-119.234602512152,
559.537703348572));
#273728=CARTESIAN_POINT('Ctrl Pts',(-116.183399296895,-110.0907706828,557.537703348572));
#273729=CARTESIAN_POINT('Ctrl Pts',(-124.847730855269,-100.946938853448,
555.537703348572));
#273730=CARTESIAN_POINT('Ctrl Pts',(-131.974979673883,-90.5602826949695,
553.537703348572));
#273731=CARTESIAN_POINT('Ctrl Pts',(-139.102228492497,-80.1736265364905,
551.537703348572));
#273732=CARTESIAN_POINT('Ctrl Pts',(-144.516898051454,-68.7998999948417,
549.537703348572));
#273733=CARTESIAN_POINT('Ctrl Pts',(-149.931567610411,-57.426173453193,
547.537703348572));
#273734=CARTESIAN_POINT('Ctrl Pts',(-153.500330774912,-45.3454354230638,
545.537703348572));
#273735=CARTESIAN_POINT('Ctrl Pts',(-157.069093939413,-33.2646973929347,
543.537703348572));
#273736=CARTESIAN_POINT('Ctrl Pts',(-158.704075916301,-20.774415738298,
541.537703348572));
#273737=CARTESIAN_POINT('Ctrl Pts',(-160.339057893189,-8.2841340836614,
539.537703348572));
#273738=CARTESIAN_POINT('Ctrl Pts',(-160.,4.30813900827767,537.537703348572));
#273739=CARTESIAN_POINT('Origin',(-160.339057893189,22.4999999999891,848.));
#273740=CARTESIAN_POINT('Origin',(-160.,-160.339057893189,367.5));
#276451=UNCERTAINTY_MEASURE_WITH_UNIT(LENGTH_MEASURE(0.01),#276463,
'DISTANCE_ACCURACY_VALUE',
'Maximum model space distance between geometric entities at asserted c
onnectivities');
#276454=UNCERTAINTY_MEASURE_WITH_UNIT(LENGTH_MEASURE(0.01),#276463,
'DISTANCE_ACCURACY_VALUE',
'Maximum model space distance between geometric entities at asserted c
onnectivities');
#276459=(
GEOMETRIC_REPRESENTATION_CONTEXT(3)
GLOBAL_UNCERTAINTY_ASSIGNED_CONTEXT((#276451))
GLOBAL_UNIT_ASSIGNED_CONTEXT((#276463,#276465,#276466))
REPRESENTATION_CONTEXT('','3D')
);
#276462=(
GEOMETRIC_REPRESENTATION_CONTEXT(3)
GLOBAL_UNCERTAINTY_ASSIGNED_CONTEXT((#276454))
GLOBAL_UNIT_ASSIGNED_CONTEXT((#276463,#276465,#276466))
REPRESENTATION_CONTEXT('','3D')
);
#276463=(
LENGTH_UNIT()
NAMED_UNIT(*)
SI_UNIT(.MILLI.,.METRE.)
);
#276465=(
NAMED_UNIT(*)
PLANE_ANGLE_UNIT()
SI_UNIT($,.RADIAN.)
);
#276466=(
NAMED_UNIT(*)
SI_UNIT($,.STERADIAN.)
SOLID_ANGLE_UNIT()
);
#276471=SHAPE_DEFINITION_REPRESENTATION(#276478,#276491);
#276478=PRODUCT_DEFINITION_SHAPE('',$,#276499);
#276491=SHAPE_REPRESENTATION('',(#110834),#276459);
#276494=PRODUCT_DEFINITION_CONTEXT('part definition',#276517,'design');
#276499=PRODUCT_DEFINITION('Agitator Blade Assembly',
'Agitator Blade Assembly',#276506,#276494);
#276506=PRODUCT_DEFINITION_FORMATION('',$,#276523);
#276517=APPLICATION_CONTEXT(
'Core Data for Automotive Mechanical Design Process');
#276518=PRODUCT_CONTEXT('part definition',#276517,'mechanical');
#276523=PRODUCT('Agitator Blade Assembly','Agitator Blade Assembly',$,(#276518));
#276530=PRESENTATION_STYLE_ASSIGNMENT((#276535));
#276535=SURFACE_STYLE_USAGE(.BOTH.,#276540);
#276540=SURFACE_SIDE_STYLE('',(#276545));
#276545=SURFACE_STYLE_FILL_AREA(#276550);
#276550=FILL_AREA_STYLE('Opaque(227,224,212)',(#276555));
#276555=FILL_AREA_STYLE_COLOUR('Opaque(227,224,212)',#276560);
#276560=COLOUR_RGB('Opaque(227,224,212)',0.890196078431372,0.87843137254902,
0.831372549019608);
ENDSEC;
END-ISO-10303-21;
